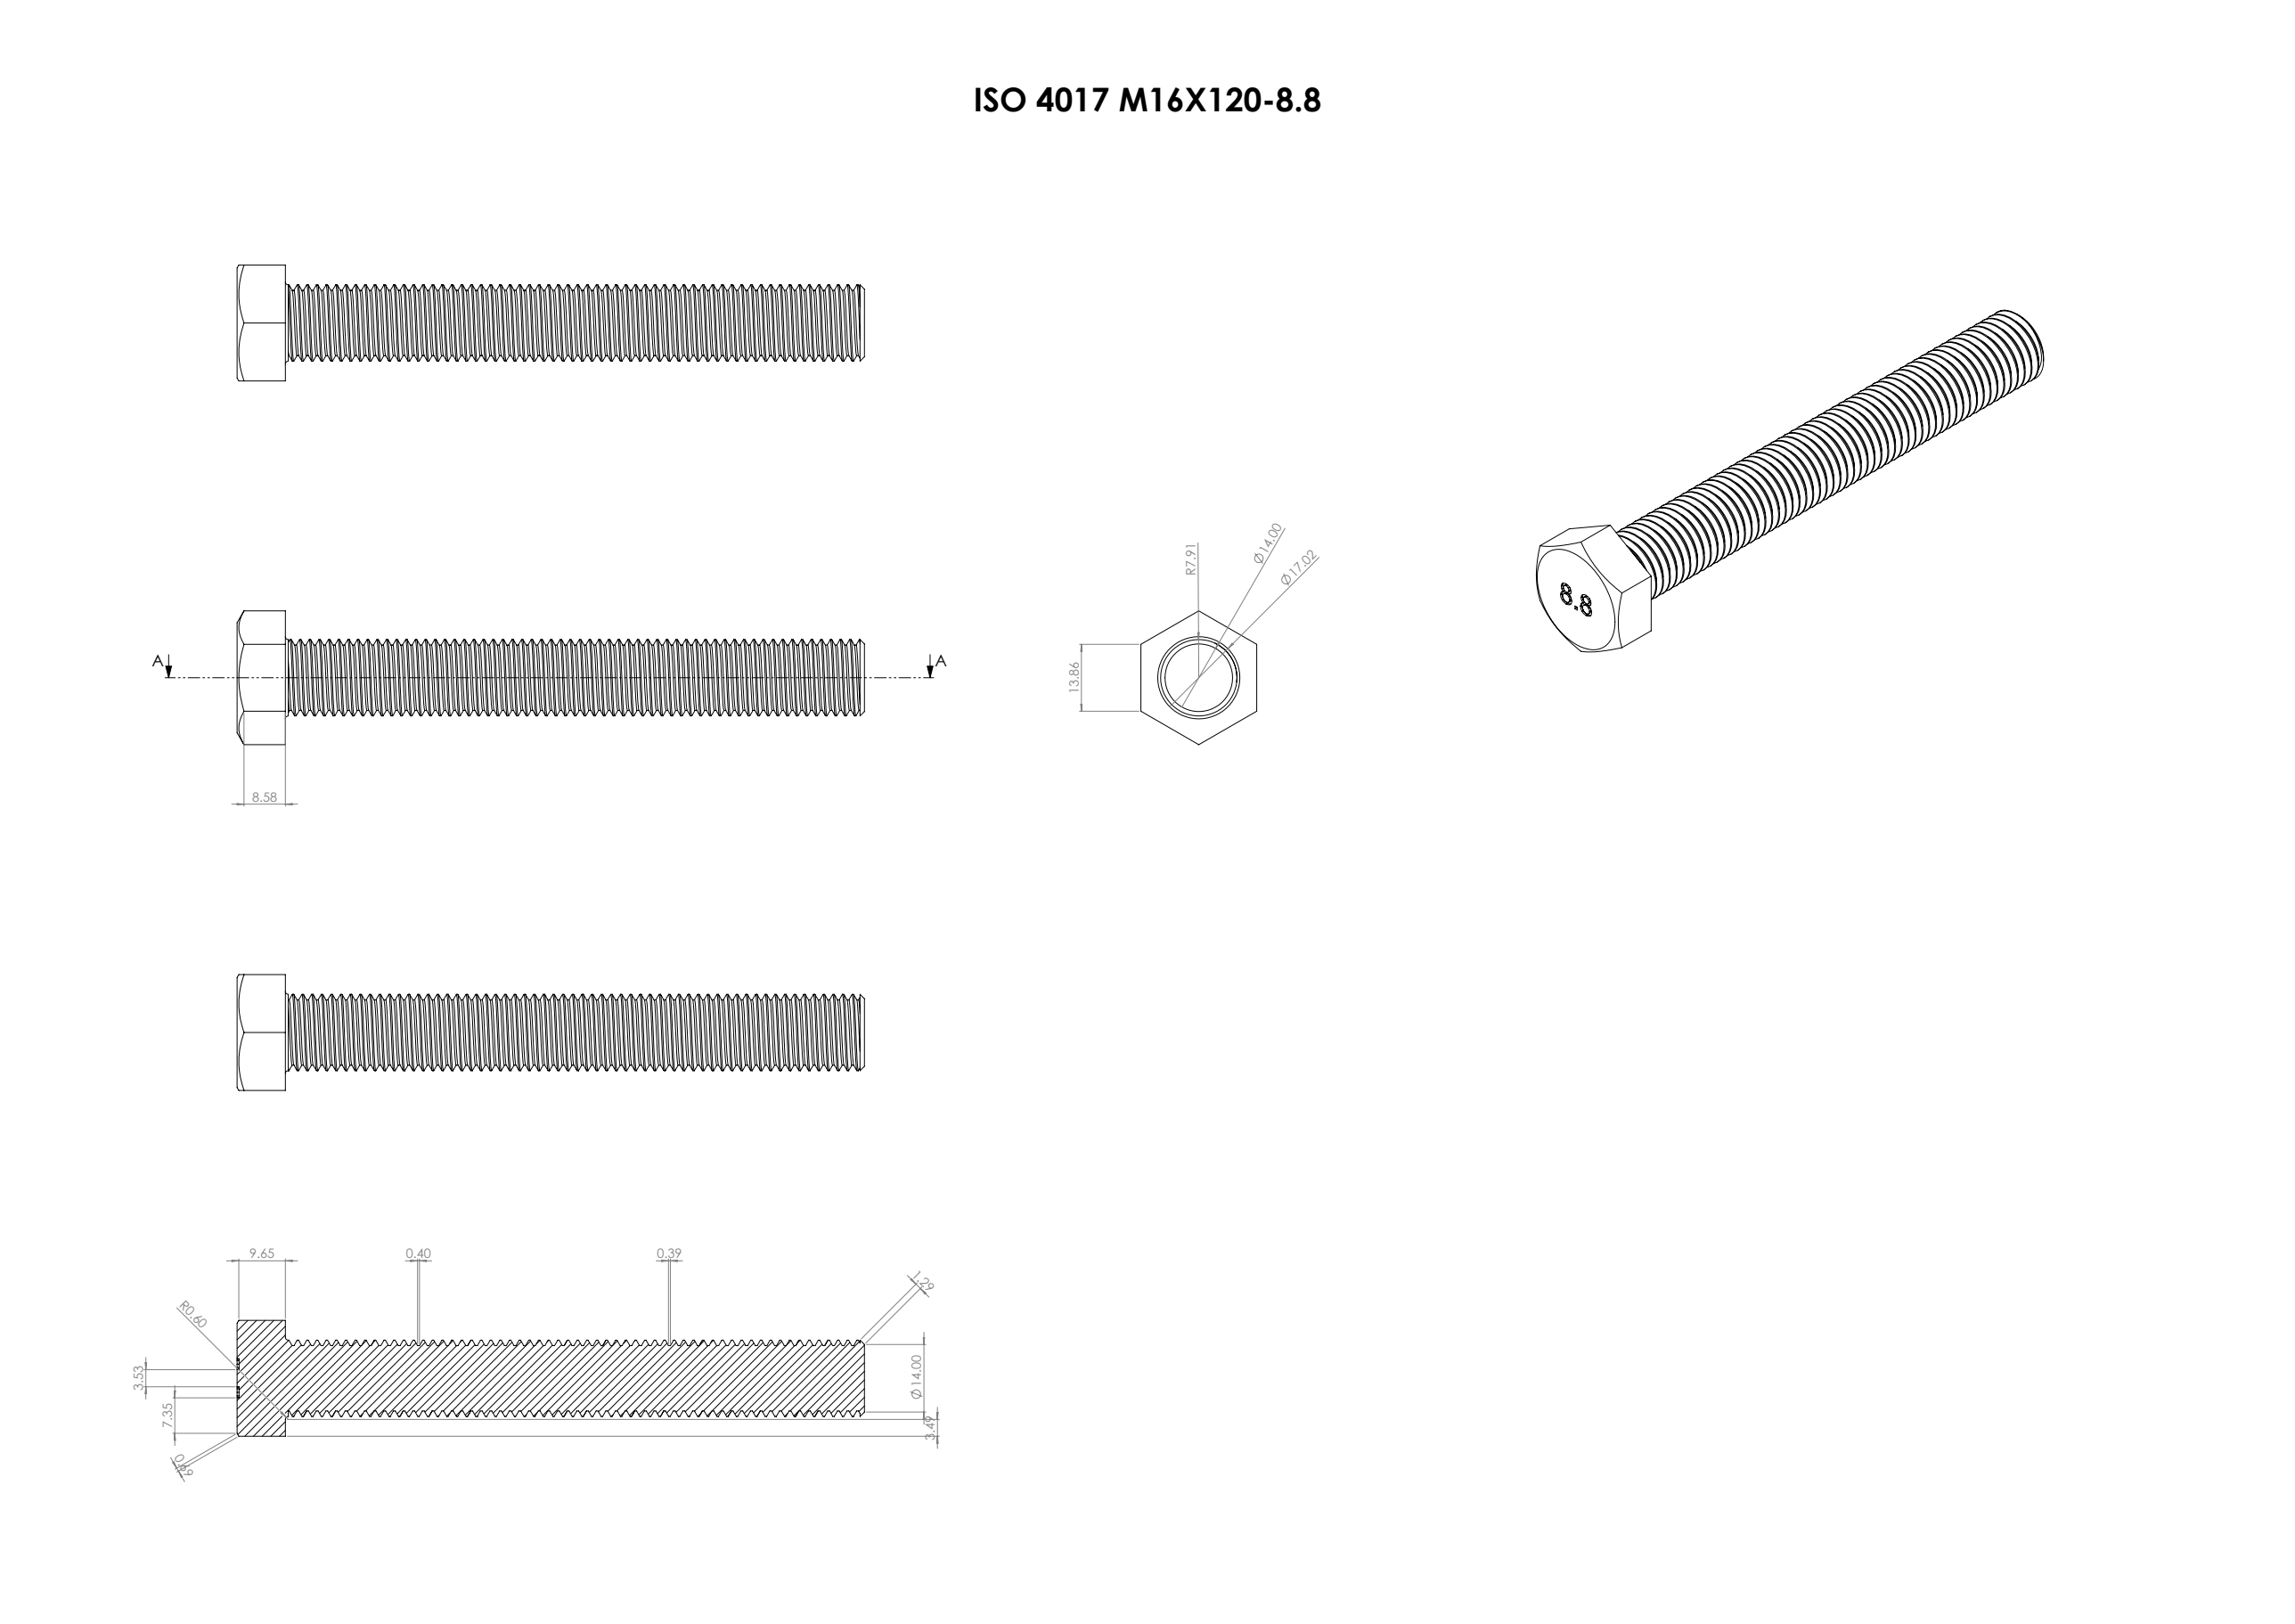
ISO-10303-21;
HEADER;
/* Generated by software containing ST-Developer
 * from STEP Tools, Inc. (www.steptools.com) 
 */

FILE_DESCRIPTION(
/* description */ (''),
/* implementation_level */ '2;1');

FILE_NAME(
/* name */ '17_ISO_4017_M16x120-8.8.step',
/* time_stamp */ '2026-10-20T10:03:03-07:00',
/* author */ (''),
/* organization */ (''),
/* preprocessor_version */ 'ST-DEVELOPER v20.2',
/* originating_system */ 'Autodesk Translation Framework v15.15.0.0',
/* authorisation */ '');

FILE_SCHEMA (('AUTOMOTIVE_DESIGN { 1 0 10303 214 3 1 1 }'));
ENDSEC;

DATA;
#10=MECHANICAL_DESIGN_GEOMETRIC_PRESENTATION_REPRESENTATION('',(#539),#71492);
#355=(
BOUNDED_CURVE()
B_SPLINE_CURVE(2,(#70524,#70525,#70526),.UNSPECIFIED.,.F.,.F.)
B_SPLINE_CURVE_WITH_KNOTS((3,3),(0.0830692064483412,1.5163968327409),
 .UNSPECIFIED.)
CURVE()
GEOMETRIC_REPRESENTATION_ITEM()
RATIONAL_B_SPLINE_CURVE((1.01933756729741,1.17702963774851,1.01933756729741))
REPRESENTATION_ITEM('')
);
#356=(
BOUNDED_CURVE()
B_SPLINE_CURVE(2,(#70528,#70529,#70530),.UNSPECIFIED.,.F.,.F.)
B_SPLINE_CURVE_WITH_KNOTS((3,3),(0.0830692064483407,1.5163968327409),
 .UNSPECIFIED.)
CURVE()
GEOMETRIC_REPRESENTATION_ITEM()
RATIONAL_B_SPLINE_CURVE((1.01933756729741,1.17702963774851,1.01933756729741))
REPRESENTATION_ITEM('')
);
#357=(
BOUNDED_CURVE()
B_SPLINE_CURVE(2,(#70532,#70533,#70534),.UNSPECIFIED.,.F.,.F.)
B_SPLINE_CURVE_WITH_KNOTS((3,3),(0.0830692064483414,1.5163968327409),
 .UNSPECIFIED.)
CURVE()
GEOMETRIC_REPRESENTATION_ITEM()
RATIONAL_B_SPLINE_CURVE((1.01933756729741,1.17702963774851,1.01933756729741))
REPRESENTATION_ITEM('')
);
#358=(
BOUNDED_CURVE()
B_SPLINE_CURVE(2,(#70536,#70537,#70538),.UNSPECIFIED.,.F.,.F.)
B_SPLINE_CURVE_WITH_KNOTS((3,3),(0.0830692064483412,1.5163968327409),
 .UNSPECIFIED.)
CURVE()
GEOMETRIC_REPRESENTATION_ITEM()
RATIONAL_B_SPLINE_CURVE((1.01933756729741,1.17702963774851,1.01933756729741))
REPRESENTATION_ITEM('')
);
#359=(
BOUNDED_CURVE()
B_SPLINE_CURVE(2,(#70540,#70541,#70542),.UNSPECIFIED.,.F.,.F.)
B_SPLINE_CURVE_WITH_KNOTS((3,3),(0.799733019594622,1.5163968327409),
 .UNSPECIFIED.)
CURVE()
GEOMETRIC_REPRESENTATION_ITEM()
RATIONAL_B_SPLINE_CURVE((1.09818360252296,1.09818360252296,1.01933756729741))
REPRESENTATION_ITEM('')
);
#360=(
BOUNDED_CURVE()
B_SPLINE_CURVE(2,(#70547,#70548,#70549),.UNSPECIFIED.,.F.,.F.)
B_SPLINE_CURVE_WITH_KNOTS((3,3),(0.083069206448341,0.799733019594622),
 .UNSPECIFIED.)
CURVE()
GEOMETRIC_REPRESENTATION_ITEM()
RATIONAL_B_SPLINE_CURVE((1.01933756729741,1.09818360252296,1.09818360252296))
REPRESENTATION_ITEM('')
);
#361=(
BOUNDED_CURVE()
B_SPLINE_CURVE(2,(#70550,#70551,#70552),.UNSPECIFIED.,.F.,.F.)
B_SPLINE_CURVE_WITH_KNOTS((3,3),(0.0830692064483408,1.5163968327409),
 .UNSPECIFIED.)
CURVE()
GEOMETRIC_REPRESENTATION_ITEM()
RATIONAL_B_SPLINE_CURVE((1.01933756729741,1.17702963774851,1.01933756729741))
REPRESENTATION_ITEM('')
);
#381=TOROIDAL_SURFACE('',#30426,0.8511,0.06);
#396=SHAPE_REPRESENTATION_RELATIONSHIP('SRR','None',#71617,#415);
#415=ADVANCED_BREP_SHAPE_REPRESENTATION('',(#434),#71487);
#434=MANIFOLD_SOLID_BREP('Bolt',#28473);
#539=STYLED_ITEM('',(#71894),#434);
#971=B_SPLINE_CURVE_WITH_KNOTS('',3,(#59083,#59084,#59085,#59086,#59087,
#59088,#59089,#59090,#59091,#59092),.UNSPECIFIED.,.F.,.F.,(4,3,3,4),(-4.0929304201308,
-3.25801350823594,-2.42309659634109,-2.07498647268397),.UNSPECIFIED.);
#972=B_SPLINE_CURVE_WITH_KNOTS('',3,(#59095,#59096,#59097,#59098,#59099,
#59100,#59101,#59102,#59103,#59104),.UNSPECIFIED.,.F.,.F.,(4,3,3,4),(0.,
0.499092211205179,0.998184422410358,1.12364870614423),.UNSPECIFIED.);
#973=B_SPLINE_CURVE_WITH_KNOTS('',3,(#59109,#59110,#59111,#59112,#59113,
#59114,#59115,#59116,#59117,#59118,#59119,#59120,#59121,#59122,#59123,#59124,
#59125,#59126,#59127,#59128,#59129,#59130,#59131,#59132,#59133,#59134,#59135,
#59136,#59137,#59138,#59139),.UNSPECIFIED.,.F.,.F.,(4,3,3,3,3,3,3,3,3,3,
4),(-10.3761157273104,-9.98184422410361,-8.98365980169324,-8.48456759048806,
-7.98547537928288,-6.98729095687252,-6.48819874566734,-5.98910653446216,
-5.49001432325698,-4.9909221120518,-4.0929304201308),.UNSPECIFIED.);
#974=B_SPLINE_CURVE_WITH_KNOTS('',3,(#59140,#59141,#59142,#59143,#59144,
#59145,#59146,#59147,#59148,#59149,#59150,#59151,#59152,#59153,#59154,#59155,
#59156,#59157,#59158,#59159,#59160,#59161,#59162,#59163,#59164,#59165,#59166,
#59167,#59168,#59169,#59170),.UNSPECIFIED.,.F.,.F.,(4,3,3,3,3,3,3,3,3,3,
4),(1.12364870614423,1.49727663361554,1.99636884482072,2.99455326723107,
3.99273768964143,4.99092211205179,5.49001432325697,5.98910653446215,6.48819874566733,
6.98729095687251,7.4068340133238),.UNSPECIFIED.);
#975=B_SPLINE_CURVE_WITH_KNOTS('',3,(#59175,#59176,#59177,#59178,#59179,
#59180,#59181,#59182,#59183,#59184,#59185,#59186,#59187,#59188,#59189,#59190,
#59191,#59192,#59193,#59194,#59195,#59196,#59197,#59198,#59199,#59200,#59201,
#59202,#59203,#59204,#59205),.UNSPECIFIED.,.F.,.F.,(4,3,3,3,3,3,3,3,3,3,
4),(-16.65930103449,-15.9709507585658,-15.4718585473606,-14.9727663361554,
-13.974581913745,-13.4754897025399,-12.9763974913347,-12.4773052801295,
-11.9782130689243,-10.980028646514,-10.3761157273104),.UNSPECIFIED.);
#976=B_SPLINE_CURVE_WITH_KNOTS('',3,(#59206,#59207,#59208,#59209,#59210,
#59211,#59212,#59213,#59214,#59215,#59216,#59217,#59218,#59219,#59220,#59221,
#59222,#59223,#59224,#59225,#59226,#59227,#59228,#59229,#59230),
 .UNSPECIFIED.,.F.,.F.,(4,3,3,3,3,3,3,3,4),(7.4068340133238,8.24175092521866,
9.07666783711352,9.91158474900838,10.7465016609032,11.5814185727981,12.416335484693,
13.2512523965878,13.6900193205034),.UNSPECIFIED.);
#977=B_SPLINE_CURVE_WITH_KNOTS('',3,(#59235,#59236,#59237,#59238,#59239,
#59240,#59241,#59242,#59243,#59244,#59245,#59246,#59247,#59248,#59249,#59250,
#59251,#59252,#59253,#59254,#59255,#59256,#59257,#59258,#59259,#59260,#59261,
#59262,#59263,#59264,#59265),.UNSPECIFIED.,.F.,.F.,(4,3,3,3,3,3,3,3,3,3,
4),(-22.9424863416695,-22.4591495042331,-21.9600572930279,-20.9618728706176,
-20.4627806594124,-19.9636884482072,-19.464596237002,-18.9655040257968,
-17.9673196033865,-16.9691351809761,-16.65930103449),.UNSPECIFIED.);
#978=B_SPLINE_CURVE_WITH_KNOTS('',3,(#59266,#59267,#59268,#59269,#59270,
#59271,#59272,#59273,#59274,#59275,#59276,#59277,#59278,#59279,#59280,#59281,
#59282,#59283,#59284,#59285,#59286,#59287,#59288,#59289,#59290),
 .UNSPECIFIED.,.F.,.F.,(4,3,3,3,3,3,3,3,4),(13.6900193205034,14.5249362323982,
15.3598531442931,16.1947700561879,17.0296869680828,17.8646038799776,18.6995207918725,
19.5344377037673,19.973204627683),.UNSPECIFIED.);
#979=B_SPLINE_CURVE_WITH_KNOTS('',3,(#59295,#59296,#59297,#59298,#59299,
#59300,#59301,#59302,#59303,#59304,#59305,#59306,#59307,#59308,#59309,#59310,
#59311,#59312,#59313,#59314,#59315,#59316,#59317,#59318,#59319,#59320,#59321,
#59322,#59323,#59324,#59325),.UNSPECIFIED.,.F.,.F.,(4,3,3,3,3,3,3,3,3,3,
4),(-29.2256716488491,-28.9473482499005,-27.9491638274901,-27.4500716162849,
-26.9509794050797,-26.4518871938745,-25.9527949826694,-24.954610560259,
-23.9564261378486,-22.9582417154383,-22.9424863416695),.UNSPECIFIED.);
#980=B_SPLINE_CURVE_WITH_KNOTS('',3,(#59326,#59327,#59328,#59329,#59330,
#59331,#59332,#59333,#59334,#59335,#59336,#59337,#59338,#59339,#59340,#59341,
#59342,#59343,#59344,#59345,#59346,#59347,#59348,#59349,#59350,#59351,#59352,
#59353),.UNSPECIFIED.,.F.,.F.,(4,3,3,3,3,3,3,3,3,4),(19.973204627683,20.4627806594124,
20.9618728706176,21.9600572930279,22.4591495042331,22.9582417154383,23.9564261378486,
24.954610560259,25.9527949826694,26.2563899348625),.UNSPECIFIED.);
#981=B_SPLINE_CURVE_WITH_KNOTS('',3,(#59358,#59359,#59360,#59361,#59362,
#59363,#59364,#59365,#59366,#59367,#59368,#59369,#59370,#59371,#59372,#59373,
#59374,#59375,#59376,#59377,#59378,#59379,#59380,#59381,#59382),
 .UNSPECIFIED.,.F.,.F.,(4,3,3,3,3,3,3,3,4),(-35.5088569560287,-34.6739400441339,
-33.839023132239,-33.0041062203442,-32.1691893084493,-31.3342723965544,
-30.4993554846596,-29.6644385727647,-29.2256716488491),.UNSPECIFIED.);
#982=B_SPLINE_CURVE_WITH_KNOTS('',3,(#59383,#59384,#59385,#59386,#59387,
#59388,#59389,#59390,#59391,#59392,#59393,#59394,#59395,#59396,#59397,#59398,
#59399,#59400,#59401,#59402,#59403,#59404,#59405,#59406,#59407,#59408,#59409,
#59410,#59411,#59412,#59413),.UNSPECIFIED.,.F.,.F.,(4,3,3,3,3,3,3,3,3,3,
4),(26.2563899348625,26.4518871938745,26.9509794050797,27.4500716162849,
27.9491638274901,28.9473482499005,29.4464404611057,29.9455326723108,30.9437170947212,
31.9419015171316,32.5395752420422),.UNSPECIFIED.);
#983=B_SPLINE_CURVE_WITH_KNOTS('',3,(#59418,#59419,#59420,#59421,#59422,
#59423,#59424,#59425,#59426,#59427,#59428,#59429,#59430,#59431,#59432,#59433,
#59434,#59435,#59436,#59437,#59438,#59439,#59440,#59441,#59442),
 .UNSPECIFIED.,.F.,.F.,(4,3,3,3,3,3,3,3,4),(-41.7920422632083,-40.9571253513134,
-40.1222084394186,-39.2872915275237,-38.4523746156289,-37.617457703734,
-36.7825407918392,-35.9476238799443,-35.5088569560287),.UNSPECIFIED.);
#984=B_SPLINE_CURVE_WITH_KNOTS('',3,(#59443,#59444,#59445,#59446,#59447,
#59448,#59449,#59450,#59451,#59452,#59453,#59454,#59455,#59456,#59457,#59458,
#59459,#59460,#59461,#59462,#59463,#59464,#59465,#59466,#59467,#59468,#59469,
#59470,#59471,#59472,#59473),.UNSPECIFIED.,.F.,.F.,(4,3,3,3,3,3,3,3,3,3,
4),(32.5395752420422,32.940085939542,33.4391781507471,33.9382703619523,
34.4373625731575,34.9364547843627,35.934639206773,36.4337314179782,36.9328236291834,
37.9310080515937,38.8227605492217),.UNSPECIFIED.);
#985=B_SPLINE_CURVE_WITH_KNOTS('',3,(#59478,#59479,#59480,#59481,#59482,
#59483,#59484,#59485,#59486,#59487,#59488,#59489,#59490,#59491,#59492,#59493,
#59494,#59495,#59496,#59497,#59498,#59499,#59500,#59501,#59502),
 .UNSPECIFIED.,.F.,.F.,(4,3,3,3,3,3,3,3,4),(-48.0752275703879,-47.240310658493,
-46.4053937465982,-45.5704768347033,-44.7355599228084,-43.9006430109136,
-43.0657260990187,-42.2308091871238,-41.7920422632083),.UNSPECIFIED.);
#986=B_SPLINE_CURVE_WITH_KNOTS('',3,(#59503,#59504,#59505,#59506,#59507,
#59508,#59509,#59510,#59511,#59512,#59513,#59514,#59515,#59516,#59517,#59518,
#59519,#59520,#59521,#59522,#59523,#59524,#59525,#59526,#59527,#59528,#59529,
#59530,#59531,#59532,#59533,#59534,#59535,#59536),.UNSPECIFIED.,.F.,.F.,
(4,3,3,3,3,3,3,3,3,3,3,4),(38.8227605492217,38.929192474004,39.9273768964144,
40.4264691076196,40.9255613188247,41.4246535300299,41.9237457412351,42.9219301636455,
43.4210223748506,43.9201145860558,44.9182990084662,45.1059458564013),
 .UNSPECIFIED.);
#987=B_SPLINE_CURVE_WITH_KNOTS('',3,(#59541,#59542,#59543,#59544,#59545,
#59546,#59547,#59548,#59549,#59550,#59551,#59552,#59553,#59554,#59555,#59556,
#59557,#59558,#59559,#59560,#59561,#59562,#59563,#59564,#59565),
 .UNSPECIFIED.,.F.,.F.,(4,3,3,3,3,3,3,3,4),(-54.3584128775675,-53.5234959656726,
-52.6885790537778,-51.8536621418829,-51.018745229988,-50.1838283180932,
-49.3489114061983,-48.5139944943034,-48.0752275703879),.UNSPECIFIED.);
#988=B_SPLINE_CURVE_WITH_KNOTS('',3,(#59566,#59567,#59568,#59569,#59570,
#59571,#59572,#59573,#59574,#59575,#59576,#59577,#59578,#59579,#59580,#59581,
#59582,#59583,#59584,#59585,#59586,#59587,#59588,#59589,#59590,#59591,#59592,
#59593,#59594,#59595,#59596),.UNSPECIFIED.,.F.,.F.,(4,3,3,3,3,3,3,3,3,3,
4),(45.1059458564013,45.9164834308765,46.9146678532869,47.4137600644921,
47.9128522756973,48.4119444869025,48.9110366981077,49.909221120518,50.4083133317232,
50.9074055429284,51.3891311635809),.UNSPECIFIED.);
#989=B_SPLINE_CURVE_WITH_KNOTS('',3,(#59601,#59602,#59603,#59604,#59605,
#59606,#59607,#59608,#59609,#59610,#59611,#59612,#59613,#59614,#59615,#59616,
#59617,#59618,#59619,#59620,#59621,#59622,#59623,#59624,#59625,#59626,#59627,
#59628,#59629,#59630,#59631),.UNSPECIFIED.,.F.,.F.,(4,3,3,3,3,3,3,3,3,3,
4),(-60.6415981847471,-59.8910653446216,-58.8928809222113,-57.8946964998009,
-57.3956042885957,-56.8965120773905,-55.8983276549802,-55.399235443775,
-54.9001432325698,-54.4010510213646,-54.3584128775675),.UNSPECIFIED.);
#990=B_SPLINE_CURVE_WITH_KNOTS('',3,(#59632,#59633,#59634,#59635,#59636,
#59637,#59638,#59639,#59640,#59641,#59642,#59643,#59644,#59645,#59646,#59647,
#59648,#59649,#59650,#59651,#59652,#59653,#59654,#59655,#59656,#59657,#59658,
#59659,#59660,#59661,#59662),.UNSPECIFIED.,.F.,.F.,(4,3,3,3,3,3,3,3,3,3,
4),(51.3891311635809,51.9055899653388,52.9037743877492,53.9019588101595,
54.4010510213647,54.9001432325699,55.3992354437751,55.8983276549802,56.8965120773906,
57.3956042885958,57.6723164707605),.UNSPECIFIED.);
#991=B_SPLINE_CURVE_WITH_KNOTS('',3,(#59667,#59668,#59669,#59670,#59671,
#59672,#59673,#59674,#59675,#59676,#59677,#59678,#59679,#59680,#59681,#59682,
#59683,#59684,#59685,#59686,#59687,#59688,#59689,#59690,#59691,#59692,#59693,
#59694,#59695,#59696,#59697,#59698,#59699,#59700),.UNSPECIFIED.,.F.,.F.,
(4,3,3,3,3,3,3,3,3,3,3,4),(-66.9247834919267,-66.8783563014941,-65.8801718790838,
-64.8819874566734,-64.3828952454682,-63.8838030342631,-62.8856186118527,
-62.3865264006475,-61.8874341894423,-61.3883419782372,-60.889249767032,
-60.6415981847471),.UNSPECIFIED.);
#992=B_SPLINE_CURVE_WITH_KNOTS('',3,(#59701,#59702,#59703,#59704,#59705,
#59706,#59707,#59708,#59709,#59710,#59711,#59712,#59713,#59714,#59715,#59716,
#59717,#59718,#59719,#59720,#59721,#59722,#59723,#59724,#59725,#59726,#59727,
#59728,#59729,#59730,#59731),.UNSPECIFIED.,.F.,.F.,(4,3,3,3,3,3,3,3,3,3,
4),(57.6723164707605,57.894696499801,58.8928809222113,59.8910653446217,
60.8892497670321,61.3883419782372,61.8874341894424,62.3865264006476,62.8856186118528,
63.8838030342631,63.9555017779401),.UNSPECIFIED.);
#993=B_SPLINE_CURVE_WITH_KNOTS('',3,(#59736,#59737,#59738,#59739,#59740,
#59741,#59742,#59743,#59744,#59745,#59746,#59747,#59748,#59749,#59750,#59751,
#59752,#59753,#59754,#59755,#59756,#59757,#59758,#59759,#59760,#59761,#59762,
#59763,#59764,#59765,#59766),.UNSPECIFIED.,.F.,.F.,(4,3,3,3,3,3,3,3,3,3,
4),(-73.2079687991063,-72.8674628359563,-71.869278413546,-71.3701862023408,
-70.8710939911356,-69.8729095687252,-69.37381735752,-68.8747251463149,-68.3756329351097,
-67.8765407239045,-66.9247834919267),.UNSPECIFIED.);
#994=B_SPLINE_CURVE_WITH_KNOTS('',3,(#59767,#59768,#59769,#59770,#59771,
#59772,#59773,#59774,#59775,#59776,#59777,#59778,#59779,#59780,#59781,#59782,
#59783,#59784,#59785,#59786,#59787,#59788,#59789,#59790,#59791,#59792,#59793,
#59794,#59795,#59796,#59797),.UNSPECIFIED.,.F.,.F.,(4,3,3,3,3,3,3,3,3,3,
4),(63.9555017779401,64.3828952454683,64.8819874566735,65.8801718790838,
66.8783563014942,67.8765407239045,68.3756329351097,68.8747251463149,69.37381735752,
69.8729095687252,70.2386870851197),.UNSPECIFIED.);
#995=B_SPLINE_CURVE_WITH_KNOTS('',3,(#59802,#59803,#59804,#59805,#59806,
#59807,#59808,#59809,#59810,#59811,#59812,#59813,#59814,#59815,#59816,#59817,
#59818,#59819,#59820,#59821,#59822,#59823,#59824,#59825,#59826,#59827,#59828,
#59829,#59830,#59831,#59832),.UNSPECIFIED.,.F.,.F.,(4,3,3,3,3,3,3,3,3,3,
4),(-79.4911541062859,-78.8565693704185,-78.3574771592133,-77.8583849480081,
-76.8602005255977,-76.3611083143926,-75.8620161031874,-75.3629238919822,
-74.863831680777,-73.8656472583666,-73.2079687991063),.UNSPECIFIED.);
#996=B_SPLINE_CURVE_WITH_KNOTS('',3,(#59833,#59834,#59835,#59836,#59837,
#59838,#59839,#59840,#59841,#59842,#59843,#59844,#59845,#59846,#59847,#59848,
#59849,#59850,#59851,#59852,#59853,#59854,#59855,#59856,#59857),
 .UNSPECIFIED.,.F.,.F.,(4,3,3,3,3,3,3,3,4),(70.2386870851197,71.0736039970146,
71.9085209089095,72.7434378208043,73.5783547326992,74.413271644594,75.2481885564889,
76.0831054683838,76.5218723922993),.UNSPECIFIED.);
#997=B_SPLINE_CURVE_WITH_KNOTS('',3,(#59862,#59863,#59864,#59865,#59866,
#59867,#59868,#59869,#59870,#59871,#59872,#59873,#59874,#59875,#59876,#59877,
#59878,#59879,#59880,#59881,#59882,#59883,#59884,#59885,#59886,#59887,#59888,
#59889,#59890,#59891,#59892),.UNSPECIFIED.,.F.,.F.,(4,3,3,3,3,3,3,3,3,3,
4),(-85.7743394134655,-85.3447681160858,-84.8456759048806,-83.8474914824703,
-83.3483992712651,-82.8493070600599,-82.3502148488547,-81.8511226376495,
-80.8529382152392,-79.8547537928288,-79.4911541062859),.UNSPECIFIED.);
#998=B_SPLINE_CURVE_WITH_KNOTS('',3,(#59893,#59894,#59895,#59896,#59897,
#59898,#59899,#59900,#59901,#59902,#59903,#59904,#59905,#59906,#59907,#59908,
#59909,#59910,#59911,#59912,#59913,#59914,#59915,#59916,#59917,#59918,#59919,
#59920),.UNSPECIFIED.,.F.,.F.,(4,3,3,3,3,3,3,3,3,4),(76.5218723922993,76.8602005255978,
77.8583849480082,78.3574771592134,78.8565693704185,79.8547537928289,80.8529382152392,
81.8511226376496,82.3502148488548,82.8050576994789),.UNSPECIFIED.);
#999=B_SPLINE_CURVE_WITH_KNOTS('',3,(#59925,#59926,#59927,#59928,#59929,
#59930,#59931,#59932,#59933,#59934,#59935,#59936,#59937,#59938,#59939,#59940,
#59941,#59942,#59943,#59944,#59945,#59946,#59947,#59948,#59949,#59950,#59951,
#59952,#59953,#59954,#59955),.UNSPECIFIED.,.F.,.F.,(4,3,3,3,3,3,3,3,3,3,
4),(-92.057524720645,-91.8329668617531,-90.8347824393428,-90.3356902281376,
-89.8365980169324,-89.3375058057272,-88.8384135945221,-87.8402291721117,
-86.8420447497013,-85.843860327291,-85.7743394134655),.UNSPECIFIED.);
#1000=B_SPLINE_CURVE_WITH_KNOTS('',3,(#59956,#59957,#59958,#59959,#59960,
#59961,#59962,#59963,#59964,#59965,#59966,#59967,#59968,#59969,#59970,#59971,
#59972,#59973,#59974,#59975,#59976,#59977,#59978,#59979,#59980,#59981,#59982,
#59983,#59984,#59985,#59986),.UNSPECIFIED.,.F.,.F.,(4,3,3,3,3,3,3,3,3,3,
4),(82.8050576994789,82.84930706006,83.3483992712651,83.8474914824703,84.8456759048807,
85.3447681160858,85.843860327291,86.8420447497014,87.8402291721117,88.8384135945221,
89.0882430066585),.UNSPECIFIED.);
#1001=B_SPLINE_CURVE_WITH_KNOTS('',3,(#59991,#59992,#59993,#59994,#59995,
#59996,#59997,#59998,#59999,#60000,#60001,#60002,#60003,#60004,#60005,#60006,
#60007,#60008,#60009,#60010,#60011,#60012,#60013,#60014,#60015),
 .UNSPECIFIED.,.F.,.F.,(4,3,3,3,3,3,3,3,4),(-98.3407100278246,-97.5057931159298,
-96.6708762040349,-95.8359592921401,-95.0010423802452,-94.1661254683504,
-93.3312085564555,-92.4962916445607,-92.057524720645),.UNSPECIFIED.);
#1002=B_SPLINE_CURVE_WITH_KNOTS('',3,(#60016,#60017,#60018,#60019,#60020,
#60021,#60022,#60023,#60024,#60025,#60026,#60027,#60028,#60029,#60030,#60031,
#60032,#60033,#60034,#60035,#60036,#60037,#60038,#60039,#60040,#60041,#60042,
#60043,#60044,#60045,#60046),.UNSPECIFIED.,.F.,.F.,(4,3,3,3,3,3,3,3,3,3,
4),(89.0882430066585,89.3375058057273,89.8365980169325,90.3356902281376,
90.8347824393428,91.8329668617532,92.3320590729584,92.8311512841636,93.8293357065739,
94.8275201289843,95.3714283138381),.UNSPECIFIED.);
#1003=B_SPLINE_CURVE_WITH_KNOTS('',3,(#60051,#60052,#60053,#60054,#60055,
#60056,#60057,#60058,#60059,#60060,#60061,#60062,#60063,#60064,#60065,#60066,
#60067,#60068,#60069,#60070,#60071,#60072,#60073,#60074,#60075),
 .UNSPECIFIED.,.F.,.F.,(4,3,3,3,3,3,3,3,4),(-104.623895335004,-103.788978423109,
-102.954061511215,-102.11914459932,-101.284227687425,-100.44931077553,-99.6143938636351,
-98.7794769517402,-98.3407100278246),.UNSPECIFIED.);
#1004=B_SPLINE_CURVE_WITH_KNOTS('',3,(#60076,#60077,#60078,#60079,#60080,
#60081,#60082,#60083,#60084,#60085,#60086,#60087,#60088,#60089,#60090,#60091,
#60092,#60093,#60094,#60095,#60096,#60097,#60098,#60099,#60100),
 .UNSPECIFIED.,.F.,.F.,(4,3,3,3,3,3,3,3,4),(95.3714283138381,96.206345225733,
97.0412621376278,97.8761790495227,98.7110959614176,99.5460128733125,100.380929785207,
101.215846697102,101.654613621018),.UNSPECIFIED.);
#1005=B_SPLINE_CURVE_WITH_KNOTS('',3,(#60105,#60106,#60107,#60108,#60109,
#60110,#60111,#60112,#60113,#60114,#60115,#60116,#60117,#60118,#60119,#60120,
#60121,#60122,#60123,#60124,#60125,#60126,#60127,#60128,#60129),
 .UNSPECIFIED.,.F.,.F.,(4,3,3,3,3,3,3,3,4),(-110.907080642184,-110.072163730289,
-109.237246818394,-108.402329906499,-107.567412994604,-106.73249608271,
-105.897579170815,-105.06266225892,-104.623895335004),.UNSPECIFIED.);
#1006=B_SPLINE_CURVE_WITH_KNOTS('',3,(#60130,#60131,#60132,#60133,#60134,
#60135,#60136,#60137,#60138,#60139,#60140,#60141,#60142,#60143,#60144,#60145,
#60146,#60147,#60148,#60149,#60150,#60151,#60152,#60153,#60154),
 .UNSPECIFIED.,.F.,.F.,(4,3,3,3,3,3,3,3,4),(101.654613621018,102.489530532913,
103.324447444807,104.159364356702,104.994281268597,105.829198180492,106.664115092387,
107.499032004282,107.937798928197),.UNSPECIFIED.);
#1007=B_SPLINE_CURVE_WITH_KNOTS('',3,(#60159,#60160,#60161,#60162,#60163,
#60164,#60165,#60166,#60167,#60168,#60169,#60170,#60171,#60172,#60173,#60174,
#60175,#60176,#60177,#60178,#60179,#60180,#60181,#60182,#60183),
 .UNSPECIFIED.,.F.,.F.,(4,3,3,3,3,3,3,3,4),(-117.190265949363,-116.355349037469,
-115.520432125574,-114.685515213679,-113.850598301784,-113.015681389889,
-112.180764477994,-111.345847566099,-110.907080642184),.UNSPECIFIED.);
#1008=B_SPLINE_CURVE_WITH_KNOTS('',3,(#60184,#60185,#60186,#60187,#60188,
#60189,#60190,#60191,#60192,#60193,#60194,#60195,#60196,#60197,#60198,#60199,
#60200,#60201,#60202,#60203,#60204,#60205,#60206,#60207,#60208,#60209,#60210,
#60211,#60212,#60213,#60214),.UNSPECIFIED.,.F.,.F.,(4,3,3,3,3,3,3,3,3,3,
4),(107.937798928197,108.802102042729,109.80028646514,110.299378676345,
110.79847088755,111.297563098755,111.79665530996,112.794839732371,113.293931943576,
113.793024154781,114.220984235377),.UNSPECIFIED.);
#1009=B_SPLINE_CURVE_WITH_KNOTS('',3,(#60219,#60220,#60221,#60222,#60223,
#60224,#60225,#60226,#60227,#60228,#60229,#60230,#60231,#60232,#60233,#60234,
#60235,#60236,#60237,#60238,#60239,#60240,#60241,#60242,#60243,#60244,#60245,
#60246,#60247,#60248,#60249),.UNSPECIFIED.,.F.,.F.,(4,3,3,3,3,3,3,3,3,3,
4),(-123.473451256543,-122.776683956474,-121.778499534064,-120.780315111654,
-120.281222900448,-119.782130689243,-118.783946266833,-118.284854055628,
-117.785761844422,-117.286669633217,-117.190265949363),.UNSPECIFIED.);
#1010=B_SPLINE_CURVE_WITH_KNOTS('',3,(#60250,#60251,#60252,#60253,#60254,
#60255,#60256,#60257,#60258,#60259,#60260,#60261,#60262,#60263,#60264,#60265,
#60266,#60267,#60268,#60269,#60270,#60271,#60272,#60273,#60274,#60275,#60276,
#60277,#60278,#60279,#60280),.UNSPECIFIED.,.F.,.F.,(4,3,3,3,3,3,3,3,3,3,
4),(114.220984235377,114.791208577191,115.789392999602,116.787577422012,
117.286669633217,117.785761844423,118.284854055628,118.783946266833,119.782130689243,
120.281222900448,120.504169542556),.UNSPECIFIED.);
#1011=B_SPLINE_CURVE_WITH_KNOTS('',3,(#60285,#60286,#60287,#60288,#60289,
#60290,#60291,#60292,#60293,#60294,#60295,#60296,#60297,#60298,#60299,#60300,
#60301,#60302,#60303,#60304,#60305,#60306,#60307,#60308,#60309,#60310,#60311,
#60312,#60313,#60314,#60315),.UNSPECIFIED.,.F.,.F.,(4,3,3,3,3,3,3,3,3,3,
4),(-129.756636563723,-128.765790490936,-127.767606068526,-127.268513857321,
-126.769421646116,-125.771237223705,-125.2721450125,-124.773052801295,-124.27396059009,
-123.774868378885,-123.473451256543),.UNSPECIFIED.);
#1012=B_SPLINE_CURVE_WITH_KNOTS('',3,(#60316,#60317,#60318,#60319,#60320,
#60321,#60322,#60323,#60324,#60325,#60326,#60327,#60328,#60329,#60330,#60331,
#60332,#60333,#60334,#60335,#60336,#60337,#60338,#60339,#60340,#60341,#60342,
#60343,#60344,#60345,#60346),.UNSPECIFIED.,.F.,.F.,(4,3,3,3,3,3,3,3,3,3,
4),(120.504169542556,120.780315111654,121.778499534064,122.776683956474,
123.774868378885,124.27396059009,124.773052801295,125.2721450125,125.771237223705,
126.769421646116,126.787354849736),.UNSPECIFIED.);
#1013=B_SPLINE_CURVE_WITH_KNOTS('',3,(#60351,#60352,#60353,#60354,#60355,
#60356,#60357,#60358,#60359,#60360,#60361,#60362,#60363,#60364,#60365,#60366,
#60367,#60368,#60369,#60370,#60371,#60372,#60373,#60374,#60375,#60376,#60377,
#60378,#60379,#60380,#60381,#60382,#60383,#60384),.UNSPECIFIED.,.F.,.F.,
(4,3,3,3,3,3,3,3,3,3,3,4),(-136.039821870902,-135.753081447809,-134.754897025399,
-134.255804814193,-133.756712602988,-132.758528180578,-132.259435969373,
-131.760343758168,-131.261251546962,-130.762159335757,-129.763974913347,
-129.756636563723),.UNSPECIFIED.);
#1014=B_SPLINE_CURVE_WITH_KNOTS('',3,(#60385,#60386,#60387,#60388,#60389,
#60390,#60391,#60392,#60393,#60394,#60395,#60396,#60397,#60398,#60399,#60400,
#60401,#60402,#60403,#60404,#60405,#60406,#60407,#60408,#60409,#60410,#60411,
#60412,#60413,#60414,#60415),.UNSPECIFIED.,.F.,.F.,(4,3,3,3,3,3,3,3,3,3,
4),(126.787354849736,127.268513857321,127.767606068526,128.765790490936,
129.763974913347,130.762159335757,131.261251546962,131.760343758168,132.259435969373,
132.758528180578,133.070540156916),.UNSPECIFIED.);
#1015=B_SPLINE_CURVE_WITH_KNOTS('',3,(#60420,#60421,#60422,#60423,#60424,
#60425,#60426,#60427,#60428,#60429,#60430,#60431,#60432,#60433,#60434,#60435,
#60436,#60437,#60438,#60439,#60440,#60441,#60442,#60443,#60444,#60445,#60446,
#60447,#60448,#60449,#60450),.UNSPECIFIED.,.F.,.F.,(4,3,3,3,3,3,3,3,3,3,
4),(-142.323007178082,-141.742187982271,-141.243095771066,-140.744003559861,
-139.74581913745,-139.246726926245,-138.74763471504,-138.248542503835,-137.74945029263,
-136.751265870219,-136.039821870902),.UNSPECIFIED.);
#1016=B_SPLINE_CURVE_WITH_KNOTS('',3,(#60451,#60452,#60453,#60454,#60455,
#60456,#60457,#60458,#60459,#60460,#60461,#60462,#60463,#60464,#60465,#60466,
#60467,#60468,#60469,#60470,#60471,#60472,#60473,#60474,#60475),
 .UNSPECIFIED.,.F.,.F.,(4,3,3,3,3,3,3,3,4),(133.070540156916,133.905457068811,
134.740373980705,135.5752908926,136.410207804495,137.24512471639,138.080041628285,
138.91495854018,139.353725464095),.UNSPECIFIED.);
#1017=B_SPLINE_CURVE_WITH_KNOTS('',3,(#60480,#60481,#60482,#60483,#60484,
#60485,#60486,#60487,#60488,#60489,#60490,#60491,#60492,#60493,#60494,#60495,
#60496,#60497,#60498,#60499,#60500,#60501,#60502,#60503,#60504,#60505,#60506,
#60507,#60508,#60509,#60510),.UNSPECIFIED.,.F.,.F.,(4,3,3,3,3,3,3,3,3,3,
4),(-148.606192485261,-148.230386727938,-147.731294516733,-146.733110094323,
-146.234017883118,-145.734925671913,-145.235833460707,-144.736741249502,
-143.738556827092,-142.740372404682,-142.323007178082),.UNSPECIFIED.);
#1018=B_SPLINE_CURVE_WITH_KNOTS('',3,(#60511,#60512,#60513,#60514,#60515,
#60516,#60517,#60518,#60519,#60520,#60521,#60522,#60523,#60524,#60525,#60526,
#60527,#60528,#60529,#60530,#60531,#60532,#60533,#60534,#60535,#60536,#60537,
#60538),.UNSPECIFIED.,.F.,.F.,(4,3,3,3,3,3,3,3,3,4),(139.353725464095,139.74581913745,
140.744003559861,141.243095771066,141.742187982271,142.740372404682,143.738556827092,
144.736741249502,145.235833460707,145.636910771275),.UNSPECIFIED.);
#1019=B_SPLINE_CURVE_WITH_KNOTS('',3,(#60543,#60544,#60545,#60546,#60547,
#60548,#60549,#60550,#60551,#60552,#60553,#60554,#60555,#60556,#60557,#60558,
#60559,#60560,#60561,#60562,#60563,#60564,#60565,#60566,#60567,#60568,#60569,
#60570,#60571,#60572,#60573),.UNSPECIFIED.,.F.,.F.,(4,3,3,3,3,3,3,3,3,3,
4),(-154.889377792441,-154.718585473606,-153.720401051195,-153.22130883999,
-152.722216628785,-152.22312441758,-151.724032206375,-150.725847783964,
-149.727663361554,-148.729478939144,-148.606192485261),.UNSPECIFIED.);
#1020=B_SPLINE_CURVE_WITH_KNOTS('',3,(#60574,#60575,#60576,#60577,#60578,
#60579,#60580,#60581,#60582,#60583,#60584,#60585,#60586,#60587,#60588,#60589,
#60590,#60591,#60592,#60593,#60594,#60595,#60596,#60597,#60598,#60599,#60600,
#60601,#60602,#60603,#60604),.UNSPECIFIED.,.F.,.F.,(4,3,3,3,3,3,3,3,3,3,
4),(145.636910771275,145.734925671913,146.234017883118,146.733110094323,
147.731294516733,148.230386727939,148.729478939144,149.727663361554,150.725847783964,
151.724032206375,151.920096078454),.UNSPECIFIED.);
#1021=B_SPLINE_CURVE_WITH_KNOTS('',3,(#60609,#60610,#60611,#60612,#60613,
#60614,#60615,#60616,#60617,#60618,#60619,#60620,#60621,#60622,#60623,#60624,
#60625,#60626,#60627,#60628,#60629,#60630,#60631,#60632,#60633,#60634,#60635,
#60636,#60637,#60638,#60639),.UNSPECIFIED.,.F.,.F.,(4,3,3,3,3,3,3,3,3,3,
4),(-161.17256309962,-160.707692008068,-160.208599796863,-159.709507585658,
-159.210415374452,-158.711323163247,-157.713138740837,-156.714954318427,
-155.716769896016,-155.217677684811,-154.889377792441),.UNSPECIFIED.);
#1022=B_SPLINE_CURVE_WITH_KNOTS('',3,(#60640,#60641,#60642,#60643,#60644,
#60645,#60646,#60647,#60648,#60649,#60650,#60651,#60652,#60653,#60654,#60655,
#60656,#60657,#60658,#60659,#60660,#60661,#60662,#60663,#60664,#60665,#60666,
#60667,#60668,#60669,#60670),.UNSPECIFIED.,.F.,.F.,(4,3,3,3,3,3,3,3,3,3,
4),(151.920096078454,152.22312441758,152.722216628785,153.22130883999,153.720401051196,
154.718585473606,155.217677684811,155.716769896016,156.714954318427,157.713138740837,
158.203281385634),.UNSPECIFIED.);
#1023=B_SPLINE_CURVE_WITH_KNOTS('',3,(#60675,#60676,#60677,#60678,#60679,
#60680,#60681,#60682,#60683,#60684,#60685,#60686,#60687,#60688,#60689,#60690,
#60691,#60692,#60693,#60694,#60695,#60696,#60697,#60698,#60699),
 .UNSPECIFIED.,.F.,.F.,(4,3,3,3,3,3,3,3,4),(-167.4557484068,-166.620831494905,
-165.78591458301,-164.950997671115,-164.116080759221,-163.281163847326,
-162.446246935431,-161.611330023536,-161.17256309962),.UNSPECIFIED.);
#1024=B_SPLINE_CURVE_WITH_KNOTS('',3,(#60700,#60701,#60702,#60703,#60704,
#60705,#60706,#60707,#60708,#60709,#60710,#60711,#60712,#60713,#60714,#60715,
#60716,#60717,#60718,#60719,#60720,#60721,#60722,#60723,#60724),
 .UNSPECIFIED.,.F.,.F.,(4,3,3,3,3,3,3,3,4),(158.203281385634,159.038198297529,
159.873115209424,160.708032121319,161.542949033213,162.377865945108,163.212782857003,
164.047699768898,164.486466692813),.UNSPECIFIED.);
#1025=B_SPLINE_CURVE_WITH_KNOTS('',3,(#60729,#60730,#60731,#60732,#60733,
#60734,#60735,#60736,#60737,#60738,#60739,#60740,#60741,#60742,#60743,#60744,
#60745,#60746,#60747,#60748,#60749,#60750,#60751,#60752,#60753),
 .UNSPECIFIED.,.F.,.F.,(4,3,3,3,3,3,3,3,4),(-173.73893371398,-172.904016802085,
-172.06909989019,-171.234182978295,-170.3992660664,-169.564349154505,-168.72943224261,
-167.894515330716,-167.4557484068),.UNSPECIFIED.);
#1026=B_SPLINE_CURVE_WITH_KNOTS('',3,(#60754,#60755,#60756,#60757,#60758,
#60759,#60760,#60761,#60762,#60763,#60764,#60765,#60766,#60767,#60768,#60769,
#60770,#60771,#60772,#60773,#60774,#60775,#60776,#60777,#60778),
 .UNSPECIFIED.,.F.,.F.,(4,3,3,3,3,3,3,3,4),(164.486466692813,165.321383604708,
166.156300516603,166.991217428498,167.826134340393,168.661051252288,169.495968164183,
170.330885076077,170.769651999993),.UNSPECIFIED.);
#1027=B_SPLINE_CURVE_WITH_KNOTS('',3,(#60783,#60784,#60785,#60786,#60787,
#60788,#60789,#60790,#60791,#60792,#60793,#60794,#60795,#60796,#60797,#60798,
#60799,#60800,#60801,#60802,#60803,#60804,#60805,#60806,#60807,#60808,#60809,
#60810),.UNSPECIFIED.,.F.,.F.,(4,3,3,3,3,3,3,3,3,4),(-180.022119021159,
-179.673196033865,-178.675011611454,-177.676827189044,-176.678642766634,
-176.179550555429,-175.680458344223,-174.682273921813,-174.183181710608,
-173.73893371398),.UNSPECIFIED.);
#1028=B_SPLINE_CURVE_WITH_KNOTS('',3,(#60811,#60812,#60813,#60814,#60815,
#60816,#60817,#60818,#60819,#60820,#60821,#60822,#60823,#60824,#60825,#60826,
#60827,#60828,#60829,#60830,#60831,#60832,#60833,#60834,#60835,#60836,#60837,
#60838,#60839,#60840,#60841),.UNSPECIFIED.,.F.,.F.,(4,3,3,3,3,3,3,3,3,3,
4),(170.769651999993,171.687720654582,172.685905076992,173.184997288198,
173.684089499403,174.183181710608,174.682273921813,175.680458344223,176.179550555429,
176.678642766634,177.052837307173),.UNSPECIFIED.);
#1029=B_SPLINE_CURVE_WITH_KNOTS('',3,(#60846,#60847,#60848,#60849,#60850,
#60851,#60852,#60853,#60854,#60855,#60856,#60857,#60858,#60859,#60860,#60861,
#60862,#60863,#60864,#60865,#60866,#60867,#60868,#60869,#60870,#60871,#60872,
#60873,#60874,#60875,#60876),.UNSPECIFIED.,.F.,.F.,(4,3,3,3,3,3,3,3,3,3,
4),(-186.305304328339,-185.662302568327,-184.664118145917,-183.665933723506,
-183.166841512301,-182.667749301096,-181.669564878686,-181.17047266748,
-180.671380456275,-180.17228824507,-180.022119021159),.UNSPECIFIED.);
#1030=B_SPLINE_CURVE_WITH_KNOTS('',3,(#60877,#60878,#60879,#60880,#60881,
#60882,#60883,#60884,#60885,#60886,#60887,#60888,#60889,#60890,#60891,#60892,
#60893,#60894,#60895,#60896,#60897,#60898,#60899,#60900,#60901,#60902,#60903,
#60904,#60905,#60906,#60907),.UNSPECIFIED.,.F.,.F.,(4,3,3,3,3,3,3,3,3,3,
4),(177.052837307173,177.676827189044,178.675011611455,179.673196033865,
180.17228824507,180.671380456275,181.17047266748,181.669564878686,182.667749301096,
183.166841512301,183.336022614352),.UNSPECIFIED.);
#1031=B_SPLINE_CURVE_WITH_KNOTS('',3,(#60912,#60913,#60914,#60915,#60916,
#60917,#60918,#60919,#60920,#60921,#60922,#60923,#60924,#60925,#60926,#60927,
#60928,#60929,#60930,#60931,#60932,#60933,#60934,#60935,#60936),
 .UNSPECIFIED.,.F.,.F.,(4,3,3,3,3,3,3,3,4),(-192.588489635518,-191.753572723623,
-190.918655811729,-190.083738899834,-189.248821987939,-188.413905076044,
-187.578988164149,-186.744071252255,-186.305304328339),.UNSPECIFIED.);
#1032=B_SPLINE_CURVE_WITH_KNOTS('',3,(#60937,#60938,#60939,#60940,#60941,
#60942,#60943,#60944,#60945,#60946,#60947,#60948,#60949,#60950,#60951,#60952,
#60953,#60954,#60955,#60956,#60957,#60958),.UNSPECIFIED.,.F.,.F.,(4,3,3,
3,3,3,3,4),(183.336022614352,183.665933723506,184.664118145917,185.662302568327,
186.660486990737,187.658671413148,188.656855835558,189.619207921532),
 .UNSPECIFIED.);
#1033=B_SPLINE_CURVE_WITH_KNOTS('',3,(#60963,#60964,#60965,#60966,#60967,
#60968,#60969,#60970,#60971,#60972,#60973,#60974,#60975,#60976,#60977,#60978,
#60979,#60980,#60981,#60982,#60983,#60984,#60985,#60986,#60987),
 .UNSPECIFIED.,.F.,.F.,(4,3,3,3,3,3,3,3,4),(-198.871674942698,-198.036758030803,
-197.201841118908,-196.366924207013,-195.532007295118,-194.697090383223,
-193.862173471329,-193.027256559434,-192.588489635518),.UNSPECIFIED.);
#1034=B_SPLINE_CURVE_WITH_KNOTS('',3,(#60988,#60989,#60990,#60991,#60992,
#60993,#60994,#60995,#60996,#60997,#60998,#60999,#61000,#61001,#61002,#61003,
#61004,#61005,#61006,#61007,#61008,#61009,#61010,#61011,#61012,#61013,#61014,
#61015,#61016,#61017,#61018,#61019,#61020,#61021),.UNSPECIFIED.,.F.,.F.,
(4,3,3,3,3,3,3,3,3,3,3,4),(189.619207921532,189.655040257969,190.653224680379,
191.152316891584,191.651409102789,192.6495935252,193.148685736405,193.64777794761,
194.146870158815,194.64596237002,195.644146792431,195.902393228711),
 .UNSPECIFIED.);
#1035=B_SPLINE_CURVE_WITH_KNOTS('',3,(#61026,#61027,#61028,#61029,#61030,
#61031,#61032,#61033,#61034,#61035,#61036,#61037,#61038,#61039,#61040,#61041,
#61042,#61043,#61044,#61045,#61046,#61047,#61048,#61049,#61050),
 .UNSPECIFIED.,.F.,.F.,(4,3,3,3,3,3,3,3,4),(-205.154860249877,-204.319943337983,
-203.485026426088,-202.650109514193,-201.815192602298,-200.980275690403,
-200.145358778508,-199.310441866614,-198.871674942698),.UNSPECIFIED.);
#1036=B_SPLINE_CURVE_WITH_KNOTS('',3,(#61051,#61052,#61053,#61054,#61055,
#61056,#61057,#61058,#61059,#61060,#61061,#61062,#61063,#61064,#61065,#61066,
#61067,#61068,#61069,#61070,#61071,#61072,#61073,#61074,#61075),
 .UNSPECIFIED.,.F.,.F.,(4,3,3,3,3,3,3,3,4),(195.902393228711,196.737310140606,
197.572227052501,198.407143964396,199.242060876291,200.076977788185,200.91189470008,
201.746811611975,202.185578535891),.UNSPECIFIED.);
#1037=B_SPLINE_CURVE_WITH_KNOTS('',3,(#61080,#61081,#61082,#61083,#61084,
#61085,#61086,#61087,#61088,#61089,#61090,#61091,#61092,#61093,#61094,#61095,
#61096,#61097,#61098,#61099,#61100,#61101,#61102,#61103,#61104,#61105,#61106,
#61107),.UNSPECIFIED.,.F.,.F.,(4,3,3,3,3,3,3,3,3,4),(-211.438045557057,
-210.616913128586,-209.618728706176,-208.620544283765,-208.12145207256,
-207.622359861355,-207.12326765015,-206.624175438945,-205.625991016534,
-205.154860249877),.UNSPECIFIED.);
#1038=B_SPLINE_CURVE_WITH_KNOTS('',3,(#61108,#61109,#61110,#61111,#61112,
#61113,#61114,#61115,#61116,#61117,#61118,#61119,#61120,#61121,#61122,#61123,
#61124,#61125,#61126,#61127,#61128,#61129,#61130,#61131,#61132,#61133,#61134,
#61135,#61136,#61137,#61138),.UNSPECIFIED.,.F.,.F.,(4,3,3,3,3,3,3,3,3,3,
4),(202.185578535891,202.631437749303,203.629622171714,204.627806594124,
205.126898805329,205.625991016534,206.624175438945,207.12326765015,207.622359861355,
208.12145207256,208.46876384307),.UNSPECIFIED.);
#1039=B_SPLINE_CURVE_WITH_KNOTS('',3,(#61143,#61144,#61145,#61146,#61147,
#61148,#61149,#61150,#61151,#61152,#61153,#61154,#61155,#61156,#61157,#61158,
#61159,#61160,#61161,#61162,#61163,#61164,#61165,#61166,#61167,#61168,#61169,
#61170,#61171,#61172,#61173,#61174,#61175,#61176),.UNSPECIFIED.,.F.,.F.,
(4,3,3,3,3,3,3,3,3,3,3,4),(-217.721230864237,-217.604204085459,-216.606019663048,
-215.607835240638,-215.108743029433,-214.609650818227,-214.110558607022,
-213.611466395817,-212.613281973407,-212.114189762202,-211.615097550996,
-211.438045557057),.UNSPECIFIED.);
#1040=B_SPLINE_CURVE_WITH_KNOTS('',3,(#61177,#61178,#61179,#61180,#61181,
#61182,#61183,#61184,#61185,#61186,#61187,#61188,#61189,#61190,#61191,#61192,
#61193,#61194,#61195,#61196,#61197,#61198,#61199,#61200,#61201,#61202,#61203,
#61204,#61205,#61206,#61207),.UNSPECIFIED.,.F.,.F.,(4,3,3,3,3,3,3,3,3,3,
4),(208.46876384307,208.620544283765,209.618728706176,210.616913128586,
211.615097550996,212.114189762202,212.613281973407,213.611466395817,214.110558607022,
214.609650818228,214.75194915025),.UNSPECIFIED.);
#1041=B_SPLINE_CURVE_WITH_KNOTS('',3,(#61212,#61213,#61214,#61215,#61216,
#61217,#61218,#61219,#61220,#61221,#61222,#61223,#61224,#61225,#61226,#61227,
#61228,#61229,#61230,#61231,#61232,#61233,#61234,#61235,#61236,#61237,#61238,
#61239,#61240,#61241,#61242),.UNSPECIFIED.,.F.,.F.,(4,3,3,3,3,3,3,3,3,3,
4),(-224.004416171416,-223.593310619921,-222.59512619751,-222.096033986305,
-221.5969417751,-221.097849563895,-220.59875735269,-219.600572930279,-219.101480719074,
-218.602388507869,-217.721230864237),.UNSPECIFIED.);
#1042=B_SPLINE_CURVE_WITH_KNOTS('',3,(#61243,#61244,#61245,#61246,#61247,
#61248,#61249,#61250,#61251,#61252,#61253,#61254,#61255,#61256,#61257,#61258,
#61259,#61260,#61261,#61262,#61263,#61264,#61265,#61266,#61267,#61268,#61269,
#61270),.UNSPECIFIED.,.F.,.F.,(4,3,3,3,3,3,3,3,3,4),(214.75194915025,215.108743029433,
215.607835240638,216.606019663048,217.604204085459,218.602388507869,219.101480719074,
219.600572930279,220.59875735269,221.03513445743),.UNSPECIFIED.);
#1043=B_SPLINE_CURVE_WITH_KNOTS('',3,(#61275,#61276,#61277,#61278,#61279,
#61280,#61281,#61282,#61283,#61284,#61285,#61286,#61287,#61288,#61289,#61290,
#61291,#61292,#61293,#61294,#61295,#61296,#61297,#61298,#61299),
 .UNSPECIFIED.,.F.,.F.,(4,3,3,3,3,3,3,3,4),(-230.287601478596,-229.452684566701,
-228.617767654806,-227.782850742911,-226.947933831016,-226.113016919121,
-225.278100007226,-224.443183095332,-224.004416171416),.UNSPECIFIED.);
#1044=B_SPLINE_CURVE_WITH_KNOTS('',3,(#61300,#61301,#61302,#61303,#61304,
#61305,#61306,#61307,#61308,#61309,#61310,#61311,#61312,#61313,#61314,#61315,
#61316,#61317,#61318,#61319,#61320,#61321,#61322,#61323,#61324),
 .UNSPECIFIED.,.F.,.F.,(4,3,3,3,3,3,3,3,4),(221.03513445743,221.870051369324,
222.704968281219,223.539885193114,224.374802105009,225.209719016904,226.044635928799,
226.879552840694,227.318319764609),.UNSPECIFIED.);
#1045=B_SPLINE_CURVE_WITH_KNOTS('',3,(#61329,#61330,#61331,#61332,#61333,
#61334,#61335,#61336,#61337,#61338,#61339,#61340,#61341,#61342,#61343,#61344,
#61345,#61346,#61347,#61348,#61349,#61350,#61351,#61352,#61353,#61354,#61355,
#61356,#61357,#61358,#61359),.UNSPECIFIED.,.F.,.F.,(4,3,3,3,3,3,3,3,3,3,
4),(-236.570786785775,-236.07061590005,-235.571523688845,-235.07243147764,
-234.573339266435,-233.575154844024,-233.076062632819,-232.576970421614,
-231.578785999204,-230.580601576793,-230.287601478596),.UNSPECIFIED.);
#1046=B_SPLINE_CURVE_WITH_KNOTS('',3,(#61360,#61361,#61362,#61363,#61364,
#61365,#61366,#61367,#61368,#61369,#61370,#61371,#61372,#61373,#61374,#61375,
#61376,#61377,#61378,#61379,#61380,#61381,#61382,#61383,#61384),
 .UNSPECIFIED.,.F.,.F.,(4,3,3,3,3,3,3,3,4),(227.318319764609,228.153236676504,
228.988153588399,229.823070500294,230.657987412188,231.492904324083,232.327821235978,
233.162738147873,233.601505071789),.UNSPECIFIED.);
#1047=B_SPLINE_CURVE_WITH_KNOTS('',3,(#61389,#61390,#61391,#61392,#61393,
#61394,#61395,#61396,#61397,#61398,#61399,#61400,#61401,#61402,#61403,#61404,
#61405,#61406,#61407,#61408,#61409,#61410,#61411,#61412,#61413,#61414,#61415,
#61416),.UNSPECIFIED.,.F.,.F.,(4,3,3,3,3,3,3,3,3,4),(-242.853972092955,
-242.558814645718,-242.059722434512,-241.560630223307,-240.562445800897,
-240.063353589692,-239.564261378486,-238.566076956076,-237.567892533666,
-236.570786785775),.UNSPECIFIED.);
#1048=B_SPLINE_CURVE_WITH_KNOTS('',3,(#61417,#61418,#61419,#61420,#61421,
#61422,#61423,#61424,#61425,#61426,#61427,#61428,#61429,#61430,#61431,#61432,
#61433,#61434,#61435,#61436,#61437,#61438,#61439,#61440,#61441,#61442,#61443,
#61444),.UNSPECIFIED.,.F.,.F.,(4,3,3,3,3,3,3,3,3,4),(233.601505071789,234.573339266435,
235.07243147764,235.571523688845,236.07061590005,236.569708111256,237.567892533666,
238.566076956076,239.564261378487,239.884690378968),.UNSPECIFIED.);
#1049=B_SPLINE_CURVE_WITH_KNOTS('',3,(#61449,#61450,#61451,#61452,#61453,
#61454,#61455,#61456,#61457,#61458,#61459,#61460,#61461,#61462,#61463,#61464,
#61465,#61466,#61467,#61468,#61469,#61470,#61471,#61472,#61473),
 .UNSPECIFIED.,.F.,.F.,(4,3,3,3,3,3,3,3,4),(-249.137157400134,-248.302240488239,
-247.467323576345,-246.63240666445,-245.797489752555,-244.96257284066,-244.127655928765,
-243.29273901687,-242.853972092955),.UNSPECIFIED.);
#1050=B_SPLINE_CURVE_WITH_KNOTS('',3,(#61474,#61475,#61476,#61477,#61478,
#61479,#61480,#61481,#61482,#61483,#61484,#61485,#61486,#61487,#61488,#61489,
#61490,#61491,#61492,#61493,#61494,#61495,#61496,#61497,#61498,#61499,#61500,
#61501,#61502,#61503,#61504),.UNSPECIFIED.,.F.,.F.,(4,3,3,3,3,3,3,3,3,3,
4),(239.884690378968,240.063353589692,240.562445800897,241.560630223307,
242.059722434512,242.558814645718,243.057906856923,243.556999068128,244.555183490538,
245.553367912949,246.167875686148),.UNSPECIFIED.);
#1051=B_SPLINE_CURVE_WITH_KNOTS('',3,(#61509,#61510,#61511,#61512,#61513,
#61514,#61515,#61516,#61517,#61518,#61519,#61520,#61521,#61522,#61523,#61524,
#61525,#61526,#61527,#61528,#61529,#61530,#61531,#61532,#61533,#61534,#61535,
#61536),.UNSPECIFIED.,.F.,.F.,(4,3,3,3,3,3,3,3,3,4),(-255.420342707314,
-254.537027714642,-254.037935503437,-253.538843292232,-252.540658869821,
-251.542474447411,-250.544290025,-250.045197813795,-249.54610560259,-249.137157400134),
 .UNSPECIFIED.);
#1052=B_SPLINE_CURVE_WITH_KNOTS('',3,(#61537,#61538,#61539,#61540,#61541,
#61542,#61543,#61544,#61545,#61546,#61547,#61548,#61549,#61550,#61551,#61552,
#61553,#61554,#61555,#61556,#61557,#61558,#61559,#61560,#61561,#61562,#61563,
#61564,#61565,#61566,#61567),.UNSPECIFIED.,.F.,.F.,(4,3,3,3,3,3,3,3,3,3,
4),(246.167875686148,246.551552335359,247.050644546564,247.549736757769,
248.54792118018,249.047013391385,249.54610560259,250.045197813795,250.544290025001,
251.542474447411,252.451060993327),.UNSPECIFIED.);
#1053=B_SPLINE_CURVE_WITH_KNOTS('',3,(#61572,#61573,#61574,#61575,#61576,
#61577,#61578,#61579,#61580,#61581,#61582,#61583,#61584,#61585,#61586,#61587,
#61588,#61589,#61590,#61591,#61592,#61593,#61594,#61595,#61596),
 .UNSPECIFIED.,.F.,.F.,(4,3,3,3,3,3,3,3,4),(-261.703528014493,-260.868611102599,
-260.033694190704,-259.198777278809,-258.363860366914,-257.528943455019,
-256.694026543124,-255.859109631229,-255.420342707314),.UNSPECIFIED.);
#1054=B_SPLINE_CURVE_WITH_KNOTS('',3,(#61597,#61598,#61599,#61600,#61601,
#61602,#61603,#61604,#61605,#61606,#61607,#61608,#61609,#61610,#61611,#61612,
#61613,#61614,#61615,#61616,#61617,#61618,#61619,#61620,#61621),
 .UNSPECIFIED.,.F.,.F.,(4,3,3,3,3,3,3,3,4),(252.451060993327,253.285977905222,
254.120894817117,254.955811729012,255.790728640907,256.625645552802,257.460562464697,
258.295479376592,258.734246300507),.UNSPECIFIED.);
#1055=B_SPLINE_CURVE_WITH_KNOTS('',3,(#61626,#61627,#61628,#61629,#61630,
#61631,#61632,#61633,#61634,#61635,#61636,#61637,#61638,#61639,#61640,#61641,
#61642,#61643,#61644,#61645,#61646,#61647,#61648,#61649,#61650),
 .UNSPECIFIED.,.F.,.F.,(4,3,3,3,3,3,3,3,4),(-267.986713321673,-267.151796409778,
-266.316879497883,-265.481962585988,-264.647045674094,-263.812128762199,
-262.977211850304,-262.142294938409,-261.703528014493),.UNSPECIFIED.);
#1056=B_SPLINE_CURVE_WITH_KNOTS('',3,(#61651,#61652,#61653,#61654,#61655,
#61656,#61657,#61658,#61659,#61660,#61661,#61662,#61663,#61664,#61665,#61666,
#61667,#61668,#61669,#61670,#61671,#61672,#61673,#61674,#61675),
 .UNSPECIFIED.,.F.,.F.,(4,3,3,3,3,3,3,3,4),(258.734246300507,259.569163212402,
260.404080124297,261.238997036192,262.073913948086,262.908830859981,263.743747771876,
264.578664683771,265.017431607686),.UNSPECIFIED.);
#1057=B_SPLINE_CURVE_WITH_KNOTS('',3,(#61680,#61681,#61682,#61683,#61684,
#61685,#61686,#61687,#61688,#61689,#61690,#61691,#61692,#61693,#61694,#61695,
#61696,#61697,#61698,#61699,#61700,#61701,#61702,#61703,#61704,#61705,#61706,
#61707,#61708,#61709,#61710),.UNSPECIFIED.,.F.,.F.,(4,3,3,3,3,3,3,3,3,3,
4),(-274.269898628853,-273.502531740439,-272.504347318028,-271.506162895618,
-271.007070684413,-270.507978473208,-270.008886262002,-269.509794050797,
-268.511609628387,-268.012517417182,-267.986713321673),.UNSPECIFIED.);
#1058=B_SPLINE_CURVE_WITH_KNOTS('',3,(#61711,#61712,#61713,#61714,#61715,
#61716,#61717,#61718,#61719,#61720,#61721,#61722,#61723,#61724,#61725,#61726,
#61727,#61728,#61729,#61730,#61731,#61732,#61733,#61734,#61735,#61736,#61737,
#61738,#61739,#61740,#61741),.UNSPECIFIED.,.F.,.F.,(4,3,3,3,3,3,3,3,3,3,
4),(265.017431607686,265.517056361156,266.515240783566,267.513425205977,
268.012517417182,268.511609628387,269.509794050797,270.008886262003,270.507978473208,
271.007070684413,271.300616914866),.UNSPECIFIED.);
#1059=B_SPLINE_CURVE_WITH_KNOTS('',3,(#61746,#61747,#61748,#61749,#61750,
#61751,#61752,#61753,#61754,#61755,#61756,#61757,#61758,#61759,#61760,#61761,
#61762,#61763,#61764,#61765,#61766,#61767,#61768,#61769,#61770,#61771,#61772,
#61773,#61774,#61775,#61776,#61777,#61778,#61779),.UNSPECIFIED.,.F.,.F.,
(4,3,3,3,3,3,3,3,3,3,3,4),(-280.553083936032,-280.489822697311,-279.491638274901,
-278.493453852491,-277.994361641285,-277.49526943008,-276.996177218875,
-276.49708500767,-275.498900585259,-274.999808374054,-274.500716162849,
-274.269898628853),.UNSPECIFIED.);
#1060=B_SPLINE_CURVE_WITH_KNOTS('',3,(#61780,#61781,#61782,#61783,#61784,
#61785,#61786,#61787,#61788,#61789,#61790,#61791,#61792,#61793,#61794,#61795,
#61796,#61797,#61798,#61799,#61800,#61801,#61802,#61803,#61804,#61805,#61806,
#61807,#61808,#61809,#61810),.UNSPECIFIED.,.F.,.F.,(4,3,3,3,3,3,3,3,3,3,
4),(271.300616914866,271.506162895618,272.504347318028,273.502531740439,
274.500716162849,274.999808374054,275.498900585259,276.49708500767,276.996177218875,
277.49526943008,277.583802222046),.UNSPECIFIED.);
#1061=B_SPLINE_CURVE_WITH_KNOTS('',3,(#61815,#61816,#61817,#61818,#61819,
#61820,#61821,#61822,#61823,#61824,#61825,#61826,#61827,#61828,#61829,#61830,
#61831,#61832,#61833,#61834,#61835,#61836,#61837,#61838,#61839,#61840,#61841,
#61842,#61843,#61844,#61845),.UNSPECIFIED.,.F.,.F.,(4,3,3,3,3,3,3,3,3,3,
4),(-286.836269243212,-286.478929231773,-285.480744809363,-284.981652598158,
-284.482560386953,-283.983468175747,-283.484375964542,-282.486191542132,
-281.987099330927,-281.488007119722,-280.553083936032),.UNSPECIFIED.);
#1062=B_SPLINE_CURVE_WITH_KNOTS('',3,(#61846,#61847,#61848,#61849,#61850,
#61851,#61852,#61853,#61854,#61855,#61856,#61857,#61858,#61859,#61860,#61861,
#61862,#61863,#61864,#61865,#61866,#61867,#61868,#61869,#61870,#61871,#61872,
#61873),.UNSPECIFIED.,.F.,.F.,(4,3,3,3,3,3,3,3,3,4),(277.583802222046,277.994361641285,
278.493453852491,279.491638274901,280.489822697311,281.488007119722,281.987099330927,
282.486191542132,283.484375964542,283.866987529225),.UNSPECIFIED.);
#1063=B_SPLINE_CURVE_WITH_KNOTS('',3,(#61878,#61879,#61880,#61881,#61882,
#61883,#61884,#61885,#61886,#61887,#61888,#61889,#61890,#61891,#61892,#61893,
#61894,#61895,#61896,#61897,#61898,#61899,#61900,#61901,#61902),
 .UNSPECIFIED.,.F.,.F.,(4,3,3,3,3,3,3,3,4),(-293.119454550391,-292.284537638496,
-291.449620726602,-290.614703814707,-289.779786902812,-288.944869990917,
-288.109953079022,-287.275036167127,-286.836269243212),.UNSPECIFIED.);
#1064=B_SPLINE_CURVE_WITH_KNOTS('',3,(#61903,#61904,#61905,#61906,#61907,
#61908,#61909,#61910,#61911,#61912,#61913,#61914,#61915,#61916,#61917,#61918,
#61919,#61920,#61921,#61922,#61923,#61924,#61925,#61926,#61927),
 .UNSPECIFIED.,.F.,.F.,(4,3,3,3,3,3,3,3,4),(283.866987529225,284.70190444112,
285.536821353015,286.37173826491,287.206655176804,288.041572088699,288.876489000594,
289.711405912489,290.150172836405),.UNSPECIFIED.);
#1065=B_SPLINE_CURVE_WITH_KNOTS('',3,(#61932,#61933,#61934,#61935,#61936,
#61937,#61938,#61939,#61940,#61941,#61942,#61943,#61944,#61945,#61946,#61947,
#61948,#61949,#61950,#61951,#61952,#61953,#61954,#61955,#61956,#61957,#61958,
#61959,#61960,#61961,#61962),.UNSPECIFIED.,.F.,.F.,(4,3,3,3,3,3,3,3,3,3,
4),(-299.402639857571,-298.956234511903,-298.457142300698,-297.958050089493,
-297.458957878287,-296.460773455877,-295.961681244672,-295.462589033467,
-294.464404611056,-293.466220188646,-293.119454550391),.UNSPECIFIED.);
#1066=B_SPLINE_CURVE_WITH_KNOTS('',3,(#61963,#61964,#61965,#61966,#61967,
#61968,#61969,#61970,#61971,#61972,#61973,#61974,#61975,#61976,#61977,#61978,
#61979,#61980,#61981,#61982,#61983,#61984,#61985,#61986,#61987,#61988,#61989,
#61990,#61991,#61992,#61993),.UNSPECIFIED.,.F.,.F.,(4,3,3,3,3,3,3,3,3,3,
4),(290.150172836405,290.471666921415,290.97075913262,291.469851343825,
291.96894355503,292.468035766236,293.466220188646,294.464404611056,295.462589033467,
295.961681244672,296.433358143584),.UNSPECIFIED.);
#1067=B_SPLINE_CURVE_WITH_KNOTS('',3,(#61998,#61999,#62000,#62001,#62002,
#62003,#62004,#62005,#62006,#62007,#62008,#62009,#62010,#62011,#62012,#62013,
#62014,#62015,#62016,#62017,#62018,#62019,#62020,#62021,#62022,#62023,#62024,
#62025,#62026,#62027,#62028),.UNSPECIFIED.,.F.,.F.,(4,3,3,3,3,3,3,3,3,3,
4),(-305.68582516475,-305.44443325757,-304.945341046365,-304.44624883516,
-303.448064412749,-302.948972201544,-302.449879990339,-301.451695567929,
-300.453511145518,-299.455326723108,-299.402639857571),.UNSPECIFIED.);
#1068=B_SPLINE_CURVE_WITH_KNOTS('',3,(#62029,#62030,#62031,#62032,#62033,
#62034,#62035,#62036,#62037,#62038,#62039,#62040,#62041,#62042,#62043,#62044,
#62045,#62046,#62047,#62048,#62049,#62050,#62051,#62052,#62053,#62054,#62055,
#62056,#62057,#62058,#62059),.UNSPECIFIED.,.F.,.F.,(4,3,3,3,3,3,3,3,3,3,
4),(296.433358143584,296.460773455877,297.458957878287,297.958050089493,
298.457142300698,298.956234511903,299.455326723108,300.453511145519,301.451695567929,
302.449879990339,302.716543450764),.UNSPECIFIED.);
#1069=B_SPLINE_CURVE_WITH_KNOTS('',3,(#62064,#62065,#62066,#62067,#62068,
#62069,#62070,#62071,#62072,#62073,#62074,#62075,#62076,#62077,#62078,#62079,
#62080,#62081,#62082,#62083,#62084,#62085,#62086,#62087,#62088),
 .UNSPECIFIED.,.F.,.F.,(4,3,3,3,3,3,3,3,4),(-311.96901047193,-311.134093560035,
-310.29917664814,-309.464259736245,-308.62934282435,-307.794425912456,-306.959509000561,
-306.124592088666,-305.68582516475),.UNSPECIFIED.);
#1070=B_SPLINE_CURVE_WITH_KNOTS('',3,(#62089,#62090,#62091,#62092,#62093,
#62094,#62095,#62096,#62097,#62098,#62099,#62100,#62101,#62102,#62103,#62104,
#62105,#62106,#62107,#62108,#62109,#62110,#62111,#62112,#62113,#62114,#62115,
#62116,#62117,#62118,#62119),.UNSPECIFIED.,.F.,.F.,(4,3,3,3,3,3,3,3,3,3,
4),(302.716543450764,302.948972201544,303.44806441275,304.44624883516,304.945341046365,
305.44443325757,305.943525468776,306.442617679981,307.440802102391,308.438986524802,
308.999728757943),.UNSPECIFIED.);
#1071=B_SPLINE_CURVE_WITH_KNOTS('',3,(#62124,#62125,#62126,#62127,#62128,
#62129,#62130,#62131,#62132,#62133,#62134,#62135,#62136,#62137,#62138,#62139,
#62140,#62141,#62142,#62143,#62144,#62145,#62146,#62147,#62148),
 .UNSPECIFIED.,.F.,.F.,(4,3,3,3,3,3,3,3,4),(-318.25219577911,-317.417278867215,
-316.58236195532,-315.747445043425,-314.91252813153,-314.077611219635,-313.24269430774,
-312.407777395845,-311.96901047193),.UNSPECIFIED.);
#1072=B_SPLINE_CURVE_WITH_KNOTS('',3,(#62149,#62150,#62151,#62152,#62153,
#62154,#62155,#62156,#62157,#62158,#62159,#62160,#62161,#62162,#62163,#62164,
#62165,#62166,#62167,#62168,#62169,#62170,#62171,#62172,#62173,#62174,#62175,
#62176,#62177,#62178,#62179),.UNSPECIFIED.,.F.,.F.,(4,3,3,3,3,3,3,3,3,3,
4),(308.999728757943,309.437170947212,309.936263158417,310.435355369622,
311.433539792033,311.932632003238,312.431724214443,312.930816425648,313.429908636853,
314.428093059264,315.282914065123),.UNSPECIFIED.);
#1073=B_SPLINE_CURVE_WITH_KNOTS('',3,(#62184,#62185,#62186,#62187,#62188,
#62189,#62190,#62191,#62192,#62193,#62194,#62195,#62196,#62197,#62198,#62199,
#62200,#62201,#62202,#62203,#62204,#62205,#62206,#62207,#62208),
 .UNSPECIFIED.,.F.,.F.,(4,3,3,3,3,3,3,3,4),(-324.535381086289,-323.700464174394,
-322.865547262499,-322.030630350604,-321.19571343871,-320.360796526815,
-319.52587961492,-318.690962703025,-318.25219577911),.UNSPECIFIED.);
#1074=B_SPLINE_CURVE_WITH_KNOTS('',3,(#62209,#62210,#62211,#62212,#62213,
#62214,#62215,#62216,#62217,#62218,#62219,#62220,#62221,#62222,#62223,#62224,
#62225,#62226,#62227,#62228,#62229,#62230,#62231,#62232,#62233),
 .UNSPECIFIED.,.F.,.F.,(4,3,3,3,3,3,3,3,4),(315.282914065123,316.117830977018,
316.952747888913,317.787664800807,318.622581712702,319.457498624597,320.292415536492,
321.127332448387,321.566099372303),.UNSPECIFIED.);
#1075=B_SPLINE_CURVE_WITH_KNOTS('',3,(#62238,#62239,#62240,#62241,#62242,
#62243,#62244,#62245,#62246,#62247,#62248,#62249,#62250,#62251,#62252,#62253,
#62254,#62255,#62256,#62257,#62258,#62259,#62260,#62261,#62262,#62263,#62264,
#62265),.UNSPECIFIED.,.F.,.F.,(4,3,3,3,3,3,3,3,3,4),(-330.818566393469,
-330.399043817829,-329.400859395419,-328.402674973009,-327.404490550598,
-326.905398339393,-326.406306128188,-325.907213916983,-325.408121705777,
-324.535381086289),.UNSPECIFIED.);
#1076=B_SPLINE_CURVE_WITH_KNOTS('',3,(#62266,#62267,#62268,#62269,#62270,
#62271,#62272,#62273,#62274,#62275,#62276,#62277,#62278,#62279,#62280,#62281,
#62282,#62283,#62284,#62285,#62286,#62287,#62288,#62289,#62290),
 .UNSPECIFIED.,.F.,.F.,(4,3,3,3,3,3,3,3,4),(321.566099372303,322.401016284197,
323.235933196092,324.070850107987,324.905767019882,325.740683931777,326.575600843672,
327.410517755567,327.849284679482),.UNSPECIFIED.);
#1077=B_SPLINE_CURVE_WITH_KNOTS('',3,(#62295,#62296,#62297,#62298,#62299,
#62300,#62301,#62302,#62303,#62304,#62305,#62306,#62307,#62308,#62309,#62310,
#62311,#62312,#62313,#62314,#62315,#62316,#62317,#62318,#62319,#62320,#62321,
#62322,#62323,#62324,#62325),.UNSPECIFIED.,.F.,.F.,(4,3,3,3,3,3,3,3,3,3,
4),(-337.101751700648,-336.388150352291,-335.389965929881,-334.391781507471,
-333.892689296266,-333.39359708506,-332.894504873855,-332.39541266265,-331.39722824024,
-330.898136029034,-330.818566393469),.UNSPECIFIED.);
#1078=B_SPLINE_CURVE_WITH_KNOTS('',3,(#62326,#62327,#62328,#62329,#62330,
#62331,#62332,#62333,#62334,#62335,#62336,#62337,#62338,#62339,#62340,#62341,
#62342,#62343,#62344,#62345,#62346,#62347,#62348,#62349,#62350,#62351,#62352,
#62353,#62354,#62355,#62356),.UNSPECIFIED.,.F.,.F.,(4,3,3,3,3,3,3,3,3,3,
4),(327.849284679482,328.402674973009,329.400859395419,330.399043817829,
330.898136029035,331.39722824024,332.39541266265,332.894504873855,333.39359708506,
333.892689296266,334.132469986662),.UNSPECIFIED.);
#1079=B_SPLINE_CURVE_WITH_KNOTS('',3,(#62361,#62362,#62363,#62364,#62365,
#62366,#62367,#62368,#62369,#62370,#62371,#62372,#62373,#62374,#62375,#62376,
#62377,#62378,#62379,#62380,#62381,#62382,#62383,#62384,#62385,#62386,#62387,
#62388,#62389,#62390,#62391,#62392,#62393,#62394),.UNSPECIFIED.,.F.,.F.,
(4,3,3,3,3,3,3,3,3,3,3,4),(-343.384937007828,-343.375441309164,-342.377256886754,
-341.379072464343,-340.879980253138,-340.380888041933,-339.881795830728,
-339.382703619523,-338.384519197112,-337.885426985907,-337.386334774702,
-337.101751700648),.UNSPECIFIED.);
#1080=B_SPLINE_CURVE_WITH_KNOTS('',3,(#62395,#62396,#62397,#62398,#62399,
#62400,#62401,#62402,#62403,#62404,#62405,#62406,#62407,#62408,#62409,#62410,
#62411,#62412,#62413,#62414,#62415,#62416,#62417,#62418,#62419,#62420,#62421,
#62422,#62423,#62424,#62425),.UNSPECIFIED.,.F.,.F.,(4,3,3,3,3,3,3,3,3,3,
4),(334.132469986662,334.391781507471,335.389965929881,336.388150352292,
337.386334774702,337.885426985907,338.384519197112,339.382703619523,339.881795830728,
340.380888041933,340.415655293841),.UNSPECIFIED.);
#1081=B_SPLINE_CURVE_WITH_KNOTS('',3,(#62430,#62431,#62432,#62433,#62434,
#62435,#62436,#62437,#62438,#62439,#62440,#62441,#62442,#62443,#62444,#62445,
#62446,#62447,#62448,#62449,#62450,#62451,#62452,#62453,#62454,#62455,#62456,
#62457,#62458,#62459,#62460),.UNSPECIFIED.,.F.,.F.,(4,3,3,3,3,3,3,3,3,3,
4),(-349.668122315007,-349.364547843626,-348.366363421216,-347.867271210011,
-347.368178998805,-346.8690867876,-346.369994576395,-345.371810153985,-344.87271794278,
-344.373625731574,-343.384937007828),.UNSPECIFIED.);
#1082=B_SPLINE_CURVE_WITH_KNOTS('',3,(#62461,#62462,#62463,#62464,#62465,
#62466,#62467,#62468,#62469,#62470,#62471,#62472,#62473,#62474,#62475,#62476,
#62477,#62478,#62479,#62480,#62481,#62482,#62483,#62484,#62485,#62486,#62487,
#62488),.UNSPECIFIED.,.F.,.F.,(4,3,3,3,3,3,3,3,3,4),(340.415655293841,340.879980253138,
341.379072464343,342.377256886754,343.375441309164,344.373625731574,344.87271794278,
345.371810153985,346.369994576395,346.698840601021),.UNSPECIFIED.);
#1083=B_SPLINE_CURVE_WITH_KNOTS('',3,(#62493,#62494,#62495,#62496,#62497,
#62498,#62499,#62500,#62501,#62502,#62503,#62504,#62505,#62506,#62507,#62508,
#62509,#62510,#62511,#62512,#62513,#62514,#62515,#62516,#62517),
 .UNSPECIFIED.,.F.,.F.,(4,3,3,3,3,3,3,3,4),(-355.951307622187,-355.116390710292,
-354.281473798397,-353.446556886502,-352.611639974607,-351.776723062712,
-350.941806150817,-350.106889238922,-349.668122315007),.UNSPECIFIED.);
#1084=B_SPLINE_CURVE_WITH_KNOTS('',3,(#62518,#62519,#62520,#62521,#62522,
#62523,#62524,#62525,#62526,#62527,#62528,#62529,#62530,#62531,#62532,#62533,
#62534,#62535,#62536,#62537,#62538,#62539,#62540,#62541,#62542),
 .UNSPECIFIED.,.F.,.F.,(4,3,3,3,3,3,3,3,4),(346.698840601021,347.533757512916,
348.36867442481,349.203591336705,350.0385082486,350.873425160495,351.70834207239,
352.543258984285,352.9820259082),.UNSPECIFIED.);
#1085=B_SPLINE_CURVE_WITH_KNOTS('',3,(#62547,#62548,#62549,#62550,#62551,
#62552,#62553,#62554,#62555,#62556,#62557,#62558,#62559,#62560,#62561,#62562,
#62563,#62564,#62565,#62566,#62567,#62568,#62569,#62570,#62571,#62572,#62573,
#62574,#62575,#62576,#62577),.UNSPECIFIED.,.F.,.F.,(4,3,3,3,3,3,3,3,3,3,
4),(-362.234492929366,-361.841853123756,-361.34276091255,-360.843668701345,
-360.34457649014,-359.34639206773,-358.847299856525,-358.348207645319,-357.350023222909,
-356.351838800499,-355.951307622187),.UNSPECIFIED.);
#1086=B_SPLINE_CURVE_WITH_KNOTS('',3,(#62578,#62579,#62580,#62581,#62582,
#62583,#62584,#62585,#62586,#62587,#62588,#62589,#62590,#62591,#62592,#62593,
#62594,#62595,#62596,#62597,#62598,#62599,#62600,#62601,#62602,#62603,#62604,
#62605,#62606,#62607,#62608),.UNSPECIFIED.,.F.,.F.,(4,3,3,3,3,3,3,3,3,3,
4),(352.9820259082,353.357285533268,353.856377744473,354.355469955678,354.854562166883,
355.353654378088,356.351838800499,357.350023222909,358.348207645319,358.847299856525,
359.26521121538),.UNSPECIFIED.);
#1087=B_SPLINE_CURVE_WITH_KNOTS('',3,(#62613,#62614,#62615,#62616,#62617,
#62618,#62619,#62620,#62621,#62622,#62623,#62624,#62625,#62626,#62627,#62628,
#62629,#62630,#62631,#62632,#62633,#62634,#62635,#62636,#62637,#62638,#62639,
#62640,#62641,#62642,#62643),.UNSPECIFIED.,.F.,.F.,(4,3,3,3,3,3,3,3,3,3,
4),(-368.517678236546,-368.330051869423,-367.830959658218,-367.331867447013,
-366.333683024602,-365.834590813397,-365.335498602192,-364.337314179782,
-363.339129757371,-362.340945334961,-362.234492929366),.UNSPECIFIED.);
#1088=B_SPLINE_CURVE_WITH_KNOTS('',3,(#62644,#62645,#62646,#62647,#62648,
#62649,#62650,#62651,#62652,#62653,#62654,#62655,#62656,#62657,#62658,#62659,
#62660,#62661,#62662,#62663,#62664,#62665,#62666,#62667,#62668,#62669,#62670,
#62671,#62672,#62673,#62674),.UNSPECIFIED.,.F.,.F.,(4,3,3,3,3,3,3,3,3,3,
4),(359.26521121538,359.34639206773,360.34457649014,360.843668701345,361.342760912551,
361.841853123756,362.340945334961,363.339129757371,364.337314179782,365.335498602192,
365.54839652256),.UNSPECIFIED.);
#1089=B_SPLINE_CURVE_WITH_KNOTS('',3,(#62681,#62682,#62683,#62684,#62685,
#62686,#62687,#62688,#62689,#62690,#62691,#62692,#62693,#62694,#62695,#62696,
#62697,#62698,#62699,#62700,#62701,#62702),.UNSPECIFIED.,.F.,.F.,(4,3,3,
3,3,3,3,4),(-374.319158403885,-373.48424149199,-372.649324580095,-371.8144076682,
-370.979490756305,-370.14457384441,-369.309656932515,-368.517678236546),
 .UNSPECIFIED.);
#1090=B_SPLINE_CURVE_WITH_KNOTS('',3,(#62703,#62704,#62705,#62706,#62707,
#62708,#62709,#62710,#62711,#62712,#62713,#62714,#62715,#62716,#62717,#62718,
#62719,#62720,#62721,#62722,#62723,#62724,#62725,#62726,#62727,#62728,#62729,
#62730,#62731,#62732,#62733),.UNSPECIFIED.,.F.,.F.,(4,3,3,3,3,3,3,3,3,3,
4),(365.54839652256,365.834590813397,366.333683024602,367.331867447013,
367.830959658218,368.330051869423,368.829144080628,369.328236291833,370.326420714244,
371.324605136654,371.831581829739),.UNSPECIFIED.);
#1091=B_SPLINE_CURVE_WITH_KNOTS('',3,(#62739,#62740,#62741,#62742,#62743,
#62744,#62745,#62746,#62747,#62748,#62749,#62750,#62751,#62752,#62753,#62754),
 .UNSPECIFIED.,.F.,.F.,(4,3,3,3,3,4),(380.132711084365,380.584976729012,
381.45314130285,382.321305876688,383.189470450526,383.85920477902),
 .UNSPECIFIED.);
#1092=B_SPLINE_CURVE_WITH_KNOTS('',3,(#62757,#62758,#62759,#62760,#62761,
#62762,#62763,#62764),.UNSPECIFIED.,.F.,.F.,(4,1,1,1,1,4),(380.132711084365,
380.623918813691,381.123011024896,381.622103236102,382.121195447307,382.620287658512),
 .UNSPECIFIED.);
#1093=B_SPLINE_CURVE_WITH_KNOTS('',3,(#62769,#62770,#62771,#62772,#62773,
#62774,#62775,#62776,#62777,#62778,#62779,#62780,#62781),.UNSPECIFIED.,
 .F.,.F.,(4,1,1,1,1,1,1,1,1,1,4),(373.849525777185,373.95597818278,374.95416260519,
375.9523470276,376.950531450011,377.449623661216,377.948715872421,378.946900294831,
379.445992506037,379.945084717242,380.132711084365),.UNSPECIFIED.);
#1094=B_SPLINE_CURVE_WITH_KNOTS('',3,(#62782,#62783,#62784,#62785,#62786,
#62787,#62788,#62789,#62790,#62791,#62792,#62793,#62794),.UNSPECIFIED.,
 .F.,.F.,(4,1,1,1,1,1,1,1,1,1,4),(373.849525777185,374.135720068024,374.634812279229,
375.632996701639,376.132088912845,376.63118112405,377.130273335255,377.62936554646,
378.627549968871,379.625734391281,380.132711084365),.UNSPECIFIED.);
#1095=B_SPLINE_CURVE_WITH_KNOTS('',3,(#62799,#62800,#62801,#62802,#62803,
#62804,#62805,#62806,#62807,#62808,#62809,#62810,#62811),.UNSPECIFIED.,
 .F.,.F.,(4,1,1,1,1,1,1,1,1,1,4),(367.566340470006,367.966871648318,368.965056070728,
369.963240493138,370.462332704343,370.961424915549,371.959609337959,372.458701549164,
372.957793760369,373.456885971574,373.849525777185),.UNSPECIFIED.);
#1096=B_SPLINE_CURVE_WITH_KNOTS('',3,(#62812,#62813,#62814,#62815,#62816,
#62817,#62818,#62819,#62820,#62821,#62822,#62823,#62824),.UNSPECIFIED.,
 .F.,.F.,(4,1,1,1,1,1,1,1,1,1,4),(367.566340470006,367.647521322357,368.645705744767,
369.144797955972,369.643890167177,370.142982378382,370.642074589588,371.640259011998,
372.638443434408,373.636627856819,373.849525777185),.UNSPECIFIED.);
#1097=B_SPLINE_CURVE_WITH_KNOTS('',3,(#62829,#62830,#62831,#62832,#62833,
#62834,#62835,#62836,#62837,#62838,#62839,#62840,#62841,#62842,#62843,#62844,
#62845,#62846,#62847,#62848,#62849,#62850,#62851,#62852,#62853,#62854,#62855,
#62856),.UNSPECIFIED.,.F.,.F.,(4,3,3,3,3,3,3,3,3,4),(361.283155162826,361.485356104573,
362.353520678412,363.22168525225,364.089849826088,364.958014399926,365.826178973764,
366.694343547602,367.56250812144,367.566340470006),.UNSPECIFIED.);
#1098=B_SPLINE_CURVE_WITH_KNOTS('',3,(#62857,#62858,#62859,#62860,#62861,
#62862,#62863,#62864,#62865,#62866,#62867,#62868,#62869),.UNSPECIFIED.,
 .F.,.F.,(4,1,1,1,1,1,1,1,1,1,4),(361.283155162826,361.658414787894,362.1575069991,
362.656599210305,363.15569142151,363.654783632715,364.652968055125,365.651152477536,
366.649336899946,367.148429111151,367.566340470006),.UNSPECIFIED.);
#1099=B_SPLINE_CURVE_WITH_KNOTS('',3,(#62874,#62875,#62876,#62877,#62878,
#62879,#62880,#62881,#62882,#62883,#62884,#62885,#62886),.UNSPECIFIED.,
 .F.,.F.,(4,1,1,1,1,1,1,1,1,1,4),(354.999969855647,355.988658579393,356.487750790598,
356.986843001804,357.985027424214,358.484119635419,358.983211846624,359.48230405783,
359.981396269035,360.979580691445,361.283155162826),.UNSPECIFIED.);
#1100=B_SPLINE_CURVE_WITH_KNOTS('',3,(#62887,#62888,#62889,#62890,#62891,
#62892,#62893,#62894,#62895,#62896,#62897,#62898,#62899,#62900,#62901,#62902,
#62903,#62904,#62905,#62906,#62907,#62908,#62909,#62910,#62911,#62912,#62913,
#62914),.UNSPECIFIED.,.F.,.F.,(4,3,3,3,3,3,3,3,3,4),(354.999969855647,355.037451541037,
355.905616114875,356.773780688713,357.641945262551,358.510109836389,359.378274410227,
360.246438984065,361.114603557904,361.283155162826),.UNSPECIFIED.);
#1101=B_SPLINE_CURVE_WITH_KNOTS('',3,(#62919,#62920,#62921,#62922,#62923,
#62924,#62925,#62926,#62927,#62928,#62929,#62930,#62931,#62932),
 .UNSPECIFIED.,.F.,.F.,(4,1,1,1,1,1,1,1,1,1,1,4),(348.716784548467,349.001367622521,
349.500459833726,349.999552044931,350.997736467341,351.496828678547,351.995920889752,
352.495013100957,352.994105312162,353.992289734573,354.990474156983,354.999969855647),
 .UNSPECIFIED.);
#1102=B_SPLINE_CURVE_WITH_KNOTS('',3,(#62933,#62934,#62935,#62936,#62937,
#62938,#62939,#62940,#62941,#62942,#62943,#62944),.UNSPECIFIED.,.F.,.F.,
(4,1,1,1,1,1,1,1,1,4),(348.716784548467,349.181109507765,349.68020171897,
350.67838614138,351.676570563791,352.674754986201,353.173847197406,353.672939408612,
354.671123831022,354.999969855647),.UNSPECIFIED.);
#1103=B_SPLINE_CURVE_WITH_KNOTS('',3,(#62949,#62950,#62951,#62952,#62953,
#62954,#62955,#62956,#62957,#62958,#62959,#62960,#62961),.UNSPECIFIED.,
 .F.,.F.,(4,1,1,1,1,1,1,1,1,1,4),(342.433599241287,342.513168876853,343.012261088059,
344.010445510469,344.509537721674,345.008629932879,345.507722144084,346.00681435529,
347.0049987777,348.00318320011,348.716784548467),.UNSPECIFIED.);
#1104=B_SPLINE_CURVE_WITH_KNOTS('',3,(#62962,#62963,#62964,#62965,#62966,
#62967,#62968,#62969,#62970,#62971,#62972,#62973,#62974),.UNSPECIFIED.,
 .F.,.F.,(4,1,1,1,1,1,1,1,1,1,4),(342.433599241288,342.692910762098,343.691095184508,
344.689279606918,345.687464029329,346.186556240534,346.685648451739,347.683832874149,
348.182925085355,348.68201729656,348.716784548467),.UNSPECIFIED.);
#1105=B_SPLINE_CURVE_WITH_KNOTS('',3,(#62979,#62980,#62981,#62982,#62983,
#62984,#62985,#62986,#62987,#62988,#62989,#62990),.UNSPECIFIED.,.F.,.F.,
(4,1,1,1,1,1,1,1,1,4),(336.150413934108,337.023154553596,337.522246764802,
338.021338976007,338.520431187212,339.019523398417,340.017707820827,341.015892243238,
342.014076665648,342.433599241287),.UNSPECIFIED.);
#1106=B_SPLINE_CURVE_WITH_KNOTS('',3,(#62991,#62992,#62993,#62994,#62995,
#62996,#62997,#62998,#62999,#63000,#63001,#63002,#63003),.UNSPECIFIED.,
 .F.,.F.,(4,1,1,1,1,1,1,1,1,1,4),(336.150413934108,336.703804227635,337.701988650046,
338.700173072456,339.199265283661,339.698357494866,340.696541917277,341.195634128482,
341.694726339687,342.193818550892,342.433599241288),.UNSPECIFIED.);
#1107=B_SPLINE_CURVE_WITH_KNOTS('',3,(#63008,#63009,#63010,#63011,#63012,
#63013,#63014,#63015,#63016,#63017,#63018,#63019,#63020,#63021,#63022,#63023,
#63024,#63025,#63026,#63027,#63028,#63029,#63030,#63031,#63032),
 .UNSPECIFIED.,.F.,.F.,(4,3,3,3,3,3,3,3,4),(329.867228626928,330.231431446402,
331.09959602024,331.967760594078,332.835925167916,333.704089741754,334.572254315592,
335.44041888943,336.150413934108),.UNSPECIFIED.);
#1108=B_SPLINE_CURVE_WITH_KNOTS('',3,(#63033,#63034,#63035,#63036,#63037,
#63038,#63039,#63040,#63041,#63042,#63043,#63044,#63045),.UNSPECIFIED.,
 .F.,.F.,(4,1,1,1,1,1,1,1,1,1,4),(329.867228626928,330.714697693173,331.712882115584,
332.211974326789,332.711066537994,333.709250960404,334.208343171609,334.707435382815,
335.20652759402,335.705619805225,336.150413934108),.UNSPECIFIED.);
#1109=B_SPLINE_CURVE_WITH_KNOTS('',3,(#63050,#63051,#63052,#63053,#63054,
#63055,#63056,#63057,#63058,#63059,#63060,#63061),.UNSPECIFIED.,.F.,.F.,
(4,1,1,1,1,1,1,1,1,4),(323.584043319749,324.046757062262,324.545849273467,
325.044941484672,326.043125907082,327.041310329493,328.039494751903,328.538586963108,
329.037679174313,329.867228626928),.UNSPECIFIED.);
#1110=B_SPLINE_CURVE_WITH_KNOTS('',3,(#63062,#63063,#63064,#63065,#63066,
#63067,#63068,#63069,#63070,#63071,#63072,#63073,#63074,#63075),
 .UNSPECIFIED.,.F.,.F.,(4,1,1,1,1,1,1,1,1,1,1,4),(323.584043319749,323.727406736301,
324.725591158711,325.224683369916,325.723775581121,326.721960003532,327.221052214737,
327.720144425942,328.219236637147,328.718328848352,329.716513270763,329.867228626928),
 .UNSPECIFIED.);
#1111=B_SPLINE_CURVE_WITH_KNOTS('',3,(#63080,#63081,#63082,#63083,#63084,
#63085,#63086,#63087,#63088,#63089,#63090,#63091,#63092,#63093,#63094,#63095,
#63096,#63097,#63098,#63099,#63100,#63101,#63102,#63103,#63104),
 .UNSPECIFIED.,.F.,.F.,(4,3,3,3,3,3,3,3,4),(317.300858012569,318.077127412668,
318.945291986507,319.813456560345,320.681621134183,321.549785708021,322.417950281859,
323.286114855697,323.584043319749),.UNSPECIFIED.);
#1112=B_SPLINE_CURVE_WITH_KNOTS('',3,(#63105,#63106,#63107,#63108,#63109,
#63110,#63111,#63112,#63113,#63114,#63115,#63116,#63117),.UNSPECIFIED.,
 .F.,.F.,(4,1,1,1,1,1,1,1,1,1,4),(317.300858012569,317.738300201839,318.237392413044,
318.736484624249,319.734669046659,320.233761257864,320.73285346907,321.231945680275,
321.73103789148,322.72922231389,323.584043319749),.UNSPECIFIED.);
#1113=B_SPLINE_CURVE_WITH_KNOTS('',3,(#63122,#63123,#63124,#63125,#63126,
#63127,#63128,#63129,#63130,#63131,#63132,#63133,#63134),.UNSPECIFIED.,
 .F.,.F.,(4,1,1,1,1,1,1,1,1,1,4),(311.01767270539,311.070359570927,312.068543993337,
313.066728415748,314.064912838158,314.564005049363,315.063097260568,316.061281682979,
316.560373894184,317.059466105389,317.300858012569),.UNSPECIFIED.);
#1114=B_SPLINE_CURVE_WITH_KNOTS('',3,(#63135,#63136,#63137,#63138,#63139,
#63140,#63141,#63142,#63143,#63144,#63145,#63146,#63147),.UNSPECIFIED.,
 .F.,.F.,(4,1,1,1,1,1,1,1,1,1,4),(311.01767270539,311.250101456171,311.749193667376,
312.747378089787,313.246470300992,313.745562512197,314.244654723402,314.743746934607,
315.741931357018,316.740115779428,317.300858012569),.UNSPECIFIED.);
#1115=B_SPLINE_CURVE_WITH_KNOTS('',3,(#63152,#63153,#63154,#63155,#63156,
#63157,#63158,#63159,#63160,#63161,#63162,#63163,#63164),.UNSPECIFIED.,
 .F.,.F.,(4,1,1,1,1,1,1,1,1,1,4),(304.73448739821,305.081253036465,306.079437458875,
307.077621881286,307.576714092491,308.075806303696,309.073990726106,309.573082937311,
310.072175148517,310.571267359722,311.01767270539),.UNSPECIFIED.);
#1116=B_SPLINE_CURVE_WITH_KNOTS('',3,(#63165,#63166,#63167,#63168,#63169,
#63170,#63171,#63172,#63173,#63174,#63175,#63176,#63177),.UNSPECIFIED.,
 .F.,.F.,(4,1,1,1,1,1,1,1,1,1,4),(304.73448739821,304.761902710504,305.760087132914,
306.259179344119,306.758271555325,307.25736376653,307.756455977735,308.754640400145,
309.752824822556,310.751009244966,311.01767270539),.UNSPECIFIED.);
#1117=B_SPLINE_CURVE_WITH_KNOTS('',3,(#63182,#63183,#63184,#63185,#63186,
#63187,#63188,#63189,#63190,#63191,#63192,#63193,#63194,#63195,#63196,#63197,
#63198,#63199,#63200,#63201,#63202,#63203,#63204,#63205,#63206),
 .UNSPECIFIED.,.F.,.F.,(4,3,3,3,3,3,3,3,4),(298.451302091031,298.97750678823,
299.845671362068,300.713835935906,301.582000509745,302.450165083583,303.318329657421,
304.186494231259,304.73448739821),.UNSPECIFIED.);
#1118=B_SPLINE_CURVE_WITH_KNOTS('',3,(#63207,#63208,#63209,#63210,#63211,
#63212,#63213,#63214,#63215,#63216,#63217,#63218,#63219),.UNSPECIFIED.,
 .F.,.F.,(4,1,1,1,1,1,1,1,1,1,4),(298.451302091031,298.772796176042,299.271888387247,
299.770980598452,300.270072809657,300.769165020862,301.767349443273,302.765533865683,
303.763718288094,304.262810499299,304.73448739821),.UNSPECIFIED.);
#1119=B_SPLINE_CURVE_WITH_KNOTS('',3,(#63224,#63225,#63226,#63227,#63228,
#63229,#63230,#63231,#63232,#63233,#63234,#63235,#63236),.UNSPECIFIED.,
 .F.,.F.,(4,1,1,1,1,1,1,1,1,1,4),(292.168116783851,293.103039967541,293.602132178746,
294.101224389951,295.099408812361,295.598501023566,296.097593234772,296.596685445977,
297.095777657182,298.093962079592,298.451302091031),.UNSPECIFIED.);
#1120=B_SPLINE_CURVE_WITH_KNOTS('',3,(#63237,#63238,#63239,#63240,#63241,
#63242,#63243,#63244,#63245,#63246,#63247,#63248,#63249,#63250,#63251,#63252,
#63253,#63254,#63255,#63256,#63257,#63258,#63259,#63260,#63261),
 .UNSPECIFIED.,.F.,.F.,(4,3,3,3,3,3,3,3,4),(292.168116783851,292.529602224694,
293.397766798532,294.26593137237,295.134095946208,296.002260520046,296.870425093884,
297.738589667722,298.451302091031),.UNSPECIFIED.);
#1121=B_SPLINE_CURVE_WITH_KNOTS('',3,(#63266,#63267,#63268,#63269,#63270,
#63271,#63272,#63273,#63274,#63275,#63276,#63277,#63278,#63279),
 .UNSPECIFIED.,.F.,.F.,(4,1,1,1,1,1,1,1,1,1,1,4),(285.884931476671,286.115749010668,
286.614841221873,287.113933433078,288.112117855489,288.611210066694,289.110302277899,
289.609394489104,290.108486700309,291.10667112272,292.10485554513,292.168116783851),
 .UNSPECIFIED.);
#1122=B_SPLINE_CURVE_WITH_KNOTS('',3,(#63280,#63281,#63282,#63283,#63284,
#63285,#63286,#63287,#63288,#63289,#63290,#63291),.UNSPECIFIED.,.F.,.F.,
(4,1,1,1,1,1,1,1,1,4),(285.884931476671,286.295490895912,286.794583107117,
287.792767529528,288.790951951938,289.789136374348,290.288228585554,290.787320796759,
291.785505219169,292.168116783851),.UNSPECIFIED.);
#1123=B_SPLINE_CURVE_WITH_KNOTS('',3,(#63296,#63297,#63298,#63299,#63300,
#63301,#63302,#63303,#63304,#63305,#63306,#63307,#63308),.UNSPECIFIED.,
 .F.,.F.,(4,1,1,1,1,1,1,1,1,1,4),(279.601746169492,279.627550265001,280.126642476206,
281.124826898616,281.623919109821,282.123011321027,282.622103532232,283.121195743437,
284.119380165847,285.117564588258,285.884931476671),.UNSPECIFIED.);
#1124=B_SPLINE_CURVE_WITH_KNOTS('',3,(#63309,#63310,#63311,#63312,#63313,
#63314,#63315,#63316,#63317,#63318,#63319,#63320,#63321),.UNSPECIFIED.,
 .F.,.F.,(4,1,1,1,1,1,1,1,1,1,4),(279.601746169492,279.807292150245,280.805476572655,
281.803660995066,282.801845417476,283.300937628681,283.800029839886,284.798214262297,
285.297306473502,285.796398684707,285.884931476671),.UNSPECIFIED.);
#1125=B_SPLINE_CURVE_WITH_KNOTS('',3,(#63326,#63327,#63328,#63329,#63330,
#63331,#63332,#63333,#63334,#63335,#63336,#63337,#63338,#63339,#63340,#63341,
#63342,#63343,#63344,#63345,#63346,#63347,#63348,#63349,#63350),
 .UNSPECIFIED.,.F.,.F.,(4,3,3,3,3,3,3,3,4),(273.318560862312,273.800734146925,
274.668898720763,275.537063294602,276.40522786844,277.273392442278,278.141557016116,
279.009721589954,279.601746169492),.UNSPECIFIED.);
#1126=B_SPLINE_CURVE_WITH_KNOTS('',3,(#63351,#63352,#63353,#63354,#63355,
#63356,#63357,#63358,#63359,#63360,#63361,#63362,#63363),.UNSPECIFIED.,
 .F.,.F.,(4,1,1,1,1,1,1,1,1,1,4),(273.318560862312,273.818185615783,274.816370038193,
275.814554460603,276.313646671809,276.812738883014,277.810923305424,278.310015516629,
278.809107727834,279.30819993904,279.601746169492),.UNSPECIFIED.);
#1127=B_SPLINE_CURVE_WITH_KNOTS('',3,(#63368,#63369,#63370,#63371,#63372,
#63373,#63374,#63375,#63376,#63377,#63378,#63379,#63380,#63381,#63382,#63383,
#63384,#63385,#63386,#63387,#63388,#63389,#63390,#63391,#63392),
 .UNSPECIFIED.,.F.,.F.,(4,3,3,3,3,3,3,3,4),(267.035375555133,267.723582130059,
268.591746703897,269.459911277735,270.328075851573,271.196240425411,272.064404999249,
272.932569573087,273.318560862312),.UNSPECIFIED.);
#1128=B_SPLINE_CURVE_WITH_KNOTS('',3,(#63393,#63394,#63395,#63396,#63397,
#63398,#63399,#63400,#63401,#63402,#63403,#63404,#63405,#63406,#63407,#63408,
#63409,#63410,#63411,#63412,#63413,#63414,#63415,#63416,#63417),
 .UNSPECIFIED.,.F.,.F.,(4,3,3,3,3,3,3,3,4),(267.035375555133,267.352829583389,
268.220994157227,269.089158731065,269.957323304903,270.825487878741,271.693652452579,
272.561817026417,273.318560862312),.UNSPECIFIED.);
#1129=B_SPLINE_CURVE_WITH_KNOTS('',3,(#63422,#63423,#63424,#63425,#63426,
#63427,#63428,#63429,#63430,#63431,#63432,#63433),.UNSPECIFIED.,.F.,.F.,
(4,1,1,1,1,1,1,1,1,4),(260.752190247953,261.161138450409,261.660230661614,
262.159322872819,263.15750729523,264.15569171764,265.15387614005,265.652968351256,
266.152060562461,267.035375555133),.UNSPECIFIED.);
#1130=B_SPLINE_CURVE_WITH_KNOTS('',3,(#63434,#63435,#63436,#63437,#63438,
#63439,#63440,#63441,#63442,#63443,#63444,#63445,#63446,#63447),
 .UNSPECIFIED.,.F.,.F.,(4,1,1,1,1,1,1,1,1,1,1,4),(260.752190247953,260.841788124448,
261.839972546858,262.339064758064,262.838156969269,263.836341391679,264.335433602884,
264.834525814089,265.333618025295,265.8327102365,266.83089465891,267.035375555133),
 .UNSPECIFIED.);
#1131=B_SPLINE_CURVE_WITH_KNOTS('',3,(#63452,#63453,#63454,#63455,#63456,
#63457,#63458,#63459,#63460,#63461,#63462,#63463,#63464,#63465,#63466,#63467,
#63468,#63469,#63470,#63471,#63472,#63473,#63474,#63475,#63476),
 .UNSPECIFIED.,.F.,.F.,(4,3,3,3,3,3,3,3,4),(254.469004940774,254.701113522487,
255.569278096325,256.437442670163,257.305607244001,258.17377181784,259.041936391678,
259.910100965516,260.752190247953),.UNSPECIFIED.);
#1132=B_SPLINE_CURVE_WITH_KNOTS('',3,(#63477,#63478,#63479,#63480,#63481,
#63482,#63483,#63484,#63485,#63486,#63487,#63488,#63489),.UNSPECIFIED.,
 .F.,.F.,(4,1,1,1,1,1,1,1,1,1,4),(254.469004940774,254.852681589986,255.351773801191,
255.850866012396,256.849050434807,257.348142646012,257.847234857217,258.346327068422,
258.845419279627,259.843603702038,260.752190247953),.UNSPECIFIED.);
#1133=B_SPLINE_CURVE_WITH_KNOTS('',3,(#63494,#63495,#63496,#63497,#63498,
#63499,#63500,#63501,#63502,#63503,#63504,#63505),.UNSPECIFIED.,.F.,.F.,
(4,1,1,1,1,1,1,1,1,4),(248.185819633594,249.182925381485,250.181109803895,
251.179294226305,251.678386437511,252.177478648716,253.175663071126,253.674755282331,
254.173847493536,254.469004940774),.UNSPECIFIED.);
#1134=B_SPLINE_CURVE_WITH_KNOTS('',3,(#63506,#63507,#63508,#63509,#63510,
#63511,#63512,#63513,#63514,#63515,#63516,#63517,#63518),.UNSPECIFIED.,
 .F.,.F.,(4,1,1,1,1,1,1,1,1,1,4),(248.185819633594,248.364482844319,248.863575055524,
249.861759477934,250.360851689139,250.859943900344,251.35903611155,251.858128322755,
252.856312745165,253.854497167575,254.469004940774),.UNSPECIFIED.);
#1135=B_SPLINE_CURVE_WITH_KNOTS('',3,(#63523,#63524,#63525,#63526,#63527,
#63528,#63529,#63530,#63531,#63532,#63533,#63534,#63535,#63536),
 .UNSPECIFIED.,.F.,.F.,(4,1,1,1,1,1,1,1,1,1,1,4),(241.902634326414,242.195634424612,
243.193818847023,244.192003269433,244.691095480638,245.190187691843,246.188372114254,
246.687464325459,247.186556536664,247.685648747869,248.184740959074,248.185819633594),
 .UNSPECIFIED.);
#1136=B_SPLINE_CURVE_WITH_KNOTS('',3,(#63537,#63538,#63539,#63540,#63541,
#63542,#63543,#63544,#63545,#63546,#63547,#63548),.UNSPECIFIED.,.F.,.F.,
(4,1,1,1,1,1,1,1,1,4),(241.902634326415,242.874468521062,243.373560732267,
243.872652943472,244.371745154677,244.870837365882,245.869021788293,246.867206210703,
247.865390633113,248.185819633594),.UNSPECIFIED.);
#1137=B_SPLINE_CURVE_WITH_KNOTS('',3,(#63553,#63554,#63555,#63556,#63557,
#63558,#63559,#63560,#63561,#63562,#63563,#63564,#63565,#63566,#63567,#63568,
#63569,#63570,#63571,#63572,#63573,#63574,#63575,#63576,#63577),
 .UNSPECIFIED.,.F.,.F.,(4,3,3,3,3,3,3,3,4),(235.619449019235,236.469657471887,
237.337822045725,238.205986619563,239.074151193401,239.942315767239,240.810480341078,
241.678644914916,241.902634326414),.UNSPECIFIED.);
#1138=B_SPLINE_CURVE_WITH_KNOTS('',3,(#63578,#63579,#63580,#63581,#63582,
#63583,#63584,#63585,#63586,#63587,#63588,#63589,#63590,#63591),
 .UNSPECIFIED.,.F.,.F.,(4,1,1,1,1,1,1,1,1,1,1,4),(235.619449019235,235.887177564189,
236.386269775394,236.885361986599,237.384454197805,237.88354640901,238.88173083142,
239.87991525383,240.878099676241,241.377191887446,241.876284098651,241.902634326415),
 .UNSPECIFIED.);
#1139=B_SPLINE_CURVE_WITH_KNOTS('',3,(#63596,#63597,#63598,#63599,#63600,
#63601,#63602,#63603,#63604,#63605,#63606,#63607,#63608),.UNSPECIFIED.,
 .F.,.F.,(4,1,1,1,1,1,1,1,1,1,4),(229.336263712055,230.217421355688,230.716513566893,
231.215605778098,232.213790200509,232.712882411714,233.211974622919,233.711066834124,
234.210159045329,235.20834346774,235.619449019235),.UNSPECIFIED.);
#1140=B_SPLINE_CURVE_WITH_KNOTS('',3,(#63609,#63610,#63611,#63612,#63613,
#63614,#63615,#63616,#63617,#63618,#63619,#63620,#63621,#63622,#63623,#63624,
#63625,#63626,#63627,#63628,#63629,#63630,#63631,#63632,#63633),
 .UNSPECIFIED.,.F.,.F.,(4,3,3,3,3,3,3,3,4),(229.336263712055,230.02175290835,
230.889917482188,231.758082056027,232.626246629865,233.494411203703,234.362575777541,
235.230740351379,235.619449019235),.UNSPECIFIED.);
#1141=B_SPLINE_CURVE_WITH_KNOTS('',3,(#63638,#63639,#63640,#63641,#63642,
#63643,#63644,#63645,#63646,#63647,#63648,#63649,#63650,#63651),
 .UNSPECIFIED.,.F.,.F.,(4,1,1,1,1,1,1,1,1,1,1,4),(223.053078404876,223.230130398815,
223.72922261002,224.228314821226,225.226499243636,225.725591454841,226.224683666046,
226.723775877252,227.222868088457,228.221052510867,229.219236933277,229.336263712055),
 .UNSPECIFIED.);
#1142=B_SPLINE_CURVE_WITH_KNOTS('',3,(#63652,#63653,#63654,#63655,#63656,
#63657,#63658,#63659,#63660,#63661,#63662,#63663),.UNSPECIFIED.,.F.,.F.,
(4,1,1,1,1,1,1,1,1,4),(223.053078404876,223.40987228406,223.908964495265,
224.907148917675,225.905333340085,226.903517762496,227.402609973701,227.901702184906,
228.899886607316,229.336263712055),.UNSPECIFIED.);
#1143=B_SPLINE_CURVE_WITH_KNOTS('',3,(#63668,#63669,#63670,#63671,#63672,
#63673,#63674,#63675,#63676,#63677,#63678,#63679),.UNSPECIFIED.,.F.,.F.,
(4,1,1,1,1,1,1,1,1,4),(216.769893097696,217.241023864353,218.239208286764,
218.738300497969,219.237392709174,219.736484920379,220.235577131584,221.233761553995,
222.231945976405,223.053078404876),.UNSPECIFIED.);
#1144=B_SPLINE_CURVE_WITH_KNOTS('',3,(#63680,#63681,#63682,#63683,#63684,
#63685,#63686,#63687,#63688,#63689,#63690,#63691,#63692),.UNSPECIFIED.,
 .F.,.F.,(4,1,1,1,1,1,1,1,1,1,4),(216.769893097696,216.921673538392,217.919857960803,
218.918042383213,219.916226805623,220.415319016828,220.914411228034,221.912595650444,
222.411687861649,222.910780072854,223.053078404876),.UNSPECIFIED.);
#1145=B_SPLINE_CURVE_WITH_KNOTS('',3,(#63697,#63698,#63699,#63700,#63701,
#63702,#63703,#63704,#63705,#63706,#63707,#63708,#63709,#63710,#63711,#63712,
#63713,#63714,#63715,#63716,#63717,#63718,#63719,#63720,#63721),
 .UNSPECIFIED.,.F.,.F.,(4,3,3,3,3,3,3,3,4),(210.486707790517,211.292884830582,
212.16104940442,213.029213978258,213.897378552096,214.765543125934,215.633707699773,
216.501872273611,216.769893097696),.UNSPECIFIED.);
#1146=B_SPLINE_CURVE_WITH_KNOTS('',3,(#63722,#63723,#63724,#63725,#63726,
#63727,#63728,#63729,#63730,#63731,#63732,#63733,#63734),.UNSPECIFIED.,
 .F.,.F.,(4,1,1,1,1,1,1,1,1,1,4),(210.486707790517,210.93256700393,211.93075142634,
212.928935848751,213.428028059956,213.927120271161,214.925304693571,215.424396904777,
215.923489115982,216.422581327187,216.769893097696),.UNSPECIFIED.);
#1147=B_SPLINE_CURVE_WITH_KNOTS('',3,(#63739,#63740,#63741,#63742,#63743,
#63744,#63745,#63746,#63747,#63748,#63749,#63750,#63751,#63752,#63753,#63754,
#63755,#63756,#63757,#63758,#63759,#63760,#63761,#63762,#63763,#63764,#63765,
#63766),.UNSPECIFIED.,.F.,.F.,(4,3,3,3,3,3,3,3,3,4),(204.203522483337,204.347568239877,
205.215732813715,206.083897387553,206.952061961392,207.82022653523,208.688391109068,
209.556555682906,210.424720256744,210.486707790517),.UNSPECIFIED.);
#1148=B_SPLINE_CURVE_WITH_KNOTS('',3,(#63767,#63768,#63769,#63770,#63771,
#63772,#63773,#63774,#63775,#63776,#63777,#63778,#63779,#63780,#63781,#63782,
#63783,#63784,#63785,#63786,#63787,#63788,#63789,#63790,#63791),
 .UNSPECIFIED.,.F.,.F.,(4,3,3,3,3,3,3,3,4),(204.203522483337,204.844980267045,
205.713144840884,206.581309414722,207.44947398856,208.317638562398,209.185803136236,
210.053967710074,210.486707790517),.UNSPECIFIED.);
#1149=B_SPLINE_CURVE_WITH_KNOTS('',3,(#63796,#63797,#63798,#63799,#63800,
#63801,#63802,#63803,#63804,#63805,#63806),.UNSPECIFIED.,.F.,.F.,(4,1,1,
1,1,1,1,1,4),(197.920337176157,198.275519838556,199.273704260967,200.271888683377,
201.270073105787,202.268257528198,202.767349739403,203.266441950608,204.203522483337),
 .UNSPECIFIED.);
#1150=B_SPLINE_CURVE_WITH_KNOTS('',3,(#63807,#63808,#63809,#63810,#63811,
#63812,#63813,#63814,#63815,#63816,#63817,#63818,#63819,#63820),
 .UNSPECIFIED.,.F.,.F.,(4,1,1,1,1,1,1,1,1,1,1,4),(197.920337176158,197.956169512595,
198.954353935006,199.453446146211,199.952538357416,200.950722779826,201.449814991032,
201.948907202237,202.447999413442,202.947091624647,203.945276047057,204.203522483337),
 .UNSPECIFIED.);
#1151=B_SPLINE_CURVE_WITH_KNOTS('',3,(#63825,#63826,#63827,#63828,#63829,
#63830,#63831,#63832,#63833,#63834,#63835,#63836,#63837),.UNSPECIFIED.,
 .F.,.F.,(4,1,1,1,1,1,1,1,1,1,4),(191.637151868978,191.787321092889,192.286413304094,
192.785505515299,193.284597726505,194.282782148915,194.78187436012,195.280966571325,
196.279150993736,197.277335416146,197.920337176157),.UNSPECIFIED.);
#1152=B_SPLINE_CURVE_WITH_KNOTS('',3,(#63838,#63839,#63840,#63841,#63842,
#63843,#63844,#63845,#63846,#63847),.UNSPECIFIED.,.F.,.F.,(4,1,1,1,1,1,
1,4),(191.637151868978,191.967062978133,192.965247400543,193.963431822954,
194.961616245364,195.959800667775,196.957985090185,197.920337176158),
 .UNSPECIFIED.);
#1153=B_SPLINE_CURVE_WITH_KNOTS('',3,(#63852,#63853,#63854,#63855,#63856,
#63857,#63858,#63859,#63860,#63861,#63862,#63863),.UNSPECIFIED.,.F.,.F.,
(4,1,1,1,1,1,1,1,1,4),(185.353966561798,185.798214558427,186.297306769632,
187.295491192042,187.794583403248,188.293675614453,189.291860036863,190.290044459273,
191.288228881684,191.637151868978),.UNSPECIFIED.);
#1154=B_SPLINE_CURVE_WITH_KNOTS('',3,(#63864,#63865,#63866,#63867,#63868,
#63869,#63870,#63871,#63872,#63873,#63874,#63875,#63876),.UNSPECIFIED.,
 .F.,.F.,(4,1,1,1,1,1,1,1,1,1,4),(185.353966561798,185.977956443671,186.976140866081,
187.974325288492,188.473417499697,188.972509710902,189.471601922107,189.970694133312,
190.968878555723,191.467970766928,191.637151868978),.UNSPECIFIED.);
#1155=B_SPLINE_CURVE_WITH_KNOTS('',3,(#63881,#63882,#63883,#63884,#63885,
#63886,#63887,#63888,#63889,#63890,#63891,#63892,#63893,#63894,#63895,#63896,
#63897,#63898,#63899,#63900,#63901,#63902,#63903,#63904,#63905,#63906,#63907,
#63908),.UNSPECIFIED.,.F.,.F.,(4,3,3,3,3,3,3,3,3,4),(179.070781254619,179.170795598572,
180.03896017241,180.907124746249,181.775289320087,182.643453893925,183.511618467763,
184.379783041601,185.247947615439,185.353966561798),.UNSPECIFIED.);
#1156=B_SPLINE_CURVE_WITH_KNOTS('',3,(#63909,#63910,#63911,#63912,#63913,
#63914,#63915,#63916,#63917,#63918,#63919,#63920,#63921),.UNSPECIFIED.,
 .F.,.F.,(4,1,1,1,1,1,1,1,1,1,4),(179.070781254619,179.988849909209,180.987034331619,
181.486126542824,181.98521875403,182.484310965235,182.98340317644,183.98158759885,
184.480679810055,184.979772021261,185.353966561798),.UNSPECIFIED.);
#1157=B_SPLINE_CURVE_WITH_KNOTS('',3,(#63926,#63927,#63928,#63929,#63930,
#63931,#63932,#63933,#63934,#63935,#63936,#63937,#63938,#63939,#63940,#63941,
#63942,#63943,#63944,#63945,#63946,#63947,#63948,#63949,#63950),
 .UNSPECIFIED.,.F.,.F.,(4,3,3,3,3,3,3,3,4),(172.787595947439,173.093643581706,
173.961808155544,174.829972729382,175.69813730322,176.566301877058,177.434466450896,
178.302631024734,179.070781254619),.UNSPECIFIED.);
#1158=B_SPLINE_CURVE_WITH_KNOTS('',3,(#63951,#63952,#63953,#63954,#63955,
#63956,#63957,#63958,#63959,#63960,#63961,#63962,#63963,#63964),
 .UNSPECIFIED.,.F.,.F.,(4,1,1,1,1,1,1,1,1,1,1,4),(172.787595947439,173.001558952336,
173.999743374747,174.498835585952,174.997927797157,175.497020008362,175.996112219567,
176.994296641978,177.493388853183,177.992481064388,178.990665486798,179.070781254619),
 .UNSPECIFIED.);
#1159=B_SPLINE_CURVE_WITH_KNOTS('',3,(#63969,#63970,#63971,#63972,#63973,
#63974,#63975,#63976,#63977,#63978,#63979,#63980,#63981),.UNSPECIFIED.,
 .F.,.F.,(4,1,1,1,1,1,1,1,1,1,4),(166.50441064026,166.83271053263,167.331802743835,
168.329987166246,169.328171588656,170.326356011066,170.825448222271,171.324540433477,
171.823632644682,172.322724855887,172.787595947439),.UNSPECIFIED.);
#1160=B_SPLINE_CURVE_WITH_KNOTS('',3,(#63982,#63983,#63984,#63985,#63986,
#63987,#63988,#63989,#63990,#63991,#63992,#63993,#63994,#63995,#63996,#63997,
#63998,#63999,#64000,#64001,#64002,#64003,#64004,#64005,#64006,#64007,#64008,
#64009),.UNSPECIFIED.,.F.,.F.,(4,3,3,3,3,3,3,3,3,4),(166.50441064026,166.645739018169,
167.513903592007,168.382068165845,169.250232739683,170.118397313521,170.986561887359,
171.854726461198,172.722891035036,172.787595947439),.UNSPECIFIED.);
#1161=B_SPLINE_CURVE_WITH_KNOTS('',3,(#64014,#64015,#64016,#64017,#64018,
#64019,#64020,#64021,#64022,#64023,#64024,#64025,#64026),.UNSPECIFIED.,
 .F.,.F.,(4,1,1,1,1,1,1,1,1,1,4),(160.22122533308,160.344511786963,161.342696209373,
162.340880631783,163.339065054194,163.838157265399,164.337249476604,164.836341687809,
165.335433899014,166.333618321425,166.50441064026),.UNSPECIFIED.);
#1162=B_SPLINE_CURVE_WITH_KNOTS('',3,(#64027,#64028,#64029,#64030,#64031,
#64032,#64033,#64034,#64035,#64036,#64037,#64038,#64039),.UNSPECIFIED.,
 .F.,.F.,(4,1,1,1,1,1,1,1,1,1,4),(160.22122533308,160.524253672207,161.023345883412,
161.522438094617,162.021530305822,163.019714728233,163.518806939438,164.017899150643,
165.016083573053,166.014267995464,166.50441064026),.UNSPECIFIED.);
#1163=B_SPLINE_CURVE_WITH_KNOTS('',3,(#64044,#64045,#64046,#64047,#64048,
#64049,#64050,#64051,#64052,#64053,#64054,#64055,#64056),.UNSPECIFIED.,
 .F.,.F.,(4,1,1,1,1,1,1,1,1,1,4),(153.938040025901,154.3554052525,155.353589674911,
156.351774097321,156.850866308526,157.349958519732,157.849050730937,158.348142942142,
159.346327364552,159.845419575757,160.22122533308),.UNSPECIFIED.);
#1164=B_SPLINE_CURVE_WITH_KNOTS('',3,(#64057,#64058,#64059,#64060,#64061,
#64062,#64063,#64064,#64065,#64066,#64067,#64068,#64069),.UNSPECIFIED.,
 .F.,.F.,(4,1,1,1,1,1,1,1,1,1,4),(153.938040025901,154.036054926539,154.535147137745,
155.03423934895,156.03242377136,156.531515982565,157.030608193771,158.028792616181,
159.026977038591,160.025161461002,160.22122533308),.UNSPECIFIED.);
#1165=B_SPLINE_CURVE_WITH_KNOTS('',3,(#64074,#64075,#64076,#64077,#64078,
#64079,#64080,#64081,#64082,#64083,#64084,#64085,#64086),.UNSPECIFIED.,
 .F.,.F.,(4,1,1,1,1,1,1,1,1,1,4),(147.654854718721,148.366298718038,149.364483140449,
149.863575351654,150.362667562859,150.861759774064,151.360851985269,152.35903640768,
152.858128618885,153.35722083009,153.938040025901),.UNSPECIFIED.);
#1166=B_SPLINE_CURVE_WITH_KNOTS('',3,(#64087,#64088,#64089,#64090,#64091,
#64092,#64093,#64094,#64095,#64096,#64097,#64098),.UNSPECIFIED.,.F.,.F.,
(4,1,1,1,1,1,1,1,1,4),(147.654854718721,148.046948392077,149.045132814488,
149.544225025693,150.043317236898,151.041501659308,152.039686081719,153.037870504129,
153.536962715334,153.938040025901),.UNSPECIFIED.);
#1167=B_SPLINE_CURVE_WITH_KNOTS('',3,(#64103,#64104,#64105,#64106,#64107,
#64108,#64109,#64110,#64111,#64112,#64113,#64114,#64115,#64116),
 .UNSPECIFIED.,.F.,.F.,(4,1,1,1,1,1,1,1,1,1,1,4),(141.371669411541,141.379007761166,
142.377192183576,142.876284394781,143.375376605987,143.874468817192,144.373561028397,
145.371745450807,145.870837662012,146.369929873218,147.368114295628,147.654854718721),
 .UNSPECIFIED.);
#1168=B_SPLINE_CURVE_WITH_KNOTS('',3,(#64117,#64118,#64119,#64120,#64121,
#64122,#64123,#64124,#64125,#64126,#64127,#64128,#64129,#64130,#64131,#64132,
#64133,#64134,#64135,#64136,#64137,#64138,#64139,#64140,#64141,#64142,#64143,
#64144),.UNSPECIFIED.,.F.,.F.,(4,3,3,3,3,3,3,3,3,4),(141.371669411542,141.468966376864,
142.337130950702,143.20529552454,144.073460098378,144.941624672216,145.809789246055,
146.677953819893,147.546118393731,147.654854718721),.UNSPECIFIED.);
#1169=B_SPLINE_CURVE_WITH_KNOTS('',3,(#64149,#64150,#64151,#64152,#64153,
#64154,#64155,#64156,#64157,#64158,#64159,#64160,#64161),.UNSPECIFIED.,
 .F.,.F.,(4,1,1,1,1,1,1,1,1,1,4),(135.088484104362,135.389901226704,135.888993437909,
136.388085649114,136.887177860319,137.386270071524,138.384454493935,138.88354670514,
139.382638916345,140.380823338755,141.371669411541),.UNSPECIFIED.);
#1170=B_SPLINE_CURVE_WITH_KNOTS('',3,(#64162,#64163,#64164,#64165,#64166,
#64167,#64168,#64169,#64170,#64171,#64172,#64173,#64174),.UNSPECIFIED.,
 .F.,.F.,(4,1,1,1,1,1,1,1,1,1,4),(135.088484104362,135.569643111948,136.068735323153,
137.066919745563,138.065104167974,139.063288590384,139.562380801589,140.061473012794,
140.560565224,141.059657435205,141.371669411542),.UNSPECIFIED.);
#1171=B_SPLINE_CURVE_WITH_KNOTS('',3,(#64179,#64180,#64181,#64182,#64183,
#64184,#64185,#64186,#64187,#64188,#64189,#64190,#64191),.UNSPECIFIED.,
 .F.,.F.,(4,1,1,1,1,1,1,1,1,1,4),(128.805298797182,128.901702481036,129.400794692241,
129.899886903447,130.398979114652,131.397163537062,131.896255748267,132.395347959473,
133.393532381883,134.391716804293,135.088484104362),.UNSPECIFIED.);
#1172=B_SPLINE_CURVE_WITH_KNOTS('',3,(#64192,#64193,#64194,#64195,#64196,
#64197,#64198,#64199,#64200,#64201,#64202,#64203,#64204),.UNSPECIFIED.,
 .F.,.F.,(4,1,1,1,1,1,1,1,1,1,4),(128.805298797182,129.08144436628,130.079628788691,
131.077813211101,132.075997633511,132.575089844717,133.074182055922,133.573274267127,
134.072366478332,135.070550900743,135.088484104362),.UNSPECIFIED.);
#1173=B_SPLINE_CURVE_WITH_KNOTS('',3,(#64209,#64210,#64211,#64212,#64213,
#64214,#64215,#64216,#64217,#64218,#64219,#64220),.UNSPECIFIED.,.F.,.F.,
(4,1,1,1,1,1,1,1,1,4),(122.522113490003,122.912595946574,123.411688157779,
124.40987258019,124.908964791395,125.4080570026,126.40624142501,127.404425847421,
128.402610269831,128.805298797182),.UNSPECIFIED.);
#1174=B_SPLINE_CURVE_WITH_KNOTS('',3,(#64221,#64222,#64223,#64224,#64225,
#64226,#64227,#64228,#64229,#64230,#64231,#64232,#64233),.UNSPECIFIED.,
 .F.,.F.,(4,1,1,1,1,1,1,1,1,1,4),(122.522113490003,123.092337831818,124.090522254229,
125.088706676639,125.587798887844,126.086891099049,126.585983310255,127.08507552146,
128.08325994387,128.582352155075,128.805298797182),.UNSPECIFIED.);
#1175=B_SPLINE_CURVE_WITH_KNOTS('',3,(#64238,#64239,#64240,#64241,#64242,
#64243,#64244,#64245,#64246,#64247,#64248,#64249,#64250,#64251,#64252,#64253,
#64254,#64255,#64256,#64257,#64258,#64259,#64260,#64261,#64262),
 .UNSPECIFIED.,.F.,.F.,(4,3,3,3,3,3,3,3,4),(116.238928182823,116.662946282229,
117.531110856067,118.399275429905,119.267440003743,120.135604577582,121.00376915142,
121.871933725258,122.522113490003),.UNSPECIFIED.);
#1176=B_SPLINE_CURVE_WITH_KNOTS('',3,(#64263,#64264,#64265,#64266,#64267,
#64268,#64269,#64270,#64271,#64272,#64273,#64274,#64275),.UNSPECIFIED.,
 .F.,.F.,(4,1,1,1,1,1,1,1,1,1,4),(116.238928182823,117.103231297356,118.101415719766,
118.600507930972,119.099600142177,119.598692353382,120.097784564587,121.095968986998,
121.595061198203,122.094153409408,122.522113490003),.UNSPECIFIED.);
#1177=B_SPLINE_CURVE_WITH_KNOTS('',3,(#64280,#64281,#64282,#64283,#64284,
#64285,#64286,#64287,#64288,#64289,#64290,#64291,#64292,#64293,#64294,#64295,
#64296,#64297,#64298,#64299,#64300,#64301,#64302,#64303,#64304),
 .UNSPECIFIED.,.F.,.F.,(4,3,3,3,3,3,3,3,4),(109.955742875643,110.585794265362,
111.453958839201,112.322123413039,113.190287986877,114.058452560715,114.926617134553,
115.794781708391,116.238928182823),.UNSPECIFIED.);
#1178=B_SPLINE_CURVE_WITH_KNOTS('',3,(#64305,#64306,#64307,#64308,#64309,
#64310,#64311,#64312,#64313,#64314,#64315,#64316,#64317,#64318),
 .UNSPECIFIED.,.F.,.F.,(4,1,1,1,1,1,1,1,1,1,1,4),(109.955742875644,110.115940340484,
111.114124762894,111.613216974099,112.112309185304,112.611401396509,113.110493607715,
114.108678030125,114.60777024133,115.106862452535,116.105046874946,116.238928182823),
 .UNSPECIFIED.);
#1179=B_SPLINE_CURVE_WITH_KNOTS('',3,(#64323,#64324,#64325,#64326,#64327,
#64328,#64329,#64330,#64331,#64332,#64333,#64334,#64335,#64336,#64337,#64338,
#64339,#64340,#64341,#64342,#64343,#64344,#64345,#64346,#64347),
 .UNSPECIFIED.,.F.,.F.,(4,3,3,3,3,3,3,3,4),(103.672557568464,104.508642248496,
105.376806822334,106.244971396172,107.11313597001,107.981300543848,108.849465117686,
109.717629691524,109.955742875643),.UNSPECIFIED.);
#1180=B_SPLINE_CURVE_WITH_KNOTS('',3,(#64348,#64349,#64350,#64351,#64352,
#64353,#64354,#64355,#64356,#64357,#64358,#64359,#64360),.UNSPECIFIED.,
 .F.,.F.,(4,1,1,1,1,1,1,1,1,1,4),(103.672557568464,104.126833806021,104.625926017227,
105.125018228432,105.624110439637,106.123202650842,107.121387073252,107.620479284458,
108.119571495663,109.117755918073,109.955742875644),.UNSPECIFIED.);
#1181=B_SPLINE_CURVE_WITH_KNOTS('',3,(#64365,#64366,#64367,#64368,#64369,
#64370,#64371,#64372,#64373,#64374,#64375,#64376,#64377),.UNSPECIFIED.,
 .F.,.F.,(4,1,1,1,1,1,1,1,1,1,4),(97.3893722612843,97.4588931751099,98.4570775975203,
99.4552620199306,100.453446442341,100.952538653546,101.451630864751,101.950723075957,
102.449815287162,103.447999709572,103.672557568464),.UNSPECIFIED.);
#1182=B_SPLINE_CURVE_WITH_KNOTS('',3,(#64378,#64379,#64380,#64381,#64382,
#64383,#64384,#64385,#64386,#64387,#64388,#64389,#64390),.UNSPECIFIED.,
 .F.,.F.,(4,1,1,1,1,1,1,1,1,1,4),(97.3893722612844,97.638635060354,98.1377272715592,
98.6368194827644,99.1359116939696,100.13409611638,100.633188327585,101.13228053879,
102.130464961201,103.128649383611,103.672557568464),.UNSPECIFIED.);
#1183=B_SPLINE_CURVE_WITH_KNOTS('',3,(#64395,#64396,#64397,#64398,#64399,
#64400,#64401,#64402,#64403,#64404,#64405,#64406,#64407),.UNSPECIFIED.,
 .F.,.F.,(4,1,1,1,1,1,1,1,1,1,4),(91.1061869541047,91.4697866406478,92.4679710630581,
93.4661554854685,93.9652476966737,94.4643399078788,94.963432119084,95.4625243302892,
96.4607087526996,96.9598009639047,97.3893722612843),.UNSPECIFIED.);
#1184=B_SPLINE_CURVE_WITH_KNOTS('',3,(#64408,#64409,#64410,#64411,#64412,
#64413,#64414,#64415,#64416,#64417,#64418,#64419,#64420),.UNSPECIFIED.,
 .F.,.F.,(4,1,1,1,1,1,1,1,1,1,4),(91.1061869541048,91.1504363146867,91.6495285258919,
92.1486207370971,93.1468051595074,93.6458973707126,94.1449895819178,95.1431740043281,
96.1413584267385,97.1395428491489,97.3893722612844),.UNSPECIFIED.);
#1185=B_SPLINE_CURVE_WITH_KNOTS('',3,(#64425,#64426,#64427,#64428,#64429,
#64430,#64431,#64432,#64433,#64434,#64435,#64436,#64437),.UNSPECIFIED.,
 .F.,.F.,(4,1,1,1,1,1,1,1,1,1,4),(84.8230016469251,85.4806801061856,86.4788645285959,
86.9779567398011,87.4770489510063,87.9761411622115,88.4752333734167,89.473417795827,
89.9725100070322,90.4716022182374,91.1061869541047),.UNSPECIFIED.);
#1186=B_SPLINE_CURVE_WITH_KNOTS('',3,(#64438,#64439,#64440,#64441,#64442,
#64443,#64444,#64445,#64446,#64447,#64448,#64449),.UNSPECIFIED.,.F.,.F.,
(4,1,1,1,1,1,1,1,1,4),(84.8230016469252,85.1613297802245,86.1595142026349,
86.6586064138401,87.1576986250453,88.1558830474556,89.154067469866,90.1522518922763,
90.6513441034815,91.1061869541048),.UNSPECIFIED.);
#1187=B_SPLINE_CURVE_WITH_KNOTS('',3,(#64454,#64455,#64456,#64457,#64458,
#64459,#64460,#64461,#64462,#64463,#64464,#64465,#64466),.UNSPECIFIED.,
 .F.,.F.,(4,1,1,1,1,1,1,1,1,1,4),(78.5398163397456,79.4915735717234,79.9906657829286,
80.4897579941338,80.988850205339,81.4879424165442,82.4861268389545,82.9852190501597,
83.4843112613649,84.4824956837752,84.8230016469251),.UNSPECIFIED.);
#1188=B_SPLINE_CURVE_WITH_KNOTS('',3,(#64467,#64468,#64469,#64470,#64471,
#64472,#64473,#64474,#64475,#64476,#64477,#64478,#64479,#64480,#64481,#64482,
#64483,#64484,#64485,#64486,#64487,#64488,#64489,#64490,#64491),
 .UNSPECIFIED.,.F.,.F.,(4,3,3,3,3,3,3,3,4),(78.5398163397456,78.9611170605208,
79.8292816343589,80.697446208197,81.5656107820351,82.4337753558732,83.3019399297113,
84.1701045035494,84.8230016469252),.UNSPECIFIED.);
#1189=B_SPLINE_CURVE_WITH_KNOTS('',3,(#64496,#64497,#64498,#64499,#64500,
#64501,#64502,#64503,#64504,#64505,#64506,#64507,#64508,#64509),
 .UNSPECIFIED.,.F.,.F.,(4,1,1,1,1,1,1,1,1,1,1,4),(72.2566310325659,72.5042826148509,
73.0033748260561,73.5024670372613,74.0015592484665,74.5006514596716,75.498835882082,
75.9979280932872,76.4970203044924,77.4952047269027,78.4933891493131,78.5398163397456),
 .UNSPECIFIED.);
#1190=B_SPLINE_CURVE_WITH_KNOTS('',3,(#64510,#64511,#64512,#64513,#64514,
#64515,#64516,#64517,#64518,#64519,#64520,#64521,#64522),.UNSPECIFIED.,
 .F.,.F.,(4,1,1,1,1,1,1,1,1,1,4),(72.256631032566,72.684024500095,73.1831167113002,
74.1813011337106,75.1794855561209,76.1776699785313,76.6767621897365,77.1758544009417,
77.6749466121468,78.174038823352,78.5398163397456),.UNSPECIFIED.);
#1191=B_SPLINE_CURVE_WITH_KNOTS('',3,(#64527,#64528,#64529,#64530,#64531,
#64532,#64533,#64534,#64535,#64536,#64537,#64538,#64539),.UNSPECIFIED.,
 .F.,.F.,(4,1,1,1,1,1,1,1,1,1,4),(65.9734457253863,66.0160838691836,66.5151760803888,
67.0142682915939,67.5133605027991,68.5115449252095,69.0106371364147,69.5097293476198,
70.5079137700302,71.5060981924406,72.2566310325659),.UNSPECIFIED.);
#1192=B_SPLINE_CURVE_WITH_KNOTS('',3,(#64540,#64541,#64542,#64543,#64544,
#64545,#64546,#64547,#64548,#64549,#64550,#64551,#64552),.UNSPECIFIED.,
 .F.,.F.,(4,1,1,1,1,1,1,1,1,1,4),(65.9734457253865,66.1958257544277,67.194010176838,
68.1921945992484,69.1903790216588,69.689471232864,70.1885634440691,70.6876556552743,
71.1867478664795,72.1849322888899,72.256631032566),.UNSPECIFIED.);
#1193=B_SPLINE_CURVE_WITH_KNOTS('',3,(#64557,#64558,#64559,#64560,#64561,
#64562,#64563,#64564,#64565,#64566,#64567,#64568,#64569,#64570,#64571,#64572,
#64573,#64574,#64575,#64576,#64577,#64578,#64579,#64580,#64581),
 .UNSPECIFIED.,.F.,.F.,(4,3,3,3,3,3,3,3,4),(59.6902604182067,60.2322489827526,
61.1004135565907,61.9685781304288,62.8367427042669,63.704907278105,64.5730718519431,
65.4412364257812,65.9734457253863),.UNSPECIFIED.);
#1194=B_SPLINE_CURVE_WITH_KNOTS('',3,(#64582,#64583,#64584,#64585,#64586,
#64587,#64588,#64589,#64590,#64591,#64592,#64593,#64594),.UNSPECIFIED.,
 .F.,.F.,(4,1,1,1,1,1,1,1,1,1,4),(59.6902604182069,60.2067192199655,61.2049036423759,
62.2030880647862,62.7021802759914,63.2012724871966,63.7003646984018,64.199456909607,
65.1976413320173,65.6967335432225,65.9734457253865),.UNSPECIFIED.);
#1195=B_SPLINE_CURVE_WITH_KNOTS('',3,(#64599,#64600,#64601,#64602,#64603,
#64604,#64605,#64606,#64607,#64608,#64609,#64610,#64611,#64612,#64613,#64614,
#64615,#64616,#64617,#64618,#64619,#64620,#64621,#64622,#64623),
 .UNSPECIFIED.,.F.,.F.,(4,3,3,3,3,3,3,3,4),(53.4070751110271,54.1550969658859,
55.023261539724,55.8914261135621,56.7595906874002,57.6277552612383,58.4959198350764,
59.3640844089145,59.6902604182067),.UNSPECIFIED.);
#1196=B_SPLINE_CURVE_WITH_KNOTS('',3,(#64624,#64625,#64626,#64627,#64628,
#64629,#64630,#64631,#64632,#64633,#64634,#64635,#64636),.UNSPECIFIED.,
 .F.,.F.,(4,1,1,1,1,1,1,1,1,1,4),(53.4070751110272,54.2176126855034,55.2157971079137,
55.7148893191189,56.2139815303241,56.7130737415293,57.2121659527344,58.2103503751448,
58.70944258635,59.2085347975552,59.6902604182069),.UNSPECIFIED.);
#1197=B_SPLINE_CURVE_WITH_KNOTS('',3,(#64641,#64642,#64643,#64644,#64645,
#64646,#64647,#64648,#64649,#64650,#64651,#64652,#64653),.UNSPECIFIED.,
 .F.,.F.,(4,1,1,1,1,1,1,1,1,1,4),(47.1238898038476,47.5496720545919,48.0487642657971,
48.5478564770023,49.5460408994126,50.544225321823,51.5424097442334,52.0415019554385,
52.5405941666437,53.0396863778489,53.4070751110271),.UNSPECIFIED.);
#1198=B_SPLINE_CURVE_WITH_KNOTS('',3,(#64654,#64655,#64656,#64657,#64658,
#64659,#64660,#64661,#64662,#64663,#64664,#64665,#64666,#64667),
 .UNSPECIFIED.,.F.,.F.,(4,1,1,1,1,1,1,1,1,1,1,4),(47.1238898038477,47.2303217286308,
48.2285061510412,48.7275983622464,49.2266905734515,49.7257827846567,50.2248749958619,
51.2230594182723,51.7221516294775,52.2212438406826,53.219428263093,53.4070751110272),
 .UNSPECIFIED.);
#1199=B_SPLINE_CURVE_WITH_KNOTS('',3,(#64672,#64673,#64674,#64675,#64676,
#64677,#64678,#64679,#64680,#64681,#64682,#64683,#64684,#64685,#64686,#64687,
#64688,#64689,#64690,#64691,#64692,#64693,#64694,#64695,#64696),
 .UNSPECIFIED.,.F.,.F.,(4,3,3,3,3,3,3,3,4),(40.8407044966679,41.1326283583144,
42.0007929321525,42.8689575059906,43.7371220798287,44.6052866536668,45.4734512275049,
46.341615801343,47.1238898038476),.UNSPECIFIED.);
#1200=B_SPLINE_CURVE_WITH_KNOTS('',3,(#64697,#64698,#64699,#64700,#64701,
#64702,#64703,#64704,#64705,#64706,#64707,#64708,#64709),.UNSPECIFIED.,
 .F.,.F.,(4,1,1,1,1,1,1,1,1,1,4),(40.8407044966681,41.2412151941687,41.7403074053738,
42.239399616579,42.7384918277842,43.2375840389894,44.2357684613998,44.7348606726049,
45.2339528838101,46.2321373062205,47.1238898038477),.UNSPECIFIED.);
#1201=B_SPLINE_CURVE_WITH_KNOTS('',3,(#64714,#64715,#64716,#64717,#64718,
#64719,#64720,#64721,#64722,#64723,#64724,#64725,#64726),.UNSPECIFIED.,
 .F.,.F.,(4,1,1,1,1,1,1,1,1,1,4),(34.5575191894884,34.5732745632572,35.5714589856676,
36.569643408078,37.5678278304883,38.0669200416935,38.5660122528987,39.0651044641039,
39.564196675309,40.5623810977194,40.8407044966679),.UNSPECIFIED.);
#1202=B_SPLINE_CURVE_WITH_KNOTS('',3,(#64727,#64728,#64729,#64730,#64731,
#64732,#64733,#64734,#64735,#64736,#64737,#64738,#64739),.UNSPECIFIED.,
 .F.,.F.,(4,1,1,1,1,1,1,1,1,1,4),(34.5575191894885,34.7530164485013,35.2521086597065,
35.7512008709117,36.2502930821169,37.2484775045272,37.7475697157324,38.2466619269376,
39.2448463493479,40.2430307717583,40.8407044966681),.UNSPECIFIED.);
#1203=B_SPLINE_CURVE_WITH_KNOTS('',3,(#64744,#64745,#64746,#64747,#64748,
#64749,#64750,#64751,#64752,#64753,#64754,#64755,#64756),.UNSPECIFIED.,
 .F.,.F.,(4,1,1,1,1,1,1,1,1,1,4),(28.2743338823088,28.5841680287951,29.5823524512054,
30.5805368736158,31.079629084821,31.5787212960261,32.0778135072313,32.5769057184365,
33.5750901408469,34.074182352052,34.5575191894884),.UNSPECIFIED.);
#1204=B_SPLINE_CURVE_WITH_KNOTS('',3,(#64757,#64758,#64759,#64760,#64761,
#64762,#64763,#64764,#64765,#64766,#64767,#64768),.UNSPECIFIED.,.F.,.F.,
(4,1,1,1,1,1,1,1,1,4),(28.2743338823089,28.7639099140392,29.2630021252443,
30.2611865476547,30.7602787588599,31.2593709700651,32.2575553924754,33.2557398148858,
34.2539242372961,34.5575191894885),.UNSPECIFIED.);
#1205=B_SPLINE_CURVE_WITH_KNOTS('',3,(#64773,#64774,#64775,#64776,#64777,
#64778,#64779,#64780,#64781,#64782,#64783,#64784,#64785),.UNSPECIFIED.,
 .F.,.F.,(4,1,1,1,1,1,1,1,1,1,4),(21.9911485751292,22.5950614943329,23.5932459167433,
24.0923381279484,24.5914303391536,25.0905225503588,25.589614761564,26.5877991839743,
27.0868913951795,27.5859836063847,28.2743338823088),.UNSPECIFIED.);
#1206=B_SPLINE_CURVE_WITH_KNOTS('',3,(#64786,#64787,#64788,#64789,#64790,
#64791,#64792,#64793,#64794,#64795,#64796,#64797,#64798),.UNSPECIFIED.,
 .F.,.F.,(4,1,1,1,1,1,1,1,1,1,4),(21.9911485751293,22.2757111683718,23.2738955907822,
23.7729878019874,24.2720800131925,25.2702644356029,26.2684488580133,27.2666332804236,
27.7657254916288,28.264817702834,28.2743338823089),.UNSPECIFIED.);
#1207=B_SPLINE_CURVE_WITH_KNOTS('',3,(#64803,#64804,#64805,#64806,#64807,
#64808,#64809,#64810,#64811,#64812,#64813,#64814,#64815),.UNSPECIFIED.,
 .F.,.F.,(4,1,1,1,1,1,1,1,1,1,4),(15.7079632679496,16.6059549598707,17.1050471710759,
17.6041393822811,18.1032315934863,18.6023238046915,19.6005082271018,20.099600438307,
20.5986926495122,21.5968770719225,21.9911485751292),.UNSPECIFIED.);
#1208=B_SPLINE_CURVE_WITH_KNOTS('',3,(#64816,#64817,#64818,#64819,#64820,
#64821,#64822,#64823,#64824,#64825,#64826,#64827,#64828,#64829,#64830,#64831,
#64832,#64833,#64834,#64835,#64836,#64837,#64838,#64839,#64840),
 .UNSPECIFIED.,.F.,.F.,(4,3,3,3,3,3,3,3,4),(15.7079632679497,16.4532677441776,
17.3214323180157,18.1895968918538,19.0577614656919,19.92592603953,20.7940906133681,
21.6622551872062,21.9911485751293),.UNSPECIFIED.);
#1209=B_SPLINE_CURVE_WITH_KNOTS('',2,(#64849,#64850,#64851),
 .UNSPECIFIED.,.F.,.F.,(3,3),(0.,1.),.UNSPECIFIED.);
#1210=B_SPLINE_CURVE_WITH_KNOTS('',2,(#64855,#64856,#64857),
 .UNSPECIFIED.,.F.,.F.,(3,3),(0.,1.),.UNSPECIFIED.);
#1211=B_SPLINE_CURVE_WITH_KNOTS('',2,(#64866,#64867,#64868),
 .UNSPECIFIED.,.F.,.F.,(3,3),(0.,1.),.UNSPECIFIED.);
#1212=B_SPLINE_CURVE_WITH_KNOTS('',2,(#64871,#64872,#64873),
 .UNSPECIFIED.,.F.,.F.,(3,3),(0.,1.),.UNSPECIFIED.);
#1213=B_SPLINE_CURVE_WITH_KNOTS('',2,(#64881,#64882,#64883),
 .UNSPECIFIED.,.F.,.F.,(3,3),(0.,1.),.UNSPECIFIED.);
#1214=B_SPLINE_CURVE_WITH_KNOTS('',2,(#64886,#64887,#64888),
 .UNSPECIFIED.,.F.,.F.,(3,3),(0.,1.),.UNSPECIFIED.);
#1215=B_SPLINE_CURVE_WITH_KNOTS('',2,(#64896,#64897,#64898),
 .UNSPECIFIED.,.F.,.F.,(3,3),(0.,1.),.UNSPECIFIED.);
#1216=B_SPLINE_CURVE_WITH_KNOTS('',2,(#64901,#64902,#64903),
 .UNSPECIFIED.,.F.,.F.,(3,3),(0.,1.),.UNSPECIFIED.);
#1217=B_SPLINE_CURVE_WITH_KNOTS('',2,(#64911,#64912,#64913),
 .UNSPECIFIED.,.F.,.F.,(3,3),(0.,1.),.UNSPECIFIED.);
#1218=B_SPLINE_CURVE_WITH_KNOTS('',2,(#64916,#64917,#64918),
 .UNSPECIFIED.,.F.,.F.,(3,3),(0.,1.),.UNSPECIFIED.);
#1219=B_SPLINE_CURVE_WITH_KNOTS('',2,(#64926,#64927,#64928),
 .UNSPECIFIED.,.F.,.F.,(3,3),(0.,1.),.UNSPECIFIED.);
#1220=B_SPLINE_CURVE_WITH_KNOTS('',2,(#64931,#64932,#64933),
 .UNSPECIFIED.,.F.,.F.,(3,3),(0.,1.),.UNSPECIFIED.);
#1221=B_SPLINE_CURVE_WITH_KNOTS('',2,(#64941,#64942,#64943),
 .UNSPECIFIED.,.F.,.F.,(3,3),(0.,1.),.UNSPECIFIED.);
#1222=B_SPLINE_CURVE_WITH_KNOTS('',2,(#64946,#64947,#64948),
 .UNSPECIFIED.,.F.,.F.,(3,3),(0.,1.),.UNSPECIFIED.);
#1223=B_SPLINE_CURVE_WITH_KNOTS('',2,(#64956,#64957,#64958),
 .UNSPECIFIED.,.F.,.F.,(3,3),(0.,1.),.UNSPECIFIED.);
#1224=B_SPLINE_CURVE_WITH_KNOTS('',2,(#64961,#64962,#64963),
 .UNSPECIFIED.,.F.,.F.,(3,3),(0.,1.),.UNSPECIFIED.);
#1225=B_SPLINE_CURVE_WITH_KNOTS('',2,(#64970,#64971,#64972),
 .UNSPECIFIED.,.F.,.F.,(3,3),(0.,1.),.UNSPECIFIED.);
#1226=B_SPLINE_CURVE_WITH_KNOTS('',2,(#64973,#64974,#64975),
 .UNSPECIFIED.,.F.,.F.,(3,3),(0.,1.),.UNSPECIFIED.);
#1227=B_SPLINE_CURVE_WITH_KNOTS('',2,(#64984,#64985,#64986),
 .UNSPECIFIED.,.F.,.F.,(3,3),(0.,1.),.UNSPECIFIED.);
#1228=B_SPLINE_CURVE_WITH_KNOTS('',2,(#64990,#64991,#64992),
 .UNSPECIFIED.,.F.,.F.,(3,3),(0.,1.),.UNSPECIFIED.);
#1229=B_SPLINE_CURVE_WITH_KNOTS('',2,(#65001,#65002,#65003),
 .UNSPECIFIED.,.F.,.F.,(3,3),(0.,1.),.UNSPECIFIED.);
#1230=B_SPLINE_CURVE_WITH_KNOTS('',2,(#65006,#65007,#65008),
 .UNSPECIFIED.,.F.,.F.,(3,3),(0.,1.),.UNSPECIFIED.);
#1231=B_SPLINE_CURVE_WITH_KNOTS('',2,(#65016,#65017,#65018),
 .UNSPECIFIED.,.F.,.F.,(3,3),(0.,1.),.UNSPECIFIED.);
#1232=B_SPLINE_CURVE_WITH_KNOTS('',2,(#65021,#65022,#65023),
 .UNSPECIFIED.,.F.,.F.,(3,3),(0.,1.),.UNSPECIFIED.);
#1233=B_SPLINE_CURVE_WITH_KNOTS('',2,(#65031,#65032,#65033),
 .UNSPECIFIED.,.F.,.F.,(3,3),(0.,1.),.UNSPECIFIED.);
#1234=B_SPLINE_CURVE_WITH_KNOTS('',2,(#65036,#65037,#65038),
 .UNSPECIFIED.,.F.,.F.,(3,3),(0.,1.),.UNSPECIFIED.);
#1235=B_SPLINE_CURVE_WITH_KNOTS('',2,(#65046,#65047,#65048),
 .UNSPECIFIED.,.F.,.F.,(3,3),(0.,1.),.UNSPECIFIED.);
#1236=B_SPLINE_CURVE_WITH_KNOTS('',2,(#65051,#65052,#65053),
 .UNSPECIFIED.,.F.,.F.,(3,3),(0.,1.),.UNSPECIFIED.);
#1237=B_SPLINE_CURVE_WITH_KNOTS('',2,(#65061,#65062,#65063),
 .UNSPECIFIED.,.F.,.F.,(3,3),(0.,1.),.UNSPECIFIED.);
#1238=B_SPLINE_CURVE_WITH_KNOTS('',2,(#65066,#65067,#65068),
 .UNSPECIFIED.,.F.,.F.,(3,3),(0.,1.),.UNSPECIFIED.);
#1239=B_SPLINE_CURVE_WITH_KNOTS('',2,(#65076,#65077,#65078),
 .UNSPECIFIED.,.F.,.F.,(3,3),(0.,1.),.UNSPECIFIED.);
#1240=B_SPLINE_CURVE_WITH_KNOTS('',2,(#65081,#65082,#65083),
 .UNSPECIFIED.,.F.,.F.,(3,3),(0.,1.),.UNSPECIFIED.);
#1241=B_SPLINE_CURVE_WITH_KNOTS('',2,(#65090,#65091,#65092),
 .UNSPECIFIED.,.F.,.F.,(3,3),(0.,1.),.UNSPECIFIED.);
#1242=B_SPLINE_CURVE_WITH_KNOTS('',2,(#65093,#65094,#65095),
 .UNSPECIFIED.,.F.,.F.,(3,3),(0.,1.),.UNSPECIFIED.);
#1243=B_SPLINE_CURVE_WITH_KNOTS('',2,(#65104,#65105,#65106),
 .UNSPECIFIED.,.F.,.F.,(3,3),(0.,1.),.UNSPECIFIED.);
#1244=B_SPLINE_CURVE_WITH_KNOTS('',2,(#65110,#65111,#65112),
 .UNSPECIFIED.,.F.,.F.,(3,3),(0.,1.),.UNSPECIFIED.);
#1245=B_SPLINE_CURVE_WITH_KNOTS('',2,(#65121,#65122,#65123),
 .UNSPECIFIED.,.F.,.F.,(3,3),(0.,1.),.UNSPECIFIED.);
#1246=B_SPLINE_CURVE_WITH_KNOTS('',2,(#65126,#65127,#65128),
 .UNSPECIFIED.,.F.,.F.,(3,3),(0.,1.),.UNSPECIFIED.);
#1247=B_SPLINE_CURVE_WITH_KNOTS('',2,(#65136,#65137,#65138),
 .UNSPECIFIED.,.F.,.F.,(3,3),(0.,1.),.UNSPECIFIED.);
#1248=B_SPLINE_CURVE_WITH_KNOTS('',2,(#65141,#65142,#65143),
 .UNSPECIFIED.,.F.,.F.,(3,3),(0.,1.),.UNSPECIFIED.);
#1249=B_SPLINE_CURVE_WITH_KNOTS('',2,(#65151,#65152,#65153),
 .UNSPECIFIED.,.F.,.F.,(3,3),(0.,1.),.UNSPECIFIED.);
#1250=B_SPLINE_CURVE_WITH_KNOTS('',2,(#65156,#65157,#65158),
 .UNSPECIFIED.,.F.,.F.,(3,3),(0.,1.),.UNSPECIFIED.);
#1251=B_SPLINE_CURVE_WITH_KNOTS('',2,(#65166,#65167,#65168),
 .UNSPECIFIED.,.F.,.F.,(3,3),(0.,1.),.UNSPECIFIED.);
#1252=B_SPLINE_CURVE_WITH_KNOTS('',2,(#65171,#65172,#65173),
 .UNSPECIFIED.,.F.,.F.,(3,3),(0.,1.),.UNSPECIFIED.);
#1253=B_SPLINE_CURVE_WITH_KNOTS('',2,(#65181,#65182,#65183),
 .UNSPECIFIED.,.F.,.F.,(3,3),(0.,1.),.UNSPECIFIED.);
#1254=B_SPLINE_CURVE_WITH_KNOTS('',2,(#65186,#65187,#65188),
 .UNSPECIFIED.,.F.,.F.,(3,3),(0.,1.),.UNSPECIFIED.);
#1255=B_SPLINE_CURVE_WITH_KNOTS('',2,(#65196,#65197,#65198),
 .UNSPECIFIED.,.F.,.F.,(3,3),(0.,1.),.UNSPECIFIED.);
#1256=B_SPLINE_CURVE_WITH_KNOTS('',2,(#65201,#65202,#65203),
 .UNSPECIFIED.,.F.,.F.,(3,3),(0.,1.),.UNSPECIFIED.);
#1257=B_SPLINE_CURVE_WITH_KNOTS('',2,(#65211,#65212,#65213),
 .UNSPECIFIED.,.F.,.F.,(3,3),(0.,1.),.UNSPECIFIED.);
#1258=B_SPLINE_CURVE_WITH_KNOTS('',2,(#65216,#65217,#65218),
 .UNSPECIFIED.,.F.,.F.,(3,3),(0.,1.),.UNSPECIFIED.);
#1259=B_SPLINE_CURVE_WITH_KNOTS('',2,(#65226,#65227,#65228),
 .UNSPECIFIED.,.F.,.F.,(3,3),(0.,1.),.UNSPECIFIED.);
#1260=B_SPLINE_CURVE_WITH_KNOTS('',2,(#65231,#65232,#65233),
 .UNSPECIFIED.,.F.,.F.,(3,3),(0.,1.),.UNSPECIFIED.);
#1261=B_SPLINE_CURVE_WITH_KNOTS('',2,(#65241,#65242,#65243),
 .UNSPECIFIED.,.F.,.F.,(3,3),(0.,1.),.UNSPECIFIED.);
#1262=B_SPLINE_CURVE_WITH_KNOTS('',2,(#65246,#65247,#65248),
 .UNSPECIFIED.,.F.,.F.,(3,3),(0.,1.),.UNSPECIFIED.);
#1263=B_SPLINE_CURVE_WITH_KNOTS('',2,(#65256,#65257,#65258),
 .UNSPECIFIED.,.F.,.F.,(3,3),(0.,1.),.UNSPECIFIED.);
#1264=B_SPLINE_CURVE_WITH_KNOTS('',2,(#65261,#65262,#65263),
 .UNSPECIFIED.,.F.,.F.,(3,3),(0.,1.),.UNSPECIFIED.);
#1265=B_SPLINE_CURVE_WITH_KNOTS('',2,(#65271,#65272,#65273),
 .UNSPECIFIED.,.F.,.F.,(3,3),(0.,1.),.UNSPECIFIED.);
#1266=B_SPLINE_CURVE_WITH_KNOTS('',2,(#65276,#65277,#65278),
 .UNSPECIFIED.,.F.,.F.,(3,3),(0.,1.),.UNSPECIFIED.);
#1267=B_SPLINE_CURVE_WITH_KNOTS('',2,(#65286,#65287,#65288),
 .UNSPECIFIED.,.F.,.F.,(3,3),(0.,1.),.UNSPECIFIED.);
#1268=B_SPLINE_CURVE_WITH_KNOTS('',2,(#65291,#65292,#65293),
 .UNSPECIFIED.,.F.,.F.,(3,3),(0.,1.),.UNSPECIFIED.);
#1269=B_SPLINE_CURVE_WITH_KNOTS('',2,(#65301,#65302,#65303),
 .UNSPECIFIED.,.F.,.F.,(3,3),(0.,1.),.UNSPECIFIED.);
#1270=B_SPLINE_CURVE_WITH_KNOTS('',2,(#65306,#65307,#65308),
 .UNSPECIFIED.,.F.,.F.,(3,3),(0.,1.),.UNSPECIFIED.);
#1271=B_SPLINE_CURVE_WITH_KNOTS('',2,(#65316,#65317,#65318),
 .UNSPECIFIED.,.F.,.F.,(3,3),(0.,1.),.UNSPECIFIED.);
#1272=B_SPLINE_CURVE_WITH_KNOTS('',2,(#65321,#65322,#65323),
 .UNSPECIFIED.,.F.,.F.,(3,3),(0.,1.),.UNSPECIFIED.);
#1273=B_SPLINE_CURVE_WITH_KNOTS('',2,(#65330,#65331,#65332),
 .UNSPECIFIED.,.F.,.F.,(3,3),(0.,1.),.UNSPECIFIED.);
#1274=B_SPLINE_CURVE_WITH_KNOTS('',2,(#65333,#65334,#65335),
 .UNSPECIFIED.,.F.,.F.,(3,3),(0.,1.),.UNSPECIFIED.);
#1275=B_SPLINE_CURVE_WITH_KNOTS('',2,(#65370,#65371,#65372),
 .UNSPECIFIED.,.F.,.F.,(3,3),(0.,1.),.UNSPECIFIED.);
#1276=B_SPLINE_CURVE_WITH_KNOTS('',2,(#65376,#65377,#65378),
 .UNSPECIFIED.,.F.,.F.,(3,3),(0.,1.),.UNSPECIFIED.);
#1277=B_SPLINE_CURVE_WITH_KNOTS('',2,(#65387,#65388,#65389),
 .UNSPECIFIED.,.F.,.F.,(3,3),(0.,1.),.UNSPECIFIED.);
#1278=B_SPLINE_CURVE_WITH_KNOTS('',2,(#65392,#65393,#65394),
 .UNSPECIFIED.,.F.,.F.,(3,3),(0.,1.),.UNSPECIFIED.);
#1279=B_SPLINE_CURVE_WITH_KNOTS('',2,(#65402,#65403,#65404),
 .UNSPECIFIED.,.F.,.F.,(3,3),(0.,1.),.UNSPECIFIED.);
#1280=B_SPLINE_CURVE_WITH_KNOTS('',2,(#65407,#65408,#65409),
 .UNSPECIFIED.,.F.,.F.,(3,3),(0.,1.),.UNSPECIFIED.);
#1281=B_SPLINE_CURVE_WITH_KNOTS('',2,(#65417,#65418,#65419),
 .UNSPECIFIED.,.F.,.F.,(3,3),(0.,1.),.UNSPECIFIED.);
#1282=B_SPLINE_CURVE_WITH_KNOTS('',2,(#65422,#65423,#65424),
 .UNSPECIFIED.,.F.,.F.,(3,3),(0.,1.),.UNSPECIFIED.);
#1283=B_SPLINE_CURVE_WITH_KNOTS('',2,(#65432,#65433,#65434),
 .UNSPECIFIED.,.F.,.F.,(3,3),(0.,1.),.UNSPECIFIED.);
#1284=B_SPLINE_CURVE_WITH_KNOTS('',2,(#65437,#65438,#65439),
 .UNSPECIFIED.,.F.,.F.,(3,3),(0.,1.),.UNSPECIFIED.);
#1285=B_SPLINE_CURVE_WITH_KNOTS('',2,(#65447,#65448,#65449),
 .UNSPECIFIED.,.F.,.F.,(3,3),(0.,1.),.UNSPECIFIED.);
#1286=B_SPLINE_CURVE_WITH_KNOTS('',2,(#65452,#65453,#65454),
 .UNSPECIFIED.,.F.,.F.,(3,3),(0.,1.),.UNSPECIFIED.);
#1287=B_SPLINE_CURVE_WITH_KNOTS('',2,(#65462,#65463,#65464),
 .UNSPECIFIED.,.F.,.F.,(3,3),(0.,1.),.UNSPECIFIED.);
#1288=B_SPLINE_CURVE_WITH_KNOTS('',2,(#65467,#65468,#65469),
 .UNSPECIFIED.,.F.,.F.,(3,3),(0.,1.),.UNSPECIFIED.);
#1289=B_SPLINE_CURVE_WITH_KNOTS('',2,(#65477,#65478,#65479),
 .UNSPECIFIED.,.F.,.F.,(3,3),(0.,1.),.UNSPECIFIED.);
#1290=B_SPLINE_CURVE_WITH_KNOTS('',2,(#65482,#65483,#65484),
 .UNSPECIFIED.,.F.,.F.,(3,3),(0.,1.),.UNSPECIFIED.);
#1291=B_SPLINE_CURVE_WITH_KNOTS('',2,(#65491,#65492,#65493),
 .UNSPECIFIED.,.F.,.F.,(3,3),(0.,1.),.UNSPECIFIED.);
#1292=B_SPLINE_CURVE_WITH_KNOTS('',2,(#65494,#65495,#65496),
 .UNSPECIFIED.,.F.,.F.,(3,3),(0.,1.),.UNSPECIFIED.);
#1293=B_SPLINE_CURVE_WITH_KNOTS('',2,(#65505,#65506,#65507),
 .UNSPECIFIED.,.F.,.F.,(3,3),(0.,1.),.UNSPECIFIED.);
#1294=B_SPLINE_CURVE_WITH_KNOTS('',2,(#65511,#65512,#65513),
 .UNSPECIFIED.,.F.,.F.,(3,3),(0.,1.),.UNSPECIFIED.);
#1295=B_SPLINE_CURVE_WITH_KNOTS('',2,(#65522,#65523,#65524),
 .UNSPECIFIED.,.F.,.F.,(3,3),(0.,1.),.UNSPECIFIED.);
#1296=B_SPLINE_CURVE_WITH_KNOTS('',2,(#65527,#65528,#65529),
 .UNSPECIFIED.,.F.,.F.,(3,3),(0.,1.),.UNSPECIFIED.);
#1297=B_SPLINE_CURVE_WITH_KNOTS('',2,(#65537,#65538,#65539),
 .UNSPECIFIED.,.F.,.F.,(3,3),(0.,1.),.UNSPECIFIED.);
#1298=B_SPLINE_CURVE_WITH_KNOTS('',2,(#65542,#65543,#65544),
 .UNSPECIFIED.,.F.,.F.,(3,3),(0.,1.),.UNSPECIFIED.);
#1299=B_SPLINE_CURVE_WITH_KNOTS('',2,(#65552,#65553,#65554),
 .UNSPECIFIED.,.F.,.F.,(3,3),(0.,1.),.UNSPECIFIED.);
#1300=B_SPLINE_CURVE_WITH_KNOTS('',2,(#65557,#65558,#65559),
 .UNSPECIFIED.,.F.,.F.,(3,3),(0.,1.),.UNSPECIFIED.);
#1301=B_SPLINE_CURVE_WITH_KNOTS('',2,(#65567,#65568,#65569),
 .UNSPECIFIED.,.F.,.F.,(3,3),(0.,1.),.UNSPECIFIED.);
#1302=B_SPLINE_CURVE_WITH_KNOTS('',2,(#65572,#65573,#65574),
 .UNSPECIFIED.,.F.,.F.,(3,3),(0.,1.),.UNSPECIFIED.);
#1303=B_SPLINE_CURVE_WITH_KNOTS('',2,(#65582,#65583,#65584),
 .UNSPECIFIED.,.F.,.F.,(3,3),(0.,1.),.UNSPECIFIED.);
#1304=B_SPLINE_CURVE_WITH_KNOTS('',2,(#65587,#65588,#65589),
 .UNSPECIFIED.,.F.,.F.,(3,3),(0.,1.),.UNSPECIFIED.);
#1305=B_SPLINE_CURVE_WITH_KNOTS('',2,(#65597,#65598,#65599),
 .UNSPECIFIED.,.F.,.F.,(3,3),(0.,1.),.UNSPECIFIED.);
#1306=B_SPLINE_CURVE_WITH_KNOTS('',2,(#65602,#65603,#65604),
 .UNSPECIFIED.,.F.,.F.,(3,3),(0.,1.),.UNSPECIFIED.);
#1307=B_SPLINE_CURVE_WITH_KNOTS('',2,(#65611,#65612,#65613),
 .UNSPECIFIED.,.F.,.F.,(3,3),(0.,1.),.UNSPECIFIED.);
#1308=B_SPLINE_CURVE_WITH_KNOTS('',2,(#65614,#65615,#65616),
 .UNSPECIFIED.,.F.,.F.,(3,3),(0.,1.),.UNSPECIFIED.);
#1309=B_SPLINE_CURVE_WITH_KNOTS('',2,(#65625,#65626,#65627),
 .UNSPECIFIED.,.F.,.F.,(3,3),(0.,1.),.UNSPECIFIED.);
#1310=B_SPLINE_CURVE_WITH_KNOTS('',2,(#65631,#65632,#65633),
 .UNSPECIFIED.,.F.,.F.,(3,3),(0.,1.),.UNSPECIFIED.);
#1311=B_SPLINE_CURVE_WITH_KNOTS('',2,(#65642,#65643,#65644),
 .UNSPECIFIED.,.F.,.F.,(3,3),(0.,1.),.UNSPECIFIED.);
#1312=B_SPLINE_CURVE_WITH_KNOTS('',2,(#65647,#65648,#65649),
 .UNSPECIFIED.,.F.,.F.,(3,3),(0.,1.),.UNSPECIFIED.);
#1313=B_SPLINE_CURVE_WITH_KNOTS('',2,(#65657,#65658,#65659),
 .UNSPECIFIED.,.F.,.F.,(3,3),(0.,1.),.UNSPECIFIED.);
#1314=B_SPLINE_CURVE_WITH_KNOTS('',2,(#65662,#65663,#65664),
 .UNSPECIFIED.,.F.,.F.,(3,3),(0.,1.),.UNSPECIFIED.);
#1315=B_SPLINE_CURVE_WITH_KNOTS('',2,(#65672,#65673,#65674),
 .UNSPECIFIED.,.F.,.F.,(3,3),(0.,1.),.UNSPECIFIED.);
#1316=B_SPLINE_CURVE_WITH_KNOTS('',2,(#65677,#65678,#65679),
 .UNSPECIFIED.,.F.,.F.,(3,3),(0.,1.),.UNSPECIFIED.);
#1317=B_SPLINE_CURVE_WITH_KNOTS('',2,(#65687,#65688,#65689),
 .UNSPECIFIED.,.F.,.F.,(3,3),(0.,1.),.UNSPECIFIED.);
#1318=B_SPLINE_CURVE_WITH_KNOTS('',2,(#65692,#65693,#65694),
 .UNSPECIFIED.,.F.,.F.,(3,3),(0.,1.),.UNSPECIFIED.);
#1319=B_SPLINE_CURVE_WITH_KNOTS('',2,(#65702,#65703,#65704),
 .UNSPECIFIED.,.F.,.F.,(3,3),(0.,1.),.UNSPECIFIED.);
#1320=B_SPLINE_CURVE_WITH_KNOTS('',2,(#65707,#65708,#65709),
 .UNSPECIFIED.,.F.,.F.,(3,3),(0.,1.),.UNSPECIFIED.);
#1321=B_SPLINE_CURVE_WITH_KNOTS('',2,(#65717,#65718,#65719),
 .UNSPECIFIED.,.F.,.F.,(3,3),(0.,1.),.UNSPECIFIED.);
#1322=B_SPLINE_CURVE_WITH_KNOTS('',2,(#65722,#65723,#65724),
 .UNSPECIFIED.,.F.,.F.,(3,3),(0.,1.),.UNSPECIFIED.);
#1323=B_SPLINE_CURVE_WITH_KNOTS('',2,(#65732,#65733,#65734),
 .UNSPECIFIED.,.F.,.F.,(3,3),(0.,1.),.UNSPECIFIED.);
#1324=B_SPLINE_CURVE_WITH_KNOTS('',2,(#65737,#65738,#65739),
 .UNSPECIFIED.,.F.,.F.,(3,3),(0.,1.),.UNSPECIFIED.);
#1325=B_SPLINE_CURVE_WITH_KNOTS('',2,(#65747,#65748,#65749),
 .UNSPECIFIED.,.F.,.F.,(3,3),(0.,1.),.UNSPECIFIED.);
#1326=B_SPLINE_CURVE_WITH_KNOTS('',2,(#65752,#65753,#65754),
 .UNSPECIFIED.,.F.,.F.,(3,3),(0.,1.),.UNSPECIFIED.);
#1327=B_SPLINE_CURVE_WITH_KNOTS('',2,(#65762,#65763,#65764),
 .UNSPECIFIED.,.F.,.F.,(3,3),(0.,1.),.UNSPECIFIED.);
#1328=B_SPLINE_CURVE_WITH_KNOTS('',2,(#65767,#65768,#65769),
 .UNSPECIFIED.,.F.,.F.,(3,3),(0.,1.),.UNSPECIFIED.);
#1329=B_SPLINE_CURVE_WITH_KNOTS('',2,(#65777,#65778,#65779),
 .UNSPECIFIED.,.F.,.F.,(3,3),(0.,1.),.UNSPECIFIED.);
#1330=B_SPLINE_CURVE_WITH_KNOTS('',2,(#65782,#65783,#65784),
 .UNSPECIFIED.,.F.,.F.,(3,3),(0.,1.),.UNSPECIFIED.);
#1331=B_SPLINE_CURVE_WITH_KNOTS('',2,(#65792,#65793,#65794),
 .UNSPECIFIED.,.F.,.F.,(3,3),(0.,1.),.UNSPECIFIED.);
#1332=B_SPLINE_CURVE_WITH_KNOTS('',2,(#65797,#65798,#65799),
 .UNSPECIFIED.,.F.,.F.,(3,3),(0.,1.),.UNSPECIFIED.);
#1333=B_SPLINE_CURVE_WITH_KNOTS('',2,(#65807,#65808,#65809),
 .UNSPECIFIED.,.F.,.F.,(3,3),(0.,1.),.UNSPECIFIED.);
#1334=B_SPLINE_CURVE_WITH_KNOTS('',2,(#65812,#65813,#65814),
 .UNSPECIFIED.,.F.,.F.,(3,3),(0.,1.),.UNSPECIFIED.);
#1335=B_SPLINE_CURVE_WITH_KNOTS('',2,(#65822,#65823,#65824),
 .UNSPECIFIED.,.F.,.F.,(3,3),(0.,1.),.UNSPECIFIED.);
#1336=B_SPLINE_CURVE_WITH_KNOTS('',2,(#65827,#65828,#65829),
 .UNSPECIFIED.,.F.,.F.,(3,3),(0.,1.),.UNSPECIFIED.);
#1337=B_SPLINE_CURVE_WITH_KNOTS('',2,(#65837,#65838,#65839),
 .UNSPECIFIED.,.F.,.F.,(3,3),(0.,1.),.UNSPECIFIED.);
#1338=B_SPLINE_CURVE_WITH_KNOTS('',2,(#65842,#65843,#65844),
 .UNSPECIFIED.,.F.,.F.,(3,3),(0.,1.),.UNSPECIFIED.);
#1339=B_SPLINE_CURVE_WITH_KNOTS('',2,(#65851,#65852,#65853),
 .UNSPECIFIED.,.F.,.F.,(3,3),(0.,1.),.UNSPECIFIED.);
#1340=B_SPLINE_CURVE_WITH_KNOTS('',2,(#65854,#65855,#65856),
 .UNSPECIFIED.,.F.,.F.,(3,3),(0.,1.),.UNSPECIFIED.);
#1341=B_SPLINE_CURVE_WITH_KNOTS('',3,(#65863,#65864,#65865,#65866,#65867,
#65868,#65869,#65870,#65871,#65872,#65873,#65874,#65875,#65876,#65877,#65878,
#65879,#65880,#65881,#65882,#65883,#65884,#65885,#65886,#65887,#65888,#65889,
#65890,#65891,#65892,#65893,#65894,#65895,#65896,#65897,#65898,#65899,#65900,
#65901,#65902,#65903,#65904,#65905,#65906,#65907,#65908,#65909,#65910,#65911,
#65912,#65913,#65914,#65915,#65916,#65917,#65918,#65919,#65920,#65921,#65922,
#65923,#65924,#65925,#65926,#65927,#65928,#65929,#65930,#65931,#65932,#65933,
#65934,#65935),.UNSPECIFIED.,.F.,.F.,(4,3,3,3,3,3,3,3,3,3,3,3,3,3,3,3,3,
3,3,3,3,3,3,3,4),(-1.53373699248747,-1.47998259246901,-1.39266174048304,
-1.36022791806051,-1.33444301006683,-1.23257109729599,-1.16841771032442,
-1.14505420412193,-1.13069918452514,-1.02732007613362,-0.923657890223372,
-0.893957590402323,-0.872515155528604,-0.767248151591737,-0.672999266808395,
-0.620634679909978,-0.597605365315507,-0.48985421101852,-0.390252612458368,
-0.338746494543295,-0.311332063159986,-0.288956015137301,-0.179727021085193,
-0.0696390475340457,0.),.UNSPECIFIED.);
#1342=B_SPLINE_CURVE_WITH_KNOTS('',3,(#65940,#65941,#65942,#65943,#65944,
#65945,#65946,#65947,#65948,#65949,#65950,#65951,#65952,#65953,#65954,#65955,
#65956,#65957,#65958,#65959,#65960,#65961,#65962,#65963,#65964,#65965,#65966,
#65967,#65968,#65969,#65970,#65971,#65972,#65973,#65974,#65975,#65976,#65977,
#65978,#65979,#65980,#65981,#65982,#65983,#65984,#65985,#65986,#65987,#65988,
#65989,#65990,#65991,#65992,#65993,#65994,#65995,#65996,#65997,#65998,#65999,
#66000,#66001,#66002,#66003,#66004,#66005,#66006,#66007,#66008,#66009,#66010,
#66011,#66012,#66013,#66014,#66015),.UNSPECIFIED.,.F.,.F.,(4,3,3,3,3,3,
3,3,3,3,3,3,3,3,3,3,3,3,3,3,3,3,3,3,3,4),(-1.52870610664506,-1.46664447796478,
-1.3700636136821,-1.32344222320383,-1.2949393095723,-1.18763016520319,-1.12106166313349,
-1.09619363797947,-1.08032102083408,-0.973278106620055,-0.867444501613014,
-0.829257794374334,-0.806280268847329,-0.706769958895532,-0.616721647432219,
-0.570817503182251,-0.543589420844949,-0.522682905689514,-0.420869349973873,
-0.346576713042279,-0.298085656104414,-0.273538172108159,-0.252565316088657,
-0.152507693175629,-0.0540854058072747,0.),.UNSPECIFIED.);
#1343=B_SPLINE_CURVE_WITH_KNOTS('',3,(#68168,#68169,#68170,#68171),
 .UNSPECIFIED.,.F.,.F.,(4,4),(371.831581829739,372.244171931201),
 .UNSPECIFIED.);
#1344=B_SPLINE_CURVE_WITH_KNOTS('',3,(#68173,#68174,#68175,#68176,#68177,
#68178,#68179,#68180,#68181,#68182,#68183,#68184,#68185,#68186,#68187,#68188,
#68189,#68190,#68191,#68192,#68193,#68194,#68195,#68196,#68197,#68198,#68199,
#68200,#68201,#68202,#68203,#68204,#68205,#68206,#68207,#68208,#68209,#68210,
#68211,#68212,#68213,#68214,#68215,#68216,#68217,#68218,#68219,#68220,#68221,
#68222,#68223,#68224,#68225,#68226,#68227,#68228,#68229,#68230,#68231,#68232,
#68233,#68234,#68235,#68236,#68237,#68238,#68239,#68240,#68241,#68242,#68243,
#68244,#68245),.UNSPECIFIED.,.F.,.F.,(4,3,3,3,3,3,3,3,3,3,3,3,3,3,3,3,3,
3,3,3,3,3,3,3,4),(-1.53373699248741,-1.47998259246889,-1.39266174048294,
-1.36022791797891,-1.33444300979088,-1.23257109715798,-1.16841771016461,
-1.14505420410101,-1.13069918452509,-1.02732007613401,-0.923657890214898,
-0.893957590232833,-0.872515155439738,-0.767248151591644,-0.672999266808298,
-0.620634679898911,-0.597605365440628,-0.489854211146256,-0.39025261245826,
-0.338746494550714,-0.31133206291671,-0.288956014985721,-0.179727020905079,
-0.069639047355687,0.),.UNSPECIFIED.);
#1345=B_SPLINE_CURVE_WITH_KNOTS('',3,(#68246,#68247,#68248,#68249,#68250,
#68251,#68252,#68253,#68254,#68255,#68256),.UNSPECIFIED.,.F.,.F.,(4,1,1,
1,1,1,1,1,4),(10.3761157273109,11.2956825218578,12.2938669442682,13.2920513666786,
13.7911435778838,14.2902357890889,14.7893280002941,15.2884202114993,15.7079632679497),
 .UNSPECIFIED.);
#1346=B_SPLINE_CURVE_WITH_KNOTS('',3,(#68262,#68263,#68264,#68265,#68266,
#68267,#68268,#68269,#68270,#68271,#68272,#68273,#68274,#68275,#68276,#68277,
#68278,#68279,#68280,#68281,#68282,#68283,#68284,#68285,#68286,#68287,#68288,
#68289,#68290,#68291,#68292,#68293,#68294,#68295,#68296,#68297,#68298,#68299,
#68300,#68301,#68302,#68303,#68304,#68305,#68306,#68307,#68308,#68309,#68310,
#68311,#68312,#68313,#68314,#68315,#68316,#68317,#68318,#68319,#68320,#68321,
#68322,#68323,#68324,#68325,#68326,#68327,#68328,#68329,#68330,#68331,#68332,
#68333,#68334,#68335,#68336,#68337),.UNSPECIFIED.,.F.,.F.,(4,3,3,3,3,3,
3,3,3,3,3,3,3,3,3,3,3,3,3,3,3,3,3,3,3,4),(-1.52870610664519,-1.46664447796486,
-1.37006361368218,-1.32344222320996,-1.29493930957835,-1.18763016520624,
-1.12106166311689,-1.09619363797475,-1.08032102083414,-0.973278106621115,
-0.867444501594008,-0.829257794543526,-0.806280268864396,-0.706769958895627,
-0.616721647432272,-0.570817503170463,-0.54358942061174,-0.52268290565152,
-0.420869349933775,-0.346576713042208,-0.29808565610603,-0.273538172313205,
-0.252565316556387,-0.152507693644889,-0.0540854062652702,0.),
 .UNSPECIFIED.);
#1347=B_SPLINE_CURVE_WITH_KNOTS('',3,(#68340,#68341,#68342,#68343,#68344,
#68345,#68346,#68347,#68348,#68349),.UNSPECIFIED.,.F.,.F.,(4,1,1,1,1,1,
1,4),(11.6150328478189,12.1141250590241,12.6132172702293,13.1123094814345,
13.6114016926397,14.60958611505,15.6077705374604,15.7079632679496),
 .UNSPECIFIED.);
#1464=B_SPLINE_SURFACE_WITH_KNOTS('',2,1,((#64841,#64842),(#64843,#64844),
(#64845,#64846)),.UNSPECIFIED.,.F.,.F.,.F.,(3,3),(2,2),(0.,1.),(0.,0.04),
 .UNSPECIFIED.);
#1465=B_SPLINE_SURFACE_WITH_KNOTS('',2,1,((#64859,#64860),(#64861,#64862),
(#64863,#64864)),.UNSPECIFIED.,.F.,.F.,.F.,(3,3),(2,2),(0.,1.),(0.,0.04),
 .UNSPECIFIED.);
#1466=B_SPLINE_SURFACE_WITH_KNOTS('',2,1,((#64874,#64875),(#64876,#64877),
(#64878,#64879)),.UNSPECIFIED.,.F.,.F.,.F.,(3,3),(2,2),(0.,1.),(0.,0.04),
 .UNSPECIFIED.);
#1467=B_SPLINE_SURFACE_WITH_KNOTS('',2,1,((#64889,#64890),(#64891,#64892),
(#64893,#64894)),.UNSPECIFIED.,.F.,.F.,.F.,(3,3),(2,2),(0.,1.),(0.,0.04),
 .UNSPECIFIED.);
#1468=B_SPLINE_SURFACE_WITH_KNOTS('',2,1,((#64904,#64905),(#64906,#64907),
(#64908,#64909)),.UNSPECIFIED.,.F.,.F.,.F.,(3,3),(2,2),(0.,1.),(0.,0.04),
 .UNSPECIFIED.);
#1469=B_SPLINE_SURFACE_WITH_KNOTS('',2,1,((#64919,#64920),(#64921,#64922),
(#64923,#64924)),.UNSPECIFIED.,.F.,.F.,.F.,(3,3),(2,2),(0.,1.),(0.,0.04),
 .UNSPECIFIED.);
#1470=B_SPLINE_SURFACE_WITH_KNOTS('',2,1,((#64934,#64935),(#64936,#64937),
(#64938,#64939)),.UNSPECIFIED.,.F.,.F.,.F.,(3,3),(2,2),(0.,1.),(0.,0.04),
 .UNSPECIFIED.);
#1471=B_SPLINE_SURFACE_WITH_KNOTS('',2,1,((#64949,#64950),(#64951,#64952),
(#64953,#64954)),.UNSPECIFIED.,.F.,.F.,.F.,(3,3),(2,2),(0.,1.),(0.,0.04),
 .UNSPECIFIED.);
#1472=B_SPLINE_SURFACE_WITH_KNOTS('',2,1,((#64964,#64965),(#64966,#64967),
(#64968,#64969)),.UNSPECIFIED.,.F.,.F.,.F.,(3,3),(2,2),(0.,1.),(0.,0.04),
 .UNSPECIFIED.);
#1473=B_SPLINE_SURFACE_WITH_KNOTS('',2,1,((#64976,#64977),(#64978,#64979),
(#64980,#64981)),.UNSPECIFIED.,.F.,.F.,.F.,(3,3),(2,2),(0.,1.),(0.,0.04),
 .UNSPECIFIED.);
#1474=B_SPLINE_SURFACE_WITH_KNOTS('',2,1,((#64994,#64995),(#64996,#64997),
(#64998,#64999)),.UNSPECIFIED.,.F.,.F.,.F.,(3,3),(2,2),(0.,1.),(0.,0.04),
 .UNSPECIFIED.);
#1475=B_SPLINE_SURFACE_WITH_KNOTS('',2,1,((#65009,#65010),(#65011,#65012),
(#65013,#65014)),.UNSPECIFIED.,.F.,.F.,.F.,(3,3),(2,2),(0.,1.),(0.,0.04),
 .UNSPECIFIED.);
#1476=B_SPLINE_SURFACE_WITH_KNOTS('',2,1,((#65024,#65025),(#65026,#65027),
(#65028,#65029)),.UNSPECIFIED.,.F.,.F.,.F.,(3,3),(2,2),(0.,1.),(0.,0.04),
 .UNSPECIFIED.);
#1477=B_SPLINE_SURFACE_WITH_KNOTS('',2,1,((#65039,#65040),(#65041,#65042),
(#65043,#65044)),.UNSPECIFIED.,.F.,.F.,.F.,(3,3),(2,2),(0.,1.),(0.,0.04),
 .UNSPECIFIED.);
#1478=B_SPLINE_SURFACE_WITH_KNOTS('',2,1,((#65054,#65055),(#65056,#65057),
(#65058,#65059)),.UNSPECIFIED.,.F.,.F.,.F.,(3,3),(2,2),(0.,1.),(0.,0.04),
 .UNSPECIFIED.);
#1479=B_SPLINE_SURFACE_WITH_KNOTS('',2,1,((#65069,#65070),(#65071,#65072),
(#65073,#65074)),.UNSPECIFIED.,.F.,.F.,.F.,(3,3),(2,2),(0.,1.),(0.,0.04),
 .UNSPECIFIED.);
#1480=B_SPLINE_SURFACE_WITH_KNOTS('',2,1,((#65084,#65085),(#65086,#65087),
(#65088,#65089)),.UNSPECIFIED.,.F.,.F.,.F.,(3,3),(2,2),(0.,1.),(0.,0.04),
 .UNSPECIFIED.);
#1481=B_SPLINE_SURFACE_WITH_KNOTS('',2,1,((#65096,#65097),(#65098,#65099),
(#65100,#65101)),.UNSPECIFIED.,.F.,.F.,.F.,(3,3),(2,2),(0.,1.),(0.,0.04),
 .UNSPECIFIED.);
#1482=B_SPLINE_SURFACE_WITH_KNOTS('',2,1,((#65114,#65115),(#65116,#65117),
(#65118,#65119)),.UNSPECIFIED.,.F.,.F.,.F.,(3,3),(2,2),(0.,1.),(0.,0.04),
 .UNSPECIFIED.);
#1483=B_SPLINE_SURFACE_WITH_KNOTS('',2,1,((#65129,#65130),(#65131,#65132),
(#65133,#65134)),.UNSPECIFIED.,.F.,.F.,.F.,(3,3),(2,2),(0.,1.),(0.,0.04),
 .UNSPECIFIED.);
#1484=B_SPLINE_SURFACE_WITH_KNOTS('',2,1,((#65144,#65145),(#65146,#65147),
(#65148,#65149)),.UNSPECIFIED.,.F.,.F.,.F.,(3,3),(2,2),(0.,1.),(0.,0.04),
 .UNSPECIFIED.);
#1485=B_SPLINE_SURFACE_WITH_KNOTS('',2,1,((#65159,#65160),(#65161,#65162),
(#65163,#65164)),.UNSPECIFIED.,.F.,.F.,.F.,(3,3),(2,2),(0.,1.),(0.,0.04),
 .UNSPECIFIED.);
#1486=B_SPLINE_SURFACE_WITH_KNOTS('',2,1,((#65174,#65175),(#65176,#65177),
(#65178,#65179)),.UNSPECIFIED.,.F.,.F.,.F.,(3,3),(2,2),(0.,1.),(0.,0.04),
 .UNSPECIFIED.);
#1487=B_SPLINE_SURFACE_WITH_KNOTS('',2,1,((#65189,#65190),(#65191,#65192),
(#65193,#65194)),.UNSPECIFIED.,.F.,.F.,.F.,(3,3),(2,2),(0.,1.),(0.,0.04),
 .UNSPECIFIED.);
#1488=B_SPLINE_SURFACE_WITH_KNOTS('',2,1,((#65204,#65205),(#65206,#65207),
(#65208,#65209)),.UNSPECIFIED.,.F.,.F.,.F.,(3,3),(2,2),(0.,1.),(0.,0.04),
 .UNSPECIFIED.);
#1489=B_SPLINE_SURFACE_WITH_KNOTS('',2,1,((#65219,#65220),(#65221,#65222),
(#65223,#65224)),.UNSPECIFIED.,.F.,.F.,.F.,(3,3),(2,2),(0.,1.),(0.,0.04),
 .UNSPECIFIED.);
#1490=B_SPLINE_SURFACE_WITH_KNOTS('',2,1,((#65234,#65235),(#65236,#65237),
(#65238,#65239)),.UNSPECIFIED.,.F.,.F.,.F.,(3,3),(2,2),(0.,1.),(0.,0.04),
 .UNSPECIFIED.);
#1491=B_SPLINE_SURFACE_WITH_KNOTS('',2,1,((#65249,#65250),(#65251,#65252),
(#65253,#65254)),.UNSPECIFIED.,.F.,.F.,.F.,(3,3),(2,2),(0.,1.),(0.,0.04),
 .UNSPECIFIED.);
#1492=B_SPLINE_SURFACE_WITH_KNOTS('',2,1,((#65264,#65265),(#65266,#65267),
(#65268,#65269)),.UNSPECIFIED.,.F.,.F.,.F.,(3,3),(2,2),(0.,1.),(0.,0.04),
 .UNSPECIFIED.);
#1493=B_SPLINE_SURFACE_WITH_KNOTS('',2,1,((#65279,#65280),(#65281,#65282),
(#65283,#65284)),.UNSPECIFIED.,.F.,.F.,.F.,(3,3),(2,2),(0.,1.),(0.,0.04),
 .UNSPECIFIED.);
#1494=B_SPLINE_SURFACE_WITH_KNOTS('',2,1,((#65294,#65295),(#65296,#65297),
(#65298,#65299)),.UNSPECIFIED.,.F.,.F.,.F.,(3,3),(2,2),(0.,1.),(0.,0.04),
 .UNSPECIFIED.);
#1495=B_SPLINE_SURFACE_WITH_KNOTS('',2,1,((#65309,#65310),(#65311,#65312),
(#65313,#65314)),.UNSPECIFIED.,.F.,.F.,.F.,(3,3),(2,2),(0.,1.),(0.,0.04),
 .UNSPECIFIED.);
#1496=B_SPLINE_SURFACE_WITH_KNOTS('',2,1,((#65324,#65325),(#65326,#65327),
(#65328,#65329)),.UNSPECIFIED.,.F.,.F.,.F.,(3,3),(2,2),(0.,1.),(0.,0.04),
 .UNSPECIFIED.);
#1497=B_SPLINE_SURFACE_WITH_KNOTS('',2,1,((#65362,#65363),(#65364,#65365),
(#65366,#65367)),.UNSPECIFIED.,.F.,.F.,.F.,(3,3),(2,2),(0.,1.),(0.,0.04),
 .UNSPECIFIED.);
#1498=B_SPLINE_SURFACE_WITH_KNOTS('',2,1,((#65380,#65381),(#65382,#65383),
(#65384,#65385)),.UNSPECIFIED.,.F.,.F.,.F.,(3,3),(2,2),(0.,1.),(0.,0.04),
 .UNSPECIFIED.);
#1499=B_SPLINE_SURFACE_WITH_KNOTS('',2,1,((#65395,#65396),(#65397,#65398),
(#65399,#65400)),.UNSPECIFIED.,.F.,.F.,.F.,(3,3),(2,2),(0.,1.),(0.,0.04),
 .UNSPECIFIED.);
#1500=B_SPLINE_SURFACE_WITH_KNOTS('',2,1,((#65410,#65411),(#65412,#65413),
(#65414,#65415)),.UNSPECIFIED.,.F.,.F.,.F.,(3,3),(2,2),(0.,1.),(0.,0.04),
 .UNSPECIFIED.);
#1501=B_SPLINE_SURFACE_WITH_KNOTS('',2,1,((#65425,#65426),(#65427,#65428),
(#65429,#65430)),.UNSPECIFIED.,.F.,.F.,.F.,(3,3),(2,2),(0.,1.),(0.,0.04),
 .UNSPECIFIED.);
#1502=B_SPLINE_SURFACE_WITH_KNOTS('',2,1,((#65440,#65441),(#65442,#65443),
(#65444,#65445)),.UNSPECIFIED.,.F.,.F.,.F.,(3,3),(2,2),(0.,1.),(0.,0.04),
 .UNSPECIFIED.);
#1503=B_SPLINE_SURFACE_WITH_KNOTS('',2,1,((#65455,#65456),(#65457,#65458),
(#65459,#65460)),.UNSPECIFIED.,.F.,.F.,.F.,(3,3),(2,2),(0.,1.),(0.,0.04),
 .UNSPECIFIED.);
#1504=B_SPLINE_SURFACE_WITH_KNOTS('',2,1,((#65470,#65471),(#65472,#65473),
(#65474,#65475)),.UNSPECIFIED.,.F.,.F.,.F.,(3,3),(2,2),(0.,1.),(0.,0.04),
 .UNSPECIFIED.);
#1505=B_SPLINE_SURFACE_WITH_KNOTS('',2,1,((#65485,#65486),(#65487,#65488),
(#65489,#65490)),.UNSPECIFIED.,.F.,.F.,.F.,(3,3),(2,2),(0.,1.),(0.,0.04),
 .UNSPECIFIED.);
#1506=B_SPLINE_SURFACE_WITH_KNOTS('',2,1,((#65497,#65498),(#65499,#65500),
(#65501,#65502)),.UNSPECIFIED.,.F.,.F.,.F.,(3,3),(2,2),(0.,1.),(0.,0.04),
 .UNSPECIFIED.);
#1507=B_SPLINE_SURFACE_WITH_KNOTS('',2,1,((#65515,#65516),(#65517,#65518),
(#65519,#65520)),.UNSPECIFIED.,.F.,.F.,.F.,(3,3),(2,2),(0.,1.),(0.,0.04),
 .UNSPECIFIED.);
#1508=B_SPLINE_SURFACE_WITH_KNOTS('',2,1,((#65530,#65531),(#65532,#65533),
(#65534,#65535)),.UNSPECIFIED.,.F.,.F.,.F.,(3,3),(2,2),(0.,1.),(0.,0.04),
 .UNSPECIFIED.);
#1509=B_SPLINE_SURFACE_WITH_KNOTS('',2,1,((#65545,#65546),(#65547,#65548),
(#65549,#65550)),.UNSPECIFIED.,.F.,.F.,.F.,(3,3),(2,2),(0.,1.),(0.,0.04),
 .UNSPECIFIED.);
#1510=B_SPLINE_SURFACE_WITH_KNOTS('',2,1,((#65560,#65561),(#65562,#65563),
(#65564,#65565)),.UNSPECIFIED.,.F.,.F.,.F.,(3,3),(2,2),(0.,1.),(0.,0.04),
 .UNSPECIFIED.);
#1511=B_SPLINE_SURFACE_WITH_KNOTS('',2,1,((#65575,#65576),(#65577,#65578),
(#65579,#65580)),.UNSPECIFIED.,.F.,.F.,.F.,(3,3),(2,2),(0.,1.),(0.,0.04),
 .UNSPECIFIED.);
#1512=B_SPLINE_SURFACE_WITH_KNOTS('',2,1,((#65590,#65591),(#65592,#65593),
(#65594,#65595)),.UNSPECIFIED.,.F.,.F.,.F.,(3,3),(2,2),(0.,1.),(0.,0.04),
 .UNSPECIFIED.);
#1513=B_SPLINE_SURFACE_WITH_KNOTS('',2,1,((#65605,#65606),(#65607,#65608),
(#65609,#65610)),.UNSPECIFIED.,.F.,.F.,.F.,(3,3),(2,2),(0.,1.),(0.,0.04),
 .UNSPECIFIED.);
#1514=B_SPLINE_SURFACE_WITH_KNOTS('',2,1,((#65617,#65618),(#65619,#65620),
(#65621,#65622)),.UNSPECIFIED.,.F.,.F.,.F.,(3,3),(2,2),(0.,1.),(0.,0.04),
 .UNSPECIFIED.);
#1515=B_SPLINE_SURFACE_WITH_KNOTS('',2,1,((#65635,#65636),(#65637,#65638),
(#65639,#65640)),.UNSPECIFIED.,.F.,.F.,.F.,(3,3),(2,2),(0.,1.),(0.,0.04),
 .UNSPECIFIED.);
#1516=B_SPLINE_SURFACE_WITH_KNOTS('',2,1,((#65650,#65651),(#65652,#65653),
(#65654,#65655)),.UNSPECIFIED.,.F.,.F.,.F.,(3,3),(2,2),(0.,1.),(0.,0.04),
 .UNSPECIFIED.);
#1517=B_SPLINE_SURFACE_WITH_KNOTS('',2,1,((#65665,#65666),(#65667,#65668),
(#65669,#65670)),.UNSPECIFIED.,.F.,.F.,.F.,(3,3),(2,2),(0.,1.),(0.,0.04),
 .UNSPECIFIED.);
#1518=B_SPLINE_SURFACE_WITH_KNOTS('',2,1,((#65680,#65681),(#65682,#65683),
(#65684,#65685)),.UNSPECIFIED.,.F.,.F.,.F.,(3,3),(2,2),(0.,1.),(0.,0.04),
 .UNSPECIFIED.);
#1519=B_SPLINE_SURFACE_WITH_KNOTS('',2,1,((#65695,#65696),(#65697,#65698),
(#65699,#65700)),.UNSPECIFIED.,.F.,.F.,.F.,(3,3),(2,2),(0.,1.),(0.,0.04),
 .UNSPECIFIED.);
#1520=B_SPLINE_SURFACE_WITH_KNOTS('',2,1,((#65710,#65711),(#65712,#65713),
(#65714,#65715)),.UNSPECIFIED.,.F.,.F.,.F.,(3,3),(2,2),(0.,1.),(0.,0.04),
 .UNSPECIFIED.);
#1521=B_SPLINE_SURFACE_WITH_KNOTS('',2,1,((#65725,#65726),(#65727,#65728),
(#65729,#65730)),.UNSPECIFIED.,.F.,.F.,.F.,(3,3),(2,2),(0.,1.),(0.,0.04),
 .UNSPECIFIED.);
#1522=B_SPLINE_SURFACE_WITH_KNOTS('',2,1,((#65740,#65741),(#65742,#65743),
(#65744,#65745)),.UNSPECIFIED.,.F.,.F.,.F.,(3,3),(2,2),(0.,1.),(0.,0.04),
 .UNSPECIFIED.);
#1523=B_SPLINE_SURFACE_WITH_KNOTS('',2,1,((#65755,#65756),(#65757,#65758),
(#65759,#65760)),.UNSPECIFIED.,.F.,.F.,.F.,(3,3),(2,2),(0.,1.),(0.,0.04),
 .UNSPECIFIED.);
#1524=B_SPLINE_SURFACE_WITH_KNOTS('',2,1,((#65770,#65771),(#65772,#65773),
(#65774,#65775)),.UNSPECIFIED.,.F.,.F.,.F.,(3,3),(2,2),(0.,1.),(0.,0.04),
 .UNSPECIFIED.);
#1525=B_SPLINE_SURFACE_WITH_KNOTS('',2,1,((#65785,#65786),(#65787,#65788),
(#65789,#65790)),.UNSPECIFIED.,.F.,.F.,.F.,(3,3),(2,2),(0.,1.),(0.,0.04),
 .UNSPECIFIED.);
#1526=B_SPLINE_SURFACE_WITH_KNOTS('',2,1,((#65800,#65801),(#65802,#65803),
(#65804,#65805)),.UNSPECIFIED.,.F.,.F.,.F.,(3,3),(2,2),(0.,1.),(0.,0.04),
 .UNSPECIFIED.);
#1527=B_SPLINE_SURFACE_WITH_KNOTS('',2,1,((#65815,#65816),(#65817,#65818),
(#65819,#65820)),.UNSPECIFIED.,.F.,.F.,.F.,(3,3),(2,2),(0.,1.),(0.,0.04),
 .UNSPECIFIED.);
#1528=B_SPLINE_SURFACE_WITH_KNOTS('',2,1,((#65830,#65831),(#65832,#65833),
(#65834,#65835)),.UNSPECIFIED.,.F.,.F.,.F.,(3,3),(2,2),(0.,1.),(0.,0.04),
 .UNSPECIFIED.);
#1529=B_SPLINE_SURFACE_WITH_KNOTS('',2,1,((#65845,#65846),(#65847,#65848),
(#65849,#65850)),.UNSPECIFIED.,.F.,.F.,.F.,(3,3),(2,2),(0.,1.),(0.,0.04),
 .UNSPECIFIED.);
#1530=B_SPLINE_SURFACE_WITH_KNOTS('',3,3,((#66016,#66017,#66018,#66019,
#66020,#66021,#66022,#66023,#66024,#66025,#66026,#66027,#66028,#66029,#66030,
#66031,#66032,#66033,#66034,#66035,#66036,#66037,#66038,#66039,#66040,#66041,
#66042,#66043,#66044,#66045,#66046,#66047,#66048,#66049,#66050,#66051,#66052,
#66053,#66054,#66055,#66056,#66057,#66058,#66059,#66060,#66061,#66062,#66063,
#66064,#66065,#66066,#66067,#66068,#66069,#66070,#66071,#66072,#66073,#66074,
#66075,#66076,#66077,#66078,#66079,#66080,#66081,#66082,#66083,#66084,#66085,
#66086,#66087,#66088,#66089,#66090,#66091,#66092,#66093,#66094,#66095,#66096,
#66097,#66098,#66099,#66100,#66101,#66102,#66103,#66104,#66105,#66106,#66107,
#66108,#66109,#66110,#66111,#66112,#66113,#66114,#66115,#66116,#66117,#66118,
#66119,#66120,#66121,#66122,#66123,#66124,#66125,#66126,#66127,#66128,#66129,
#66130,#66131,#66132,#66133,#66134,#66135,#66136,#66137,#66138,#66139,#66140,
#66141,#66142,#66143,#66144,#66145,#66146,#66147,#66148,#66149,#66150,#66151,
#66152,#66153,#66154,#66155,#66156,#66157,#66158,#66159,#66160,#66161,#66162,
#66163,#66164,#66165,#66166,#66167,#66168,#66169,#66170,#66171,#66172,#66173,
#66174,#66175,#66176,#66177,#66178,#66179,#66180,#66181,#66182,#66183,#66184,
#66185,#66186,#66187,#66188,#66189,#66190,#66191,#66192,#66193,#66194,#66195,
#66196,#66197,#66198,#66199,#66200,#66201,#66202,#66203,#66204,#66205,#66206,
#66207,#66208,#66209,#66210,#66211,#66212,#66213,#66214,#66215,#66216,#66217,
#66218,#66219,#66220,#66221,#66222,#66223,#66224,#66225,#66226,#66227,#66228,
#66229,#66230,#66231,#66232,#66233,#66234,#66235,#66236,#66237,#66238,#66239,
#66240,#66241,#66242,#66243,#66244,#66245,#66246,#66247,#66248,#66249,#66250,
#66251,#66252,#66253,#66254,#66255,#66256,#66257,#66258,#66259,#66260,#66261,
#66262,#66263,#66264,#66265,#66266,#66267,#66268,#66269,#66270,#66271,#66272,
#66273,#66274,#66275,#66276,#66277,#66278,#66279,#66280,#66281,#66282,#66283,
#66284,#66285,#66286,#66287,#66288,#66289,#66290,#66291,#66292,#66293,#66294,
#66295,#66296,#66297,#66298,#66299,#66300,#66301,#66302,#66303,#66304,#66305,
#66306,#66307,#66308,#66309,#66310,#66311,#66312,#66313,#66314,#66315,#66316,
#66317,#66318,#66319,#66320,#66321,#66322,#66323,#66324,#66325,#66326,#66327,
#66328,#66329,#66330,#66331,#66332,#66333,#66334,#66335,#66336,#66337,#66338,
#66339,#66340,#66341,#66342,#66343,#66344,#66345,#66346,#66347,#66348,#66349,
#66350,#66351,#66352,#66353,#66354,#66355,#66356,#66357,#66358,#66359,#66360,
#66361,#66362,#66363,#66364,#66365,#66366,#66367,#66368,#66369,#66370,#66371,
#66372,#66373,#66374,#66375,#66376,#66377,#66378,#66379,#66380,#66381,#66382,
#66383,#66384,#66385,#66386,#66387,#66388,#66389,#66390,#66391,#66392,#66393,
#66394,#66395,#66396,#66397,#66398,#66399,#66400,#66401,#66402,#66403,#66404,
#66405,#66406,#66407,#66408,#66409,#66410,#66411,#66412,#66413,#66414,#66415,
#66416,#66417,#66418,#66419,#66420,#66421,#66422,#66423,#66424,#66425,#66426,
#66427,#66428,#66429,#66430,#66431,#66432,#66433,#66434,#66435,#66436,#66437,
#66438,#66439,#66440,#66441,#66442,#66443,#66444,#66445,#66446,#66447,#66448,
#66449,#66450,#66451,#66452,#66453,#66454,#66455,#66456,#66457,#66458,#66459,
#66460,#66461,#66462,#66463,#66464,#66465,#66466,#66467,#66468,#66469,#66470,
#66471,#66472,#66473,#66474,#66475,#66476,#66477,#66478,#66479,#66480,#66481,
#66482,#66483,#66484,#66485,#66486,#66487,#66488,#66489,#66490,#66491,#66492,
#66493,#66494,#66495,#66496,#66497,#66498,#66499,#66500,#66501,#66502,#66503,
#66504,#66505,#66506,#66507,#66508,#66509,#66510,#66511,#66512,#66513,#66514,
#66515,#66516,#66517,#66518,#66519,#66520,#66521,#66522,#66523,#66524,#66525,
#66526,#66527,#66528,#66529,#66530,#66531,#66532,#66533,#66534,#66535,#66536,
#66537,#66538,#66539,#66540,#66541,#66542,#66543,#66544,#66545,#66546,#66547,
#66548,#66549,#66550,#66551,#66552,#66553),(#66554,#66555,#66556,#66557,
#66558,#66559,#66560,#66561,#66562,#66563,#66564,#66565,#66566,#66567,#66568,
#66569,#66570,#66571,#66572,#66573,#66574,#66575,#66576,#66577,#66578,#66579,
#66580,#66581,#66582,#66583,#66584,#66585,#66586,#66587,#66588,#66589,#66590,
#66591,#66592,#66593,#66594,#66595,#66596,#66597,#66598,#66599,#66600,#66601,
#66602,#66603,#66604,#66605,#66606,#66607,#66608,#66609,#66610,#66611,#66612,
#66613,#66614,#66615,#66616,#66617,#66618,#66619,#66620,#66621,#66622,#66623,
#66624,#66625,#66626,#66627,#66628,#66629,#66630,#66631,#66632,#66633,#66634,
#66635,#66636,#66637,#66638,#66639,#66640,#66641,#66642,#66643,#66644,#66645,
#66646,#66647,#66648,#66649,#66650,#66651,#66652,#66653,#66654,#66655,#66656,
#66657,#66658,#66659,#66660,#66661,#66662,#66663,#66664,#66665,#66666,#66667,
#66668,#66669,#66670,#66671,#66672,#66673,#66674,#66675,#66676,#66677,#66678,
#66679,#66680,#66681,#66682,#66683,#66684,#66685,#66686,#66687,#66688,#66689,
#66690,#66691,#66692,#66693,#66694,#66695,#66696,#66697,#66698,#66699,#66700,
#66701,#66702,#66703,#66704,#66705,#66706,#66707,#66708,#66709,#66710,#66711,
#66712,#66713,#66714,#66715,#66716,#66717,#66718,#66719,#66720,#66721,#66722,
#66723,#66724,#66725,#66726,#66727,#66728,#66729,#66730,#66731,#66732,#66733,
#66734,#66735,#66736,#66737,#66738,#66739,#66740,#66741,#66742,#66743,#66744,
#66745,#66746,#66747,#66748,#66749,#66750,#66751,#66752,#66753,#66754,#66755,
#66756,#66757,#66758,#66759,#66760,#66761,#66762,#66763,#66764,#66765,#66766,
#66767,#66768,#66769,#66770,#66771,#66772,#66773,#66774,#66775,#66776,#66777,
#66778,#66779,#66780,#66781,#66782,#66783,#66784,#66785,#66786,#66787,#66788,
#66789,#66790,#66791,#66792,#66793,#66794,#66795,#66796,#66797,#66798,#66799,
#66800,#66801,#66802,#66803,#66804,#66805,#66806,#66807,#66808,#66809,#66810,
#66811,#66812,#66813,#66814,#66815,#66816,#66817,#66818,#66819,#66820,#66821,
#66822,#66823,#66824,#66825,#66826,#66827,#66828,#66829,#66830,#66831,#66832,
#66833,#66834,#66835,#66836,#66837,#66838,#66839,#66840,#66841,#66842,#66843,
#66844,#66845,#66846,#66847,#66848,#66849,#66850,#66851,#66852,#66853,#66854,
#66855,#66856,#66857,#66858,#66859,#66860,#66861,#66862,#66863,#66864,#66865,
#66866,#66867,#66868,#66869,#66870,#66871,#66872,#66873,#66874,#66875,#66876,
#66877,#66878,#66879,#66880,#66881,#66882,#66883,#66884,#66885,#66886,#66887,
#66888,#66889,#66890,#66891,#66892,#66893,#66894,#66895,#66896,#66897,#66898,
#66899,#66900,#66901,#66902,#66903,#66904,#66905,#66906,#66907,#66908,#66909,
#66910,#66911,#66912,#66913,#66914,#66915,#66916,#66917,#66918,#66919,#66920,
#66921,#66922,#66923,#66924,#66925,#66926,#66927,#66928,#66929,#66930,#66931,
#66932,#66933,#66934,#66935,#66936,#66937,#66938,#66939,#66940,#66941,#66942,
#66943,#66944,#66945,#66946,#66947,#66948,#66949,#66950,#66951,#66952,#66953,
#66954,#66955,#66956,#66957,#66958,#66959,#66960,#66961,#66962,#66963,#66964,
#66965,#66966,#66967,#66968,#66969,#66970,#66971,#66972,#66973,#66974,#66975,
#66976,#66977,#66978,#66979,#66980,#66981,#66982,#66983,#66984,#66985,#66986,
#66987,#66988,#66989,#66990,#66991,#66992,#66993,#66994,#66995,#66996,#66997,
#66998,#66999,#67000,#67001,#67002,#67003,#67004,#67005,#67006,#67007,#67008,
#67009,#67010,#67011,#67012,#67013,#67014,#67015,#67016,#67017,#67018,#67019,
#67020,#67021,#67022,#67023,#67024,#67025,#67026,#67027,#67028,#67029,#67030,
#67031,#67032,#67033,#67034,#67035,#67036,#67037,#67038,#67039,#67040,#67041,
#67042,#67043,#67044,#67045,#67046,#67047,#67048,#67049,#67050,#67051,#67052,
#67053,#67054,#67055,#67056,#67057,#67058,#67059,#67060,#67061,#67062,#67063,
#67064,#67065,#67066,#67067,#67068,#67069,#67070,#67071,#67072,#67073,#67074,
#67075,#67076,#67077,#67078,#67079,#67080,#67081,#67082,#67083,#67084,#67085,
#67086,#67087,#67088,#67089,#67090,#67091),(#67092,#67093,#67094,#67095,
#67096,#67097,#67098,#67099,#67100,#67101,#67102,#67103,#67104,#67105,#67106,
#67107,#67108,#67109,#67110,#67111,#67112,#67113,#67114,#67115,#67116,#67117,
#67118,#67119,#67120,#67121,#67122,#67123,#67124,#67125,#67126,#67127,#67128,
#67129,#67130,#67131,#67132,#67133,#67134,#67135,#67136,#67137,#67138,#67139,
#67140,#67141,#67142,#67143,#67144,#67145,#67146,#67147,#67148,#67149,#67150,
#67151,#67152,#67153,#67154,#67155,#67156,#67157,#67158,#67159,#67160,#67161,
#67162,#67163,#67164,#67165,#67166,#67167,#67168,#67169,#67170,#67171,#67172,
#67173,#67174,#67175,#67176,#67177,#67178,#67179,#67180,#67181,#67182,#67183,
#67184,#67185,#67186,#67187,#67188,#67189,#67190,#67191,#67192,#67193,#67194,
#67195,#67196,#67197,#67198,#67199,#67200,#67201,#67202,#67203,#67204,#67205,
#67206,#67207,#67208,#67209,#67210,#67211,#67212,#67213,#67214,#67215,#67216,
#67217,#67218,#67219,#67220,#67221,#67222,#67223,#67224,#67225,#67226,#67227,
#67228,#67229,#67230,#67231,#67232,#67233,#67234,#67235,#67236,#67237,#67238,
#67239,#67240,#67241,#67242,#67243,#67244,#67245,#67246,#67247,#67248,#67249,
#67250,#67251,#67252,#67253,#67254,#67255,#67256,#67257,#67258,#67259,#67260,
#67261,#67262,#67263,#67264,#67265,#67266,#67267,#67268,#67269,#67270,#67271,
#67272,#67273,#67274,#67275,#67276,#67277,#67278,#67279,#67280,#67281,#67282,
#67283,#67284,#67285,#67286,#67287,#67288,#67289,#67290,#67291,#67292,#67293,
#67294,#67295,#67296,#67297,#67298,#67299,#67300,#67301,#67302,#67303,#67304,
#67305,#67306,#67307,#67308,#67309,#67310,#67311,#67312,#67313,#67314,#67315,
#67316,#67317,#67318,#67319,#67320,#67321,#67322,#67323,#67324,#67325,#67326,
#67327,#67328,#67329,#67330,#67331,#67332,#67333,#67334,#67335,#67336,#67337,
#67338,#67339,#67340,#67341,#67342,#67343,#67344,#67345,#67346,#67347,#67348,
#67349,#67350,#67351,#67352,#67353,#67354,#67355,#67356,#67357,#67358,#67359,
#67360,#67361,#67362,#67363,#67364,#67365,#67366,#67367,#67368,#67369,#67370,
#67371,#67372,#67373,#67374,#67375,#67376,#67377,#67378,#67379,#67380,#67381,
#67382,#67383,#67384,#67385,#67386,#67387,#67388,#67389,#67390,#67391,#67392,
#67393,#67394,#67395,#67396,#67397,#67398,#67399,#67400,#67401,#67402,#67403,
#67404,#67405,#67406,#67407,#67408,#67409,#67410,#67411,#67412,#67413,#67414,
#67415,#67416,#67417,#67418,#67419,#67420,#67421,#67422,#67423,#67424,#67425,
#67426,#67427,#67428,#67429,#67430,#67431,#67432,#67433,#67434,#67435,#67436,
#67437,#67438,#67439,#67440,#67441,#67442,#67443,#67444,#67445,#67446,#67447,
#67448,#67449,#67450,#67451,#67452,#67453,#67454,#67455,#67456,#67457,#67458,
#67459,#67460,#67461,#67462,#67463,#67464,#67465,#67466,#67467,#67468,#67469,
#67470,#67471,#67472,#67473,#67474,#67475,#67476,#67477,#67478,#67479,#67480,
#67481,#67482,#67483,#67484,#67485,#67486,#67487,#67488,#67489,#67490,#67491,
#67492,#67493,#67494,#67495,#67496,#67497,#67498,#67499,#67500,#67501,#67502,
#67503,#67504,#67505,#67506,#67507,#67508,#67509,#67510,#67511,#67512,#67513,
#67514,#67515,#67516,#67517,#67518,#67519,#67520,#67521,#67522,#67523,#67524,
#67525,#67526,#67527,#67528,#67529,#67530,#67531,#67532,#67533,#67534,#67535,
#67536,#67537,#67538,#67539,#67540,#67541,#67542,#67543,#67544,#67545,#67546,
#67547,#67548,#67549,#67550,#67551,#67552,#67553,#67554,#67555,#67556,#67557,
#67558,#67559,#67560,#67561,#67562,#67563,#67564,#67565,#67566,#67567,#67568,
#67569,#67570,#67571,#67572,#67573,#67574,#67575,#67576,#67577,#67578,#67579,
#67580,#67581,#67582,#67583,#67584,#67585,#67586,#67587,#67588,#67589,#67590,
#67591,#67592,#67593,#67594,#67595,#67596,#67597,#67598,#67599,#67600,#67601,
#67602,#67603,#67604,#67605,#67606,#67607,#67608,#67609,#67610,#67611,#67612,
#67613,#67614,#67615,#67616,#67617,#67618,#67619,#67620,#67621,#67622,#67623,
#67624,#67625,#67626,#67627,#67628,#67629),(#67630,#67631,#67632,#67633,
#67634,#67635,#67636,#67637,#67638,#67639,#67640,#67641,#67642,#67643,#67644,
#67645,#67646,#67647,#67648,#67649,#67650,#67651,#67652,#67653,#67654,#67655,
#67656,#67657,#67658,#67659,#67660,#67661,#67662,#67663,#67664,#67665,#67666,
#67667,#67668,#67669,#67670,#67671,#67672,#67673,#67674,#67675,#67676,#67677,
#67678,#67679,#67680,#67681,#67682,#67683,#67684,#67685,#67686,#67687,#67688,
#67689,#67690,#67691,#67692,#67693,#67694,#67695,#67696,#67697,#67698,#67699,
#67700,#67701,#67702,#67703,#67704,#67705,#67706,#67707,#67708,#67709,#67710,
#67711,#67712,#67713,#67714,#67715,#67716,#67717,#67718,#67719,#67720,#67721,
#67722,#67723,#67724,#67725,#67726,#67727,#67728,#67729,#67730,#67731,#67732,
#67733,#67734,#67735,#67736,#67737,#67738,#67739,#67740,#67741,#67742,#67743,
#67744,#67745,#67746,#67747,#67748,#67749,#67750,#67751,#67752,#67753,#67754,
#67755,#67756,#67757,#67758,#67759,#67760,#67761,#67762,#67763,#67764,#67765,
#67766,#67767,#67768,#67769,#67770,#67771,#67772,#67773,#67774,#67775,#67776,
#67777,#67778,#67779,#67780,#67781,#67782,#67783,#67784,#67785,#67786,#67787,
#67788,#67789,#67790,#67791,#67792,#67793,#67794,#67795,#67796,#67797,#67798,
#67799,#67800,#67801,#67802,#67803,#67804,#67805,#67806,#67807,#67808,#67809,
#67810,#67811,#67812,#67813,#67814,#67815,#67816,#67817,#67818,#67819,#67820,
#67821,#67822,#67823,#67824,#67825,#67826,#67827,#67828,#67829,#67830,#67831,
#67832,#67833,#67834,#67835,#67836,#67837,#67838,#67839,#67840,#67841,#67842,
#67843,#67844,#67845,#67846,#67847,#67848,#67849,#67850,#67851,#67852,#67853,
#67854,#67855,#67856,#67857,#67858,#67859,#67860,#67861,#67862,#67863,#67864,
#67865,#67866,#67867,#67868,#67869,#67870,#67871,#67872,#67873,#67874,#67875,
#67876,#67877,#67878,#67879,#67880,#67881,#67882,#67883,#67884,#67885,#67886,
#67887,#67888,#67889,#67890,#67891,#67892,#67893,#67894,#67895,#67896,#67897,
#67898,#67899,#67900,#67901,#67902,#67903,#67904,#67905,#67906,#67907,#67908,
#67909,#67910,#67911,#67912,#67913,#67914,#67915,#67916,#67917,#67918,#67919,
#67920,#67921,#67922,#67923,#67924,#67925,#67926,#67927,#67928,#67929,#67930,
#67931,#67932,#67933,#67934,#67935,#67936,#67937,#67938,#67939,#67940,#67941,
#67942,#67943,#67944,#67945,#67946,#67947,#67948,#67949,#67950,#67951,#67952,
#67953,#67954,#67955,#67956,#67957,#67958,#67959,#67960,#67961,#67962,#67963,
#67964,#67965,#67966,#67967,#67968,#67969,#67970,#67971,#67972,#67973,#67974,
#67975,#67976,#67977,#67978,#67979,#67980,#67981,#67982,#67983,#67984,#67985,
#67986,#67987,#67988,#67989,#67990,#67991,#67992,#67993,#67994,#67995,#67996,
#67997,#67998,#67999,#68000,#68001,#68002,#68003,#68004,#68005,#68006,#68007,
#68008,#68009,#68010,#68011,#68012,#68013,#68014,#68015,#68016,#68017,#68018,
#68019,#68020,#68021,#68022,#68023,#68024,#68025,#68026,#68027,#68028,#68029,
#68030,#68031,#68032,#68033,#68034,#68035,#68036,#68037,#68038,#68039,#68040,
#68041,#68042,#68043,#68044,#68045,#68046,#68047,#68048,#68049,#68050,#68051,
#68052,#68053,#68054,#68055,#68056,#68057,#68058,#68059,#68060,#68061,#68062,
#68063,#68064,#68065,#68066,#68067,#68068,#68069,#68070,#68071,#68072,#68073,
#68074,#68075,#68076,#68077,#68078,#68079,#68080,#68081,#68082,#68083,#68084,
#68085,#68086,#68087,#68088,#68089,#68090,#68091,#68092,#68093,#68094,#68095,
#68096,#68097,#68098,#68099,#68100,#68101,#68102,#68103,#68104,#68105,#68106,
#68107,#68108,#68109,#68110,#68111,#68112,#68113,#68114,#68115,#68116,#68117,
#68118,#68119,#68120,#68121,#68122,#68123,#68124,#68125,#68126,#68127,#68128,
#68129,#68130,#68131,#68132,#68133,#68134,#68135,#68136,#68137,#68138,#68139,
#68140,#68141,#68142,#68143,#68144,#68145,#68146,#68147,#68148,#68149,#68150,
#68151,#68152,#68153,#68154,#68155,#68156,#68157,#68158,#68159,#68160,#68161,
#68162,#68163,#68164,#68165,#68166,#68167)),.UNSPECIFIED.,.F.,.F.,.F.,(4,
4),(4,1,1,1,1,1,1,1,1,1,1,1,1,1,1,1,1,1,1,1,1,1,1,1,1,1,1,1,1,1,1,1,1,1,
1,1,1,1,1,1,1,1,1,1,1,1,1,1,1,1,1,1,1,1,1,1,1,1,1,1,1,1,1,1,1,1,1,1,1,1,
1,1,1,1,1,1,1,1,1,1,1,1,1,1,1,1,1,1,1,1,1,1,1,1,1,1,1,1,1,1,1,1,1,1,1,1,
1,1,1,1,1,1,1,1,1,1,1,1,1,1,1,1,1,1,1,1,1,1,1,1,1,1,1,1,1,1,1,1,1,1,1,1,
1,1,1,1,1,1,1,1,1,1,1,1,1,1,1,1,1,1,1,1,1,1,1,1,1,1,1,1,1,1,1,1,1,1,1,1,
1,1,1,1,1,1,1,1,1,1,1,1,1,1,1,1,1,1,1,1,1,1,1,1,1,1,1,1,1,1,1,1,1,1,1,1,
1,1,1,1,1,1,1,1,1,1,1,1,1,1,1,1,1,1,1,1,1,1,1,1,1,1,1,1,1,1,1,1,1,1,1,1,
1,1,1,1,1,1,1,1,1,1,1,1,1,1,1,1,1,1,1,1,1,1,1,1,1,1,1,1,1,1,1,1,1,1,1,1,
1,1,1,1,1,1,1,1,1,1,1,1,1,1,1,1,1,1,1,1,1,1,1,1,1,1,1,1,1,1,1,1,1,1,1,1,
1,1,1,1,1,1,1,1,1,1,1,1,1,1,1,1,1,1,1,1,1,1,1,1,1,1,1,1,1,1,1,1,1,1,1,1,
1,1,1,1,1,1,1,1,1,1,1,1,1,1,1,1,1,1,1,1,1,1,1,1,1,1,1,1,1,1,1,1,1,1,1,1,
1,1,1,1,1,1,1,1,1,1,1,1,1,1,1,1,1,1,1,1,1,1,1,1,1,1,1,1,1,1,1,1,1,1,1,1,
1,1,1,1,1,1,1,1,1,1,1,1,1,1,1,1,1,1,1,1,1,1,1,1,1,1,1,1,1,1,1,1,1,1,1,1,
1,1,1,1,1,1,1,1,1,1,1,1,1,1,1,1,1,1,1,1,1,1,1,1,1,1,1,1,1,1,1,1,1,1,1,1,
1,1,1,1,1,1,1,1,1,1,1,1,1,1,1,1,1,1,1,1,1,1,1,1,1,1,1,1,1,1,1,1,1,4),(0.,
0.132097741590587),(8.30112925462677,8.80022146583195,9.29931367703713,
9.79840588824231,10.2974980994475,11.2956825218578,12.2938669442682,13.2920513666786,
13.7911435778838,14.2902357890889,14.7893280002941,15.2884202114993,16.2866046339097,
16.7856968451148,17.28478905632,18.2829734787304,19.2811579011407,20.2793423235511,
20.7784345347563,21.2775267459615,21.7766189571666,22.2757111683718,23.2738955907822,
23.7729878019874,24.2720800131925,25.2702644356029,26.2684488580133,27.2666332804236,
27.7657254916288,28.264817702834,28.7639099140392,29.2630021252443,30.2611865476547,
30.7602787588599,31.2593709700651,32.2575553924754,33.2557398148858,34.2539242372961,
34.7530164485013,35.2521086597065,35.7512008709117,36.2502930821169,37.2484775045272,
37.7475697157324,38.2466619269376,39.2448463493479,40.2430307717583,41.2412151941687,
41.7403074053738,42.239399616579,42.7384918277842,43.2375840389894,44.2357684613998,
44.7348606726049,45.2339528838101,46.2321373062205,47.2303217286308,48.2285061510412,
48.7275983622464,49.2266905734515,49.7257827846567,50.2248749958619,51.2230594182723,
51.7221516294775,52.2212438406826,53.219428263093,54.2176126855034,55.2157971079137,
55.7148893191189,56.2139815303241,56.7130737415293,57.2121659527344,58.2103503751448,
58.70944258635,59.2085347975552,60.2067192199655,61.2049036423759,62.2030880647862,
62.7021802759914,63.2012724871966,63.7003646984018,64.199456909607,65.1976413320173,
65.6967335432225,66.1958257544277,67.194010176838,68.1921945992484,69.1903790216588,
69.689471232864,70.1885634440691,70.6876556552743,71.1867478664795,72.1849322888899,
72.684024500095,73.1831167113002,74.1813011337106,75.1794855561209,76.1776699785313,
76.6767621897365,77.1758544009417,77.6749466121468,78.174038823352,79.1722232457624,
79.6713154569676,80.1704076681727,81.1685920905831,82.1667765129935,83.1649609354038,
83.664053146609,84.1631453578142,84.6622375690194,85.1613297802245,86.1595142026349,
86.6586064138401,87.1576986250453,88.1558830474556,89.154067469866,90.1522518922763,
90.6513441034815,91.1504363146867,91.6495285258919,92.1486207370971,93.1468051595074,
93.6458973707126,94.1449895819178,95.1431740043281,96.1413584267385,97.1395428491489,
97.638635060354,98.1377272715592,98.6368194827644,99.1359116939696,100.13409611638,
100.633188327585,101.13228053879,102.130464961201,103.128649383611,104.126833806021,
104.625926017227,105.125018228432,105.624110439637,106.123202650842,107.121387073252,
107.620479284458,108.119571495663,109.117755918073,110.115940340484,111.114124762894,
111.613216974099,112.112309185304,112.611401396509,113.110493607715,114.108678030125,
114.60777024133,115.106862452535,116.105046874946,117.103231297356,118.101415719766,
118.600507930972,119.099600142177,119.598692353382,120.097784564587,121.095968986998,
121.595061198203,122.094153409408,123.092337831818,124.090522254229,125.088706676639,
125.587798887844,126.086891099049,126.585983310255,127.08507552146,128.08325994387,
128.582352155075,129.08144436628,130.079628788691,131.077813211101,132.075997633511,
132.575089844717,133.074182055922,133.573274267127,134.072366478332,135.070550900743,
135.569643111948,136.068735323153,137.066919745563,138.065104167974,139.063288590384,
139.562380801589,140.061473012794,140.560565224,141.059657435205,142.057841857615,
142.55693406882,143.056026280025,144.054210702436,145.052395124846,146.050579547257,
146.549671758462,147.048763969667,147.547856180872,148.046948392077,149.045132814488,
149.544225025693,150.043317236898,151.041501659308,152.039686081719,153.037870504129,
153.536962715334,154.036054926539,154.535147137745,155.03423934895,156.03242377136,
156.531515982565,157.030608193771,158.028792616181,159.026977038591,160.025161461002,
160.524253672207,161.023345883412,161.522438094617,162.021530305822,163.019714728233,
163.518806939438,164.017899150643,165.016083573053,166.014267995464,167.012452417874,
167.511544629079,168.010636840284,168.50972905149,169.008821262695,170.007005685105,
170.50609789631,171.005190107516,172.003374529926,173.001558952336,173.999743374747,
174.498835585952,174.997927797157,175.497020008362,175.996112219567,176.994296641978,
177.493388853183,177.992481064388,178.990665486798,179.988849909209,180.987034331619,
181.486126542824,181.98521875403,182.484310965235,182.98340317644,183.98158759885,
184.480679810055,184.979772021261,185.977956443671,186.976140866081,187.974325288492,
188.473417499697,188.972509710902,189.471601922107,189.970694133312,190.968878555723,
191.467970766928,191.967062978133,192.965247400543,193.963431822954,194.961616245364,
195.959800667775,196.957985090185,197.956169512595,198.954353935006,199.453446146211,
199.952538357416,200.950722779826,201.449814991032,201.948907202237,202.447999413442,
202.947091624647,203.945276047057,204.943460469468,205.941644891878,206.440737103083,
206.939829314289,207.938013736699,208.437105947904,208.936198159109,209.435290370314,
209.93438258152,210.93256700393,211.93075142634,212.928935848751,213.428028059956,
213.927120271161,214.925304693571,215.424396904777,215.923489115982,216.422581327187,
216.921673538392,217.919857960803,218.918042383213,219.916226805623,220.415319016828,
220.914411228034,221.912595650444,222.411687861649,222.910780072854,223.40987228406,
223.908964495265,224.907148917675,225.905333340085,226.903517762496,227.402609973701,
227.901702184906,228.899886607316,229.398978818522,229.898071029727,230.397163240932,
230.896255452137,231.894439874548,232.892624296958,233.890808719368,234.389900930573,
234.888993141779,235.887177564189,236.386269775394,236.885361986599,237.384454197805,
237.88354640901,238.88173083142,239.87991525383,240.878099676241,241.377191887446,
241.876284098651,242.874468521062,243.373560732267,243.872652943472,244.371745154677,
244.870837365882,245.869021788293,246.867206210703,247.865390633113,248.364482844319,
248.863575055524,249.861759477934,250.360851689139,250.859943900344,251.35903611155,
251.858128322755,252.856312745165,253.854497167575,254.852681589986,255.351773801191,
255.850866012396,256.849050434807,257.348142646012,257.847234857217,258.346327068422,
258.845419279627,259.843603702038,260.841788124448,261.839972546858,262.339064758064,
262.838156969269,263.836341391679,264.335433602884,264.834525814089,265.333618025295,
265.8327102365,266.83089465891,267.829079081321,268.827263503731,269.326355714936,
269.825447926141,270.823632348552,271.322724559757,271.821816770962,272.320908982167,
272.820001193372,273.818185615783,274.816370038193,275.814554460603,276.313646671809,
276.812738883014,277.810923305424,278.310015516629,278.809107727834,279.30819993904,
279.807292150245,280.805476572655,281.803660995066,282.801845417476,283.300937628681,
283.800029839886,284.798214262297,285.297306473502,285.796398684707,286.295490895912,
286.794583107117,287.792767529528,288.790951951938,289.789136374348,290.288228585554,
290.787320796759,291.785505219169,292.284597430374,292.78368964158,293.282781852785,
293.78187406399,294.7800584864,295.778242908811,296.776427331221,297.275519542426,
297.774611753631,298.772796176042,299.271888387247,299.770980598452,300.270072809657,
300.769165020862,301.767349443273,302.765533865683,303.763718288094,304.262810499299,
304.761902710504,305.760087132914,306.259179344119,306.758271555325,307.25736376653,
307.756455977735,308.754640400145,309.752824822556,310.751009244966,311.250101456171,
311.749193667376,312.747378089787,313.246470300992,313.745562512197,314.244654723402,
314.743746934607,315.741931357018,316.740115779428,317.738300201839,318.237392413044,
318.736484624249,319.734669046659,320.233761257864,320.73285346907,321.231945680275,
321.73103789148,322.72922231389,323.727406736301,324.725591158711,325.224683369916,
325.723775581121,326.721960003532,327.221052214737,327.720144425942,328.219236637147,
328.718328848352,329.716513270763,330.714697693173,331.712882115584,332.211974326789,
332.711066537994,333.709250960404,334.208343171609,334.707435382815,335.20652759402,
335.705619805225,336.703804227635,337.701988650046,338.700173072456,339.199265283661,
339.698357494866,340.696541917277,341.195634128482,341.694726339687,342.193818550892,
342.692910762098,343.691095184508,344.689279606918,345.687464029329,346.186556240534,
346.685648451739,347.683832874149,348.182925085355,348.68201729656,349.181109507765,
349.68020171897,350.67838614138,351.676570563791,352.674754986201,353.173847197406,
353.672939408612,354.671123831022,355.170216042227,355.669308253432,356.168400464637,
356.667492675843,357.665677098253,358.663861520663,359.662045943074,360.161138154279,
360.660230365484,361.658414787894,362.1575069991,362.656599210305,363.15569142151,
363.654783632715,364.652968055125,365.651152477536,366.649336899946,367.148429111151,
367.647521322357,368.645705744767,369.144797955972,369.643890167177,370.142982378382,
370.642074589588,371.640259011998,372.638443434408,373.636627856819,374.135720068024,
374.634812279229,375.632996701639,376.132088912845,376.63118112405,377.130273335255,
377.62936554646,378.627549968871,379.625734391281,380.623918813691,381.123011024896,
381.622103236102,382.121195447307,382.620287658512),.UNSPECIFIED.);
#1531=B_SPLINE_SURFACE_WITH_KNOTS('',3,3,((#68350,#68351,#68352,#68353,
#68354,#68355,#68356,#68357,#68358,#68359,#68360,#68361,#68362,#68363,#68364,
#68365,#68366,#68367,#68368,#68369,#68370,#68371,#68372,#68373,#68374,#68375,
#68376,#68377,#68378,#68379,#68380,#68381,#68382,#68383,#68384,#68385,#68386,
#68387,#68388,#68389,#68390,#68391,#68392,#68393,#68394,#68395,#68396,#68397,
#68398,#68399,#68400,#68401,#68402,#68403,#68404,#68405,#68406,#68407,#68408,
#68409,#68410,#68411,#68412,#68413,#68414,#68415,#68416,#68417,#68418,#68419,
#68420,#68421,#68422,#68423,#68424,#68425,#68426,#68427,#68428,#68429,#68430,
#68431,#68432,#68433,#68434,#68435,#68436,#68437,#68438,#68439,#68440,#68441,
#68442,#68443,#68444,#68445,#68446,#68447,#68448,#68449,#68450,#68451,#68452,
#68453,#68454,#68455,#68456,#68457,#68458,#68459,#68460,#68461,#68462,#68463,
#68464,#68465,#68466,#68467,#68468,#68469,#68470,#68471,#68472,#68473,#68474,
#68475,#68476,#68477,#68478,#68479,#68480,#68481,#68482,#68483,#68484,#68485,
#68486,#68487,#68488,#68489,#68490,#68491,#68492,#68493,#68494,#68495,#68496,
#68497,#68498,#68499,#68500,#68501,#68502,#68503,#68504,#68505,#68506,#68507,
#68508,#68509,#68510,#68511,#68512,#68513,#68514,#68515,#68516,#68517,#68518,
#68519,#68520,#68521,#68522,#68523,#68524,#68525,#68526,#68527,#68528,#68529,
#68530,#68531,#68532,#68533,#68534,#68535,#68536,#68537,#68538,#68539,#68540,
#68541,#68542,#68543,#68544,#68545,#68546,#68547,#68548,#68549,#68550,#68551,
#68552,#68553,#68554,#68555,#68556,#68557,#68558,#68559,#68560,#68561,#68562,
#68563,#68564,#68565,#68566,#68567,#68568,#68569,#68570,#68571,#68572,#68573,
#68574,#68575,#68576,#68577,#68578,#68579,#68580,#68581,#68582,#68583,#68584,
#68585,#68586,#68587,#68588,#68589,#68590,#68591,#68592,#68593,#68594,#68595,
#68596,#68597,#68598,#68599,#68600,#68601,#68602,#68603,#68604,#68605,#68606,
#68607,#68608,#68609,#68610,#68611,#68612,#68613,#68614,#68615,#68616,#68617,
#68618,#68619,#68620,#68621,#68622,#68623,#68624,#68625,#68626,#68627,#68628,
#68629,#68630,#68631,#68632,#68633,#68634,#68635,#68636,#68637,#68638,#68639,
#68640,#68641,#68642,#68643,#68644,#68645,#68646,#68647,#68648,#68649,#68650,
#68651,#68652,#68653,#68654,#68655,#68656,#68657,#68658,#68659,#68660,#68661,
#68662,#68663,#68664,#68665,#68666,#68667,#68668,#68669,#68670,#68671,#68672,
#68673,#68674,#68675,#68676,#68677,#68678,#68679,#68680,#68681,#68682,#68683,
#68684,#68685,#68686,#68687,#68688,#68689,#68690,#68691,#68692,#68693,#68694,
#68695,#68696,#68697,#68698,#68699,#68700,#68701,#68702,#68703,#68704,#68705,
#68706,#68707,#68708,#68709,#68710,#68711,#68712,#68713,#68714,#68715,#68716,
#68717,#68718,#68719,#68720,#68721,#68722,#68723,#68724,#68725,#68726,#68727,
#68728,#68729,#68730,#68731,#68732,#68733,#68734,#68735,#68736,#68737,#68738,
#68739,#68740,#68741,#68742,#68743,#68744,#68745,#68746,#68747,#68748,#68749,
#68750,#68751,#68752,#68753,#68754,#68755,#68756,#68757,#68758,#68759,#68760,
#68761,#68762,#68763,#68764,#68765,#68766,#68767,#68768,#68769,#68770,#68771,
#68772,#68773,#68774,#68775,#68776,#68777,#68778,#68779,#68780,#68781,#68782,
#68783,#68784,#68785,#68786,#68787,#68788,#68789,#68790,#68791,#68792,#68793,
#68794,#68795,#68796,#68797,#68798,#68799,#68800,#68801,#68802,#68803,#68804,
#68805,#68806,#68807,#68808,#68809,#68810,#68811,#68812,#68813,#68814,#68815,
#68816,#68817,#68818,#68819,#68820,#68821,#68822,#68823,#68824,#68825,#68826,
#68827,#68828,#68829,#68830,#68831,#68832,#68833,#68834,#68835,#68836,#68837,
#68838,#68839,#68840,#68841,#68842,#68843,#68844,#68845,#68846,#68847,#68848,
#68849,#68850,#68851,#68852,#68853,#68854,#68855,#68856,#68857,#68858,#68859,
#68860,#68861,#68862,#68863,#68864,#68865,#68866,#68867,#68868,#68869,#68870,
#68871,#68872,#68873,#68874,#68875,#68876,#68877,#68878,#68879,#68880,#68881,
#68882,#68883,#68884,#68885,#68886,#68887),(#68888,#68889,#68890,#68891,
#68892,#68893,#68894,#68895,#68896,#68897,#68898,#68899,#68900,#68901,#68902,
#68903,#68904,#68905,#68906,#68907,#68908,#68909,#68910,#68911,#68912,#68913,
#68914,#68915,#68916,#68917,#68918,#68919,#68920,#68921,#68922,#68923,#68924,
#68925,#68926,#68927,#68928,#68929,#68930,#68931,#68932,#68933,#68934,#68935,
#68936,#68937,#68938,#68939,#68940,#68941,#68942,#68943,#68944,#68945,#68946,
#68947,#68948,#68949,#68950,#68951,#68952,#68953,#68954,#68955,#68956,#68957,
#68958,#68959,#68960,#68961,#68962,#68963,#68964,#68965,#68966,#68967,#68968,
#68969,#68970,#68971,#68972,#68973,#68974,#68975,#68976,#68977,#68978,#68979,
#68980,#68981,#68982,#68983,#68984,#68985,#68986,#68987,#68988,#68989,#68990,
#68991,#68992,#68993,#68994,#68995,#68996,#68997,#68998,#68999,#69000,#69001,
#69002,#69003,#69004,#69005,#69006,#69007,#69008,#69009,#69010,#69011,#69012,
#69013,#69014,#69015,#69016,#69017,#69018,#69019,#69020,#69021,#69022,#69023,
#69024,#69025,#69026,#69027,#69028,#69029,#69030,#69031,#69032,#69033,#69034,
#69035,#69036,#69037,#69038,#69039,#69040,#69041,#69042,#69043,#69044,#69045,
#69046,#69047,#69048,#69049,#69050,#69051,#69052,#69053,#69054,#69055,#69056,
#69057,#69058,#69059,#69060,#69061,#69062,#69063,#69064,#69065,#69066,#69067,
#69068,#69069,#69070,#69071,#69072,#69073,#69074,#69075,#69076,#69077,#69078,
#69079,#69080,#69081,#69082,#69083,#69084,#69085,#69086,#69087,#69088,#69089,
#69090,#69091,#69092,#69093,#69094,#69095,#69096,#69097,#69098,#69099,#69100,
#69101,#69102,#69103,#69104,#69105,#69106,#69107,#69108,#69109,#69110,#69111,
#69112,#69113,#69114,#69115,#69116,#69117,#69118,#69119,#69120,#69121,#69122,
#69123,#69124,#69125,#69126,#69127,#69128,#69129,#69130,#69131,#69132,#69133,
#69134,#69135,#69136,#69137,#69138,#69139,#69140,#69141,#69142,#69143,#69144,
#69145,#69146,#69147,#69148,#69149,#69150,#69151,#69152,#69153,#69154,#69155,
#69156,#69157,#69158,#69159,#69160,#69161,#69162,#69163,#69164,#69165,#69166,
#69167,#69168,#69169,#69170,#69171,#69172,#69173,#69174,#69175,#69176,#69177,
#69178,#69179,#69180,#69181,#69182,#69183,#69184,#69185,#69186,#69187,#69188,
#69189,#69190,#69191,#69192,#69193,#69194,#69195,#69196,#69197,#69198,#69199,
#69200,#69201,#69202,#69203,#69204,#69205,#69206,#69207,#69208,#69209,#69210,
#69211,#69212,#69213,#69214,#69215,#69216,#69217,#69218,#69219,#69220,#69221,
#69222,#69223,#69224,#69225,#69226,#69227,#69228,#69229,#69230,#69231,#69232,
#69233,#69234,#69235,#69236,#69237,#69238,#69239,#69240,#69241,#69242,#69243,
#69244,#69245,#69246,#69247,#69248,#69249,#69250,#69251,#69252,#69253,#69254,
#69255,#69256,#69257,#69258,#69259,#69260,#69261,#69262,#69263,#69264,#69265,
#69266,#69267,#69268,#69269,#69270,#69271,#69272,#69273,#69274,#69275,#69276,
#69277,#69278,#69279,#69280,#69281,#69282,#69283,#69284,#69285,#69286,#69287,
#69288,#69289,#69290,#69291,#69292,#69293,#69294,#69295,#69296,#69297,#69298,
#69299,#69300,#69301,#69302,#69303,#69304,#69305,#69306,#69307,#69308,#69309,
#69310,#69311,#69312,#69313,#69314,#69315,#69316,#69317,#69318,#69319,#69320,
#69321,#69322,#69323,#69324,#69325,#69326,#69327,#69328,#69329,#69330,#69331,
#69332,#69333,#69334,#69335,#69336,#69337,#69338,#69339,#69340,#69341,#69342,
#69343,#69344,#69345,#69346,#69347,#69348,#69349,#69350,#69351,#69352,#69353,
#69354,#69355,#69356,#69357,#69358,#69359,#69360,#69361,#69362,#69363,#69364,
#69365,#69366,#69367,#69368,#69369,#69370,#69371,#69372,#69373,#69374,#69375,
#69376,#69377,#69378,#69379,#69380,#69381,#69382,#69383,#69384,#69385,#69386,
#69387,#69388,#69389,#69390,#69391,#69392,#69393,#69394,#69395,#69396,#69397,
#69398,#69399,#69400,#69401,#69402,#69403,#69404,#69405,#69406,#69407,#69408,
#69409,#69410,#69411,#69412,#69413,#69414,#69415,#69416,#69417,#69418,#69419,
#69420,#69421,#69422,#69423,#69424,#69425),(#69426,#69427,#69428,#69429,
#69430,#69431,#69432,#69433,#69434,#69435,#69436,#69437,#69438,#69439,#69440,
#69441,#69442,#69443,#69444,#69445,#69446,#69447,#69448,#69449,#69450,#69451,
#69452,#69453,#69454,#69455,#69456,#69457,#69458,#69459,#69460,#69461,#69462,
#69463,#69464,#69465,#69466,#69467,#69468,#69469,#69470,#69471,#69472,#69473,
#69474,#69475,#69476,#69477,#69478,#69479,#69480,#69481,#69482,#69483,#69484,
#69485,#69486,#69487,#69488,#69489,#69490,#69491,#69492,#69493,#69494,#69495,
#69496,#69497,#69498,#69499,#69500,#69501,#69502,#69503,#69504,#69505,#69506,
#69507,#69508,#69509,#69510,#69511,#69512,#69513,#69514,#69515,#69516,#69517,
#69518,#69519,#69520,#69521,#69522,#69523,#69524,#69525,#69526,#69527,#69528,
#69529,#69530,#69531,#69532,#69533,#69534,#69535,#69536,#69537,#69538,#69539,
#69540,#69541,#69542,#69543,#69544,#69545,#69546,#69547,#69548,#69549,#69550,
#69551,#69552,#69553,#69554,#69555,#69556,#69557,#69558,#69559,#69560,#69561,
#69562,#69563,#69564,#69565,#69566,#69567,#69568,#69569,#69570,#69571,#69572,
#69573,#69574,#69575,#69576,#69577,#69578,#69579,#69580,#69581,#69582,#69583,
#69584,#69585,#69586,#69587,#69588,#69589,#69590,#69591,#69592,#69593,#69594,
#69595,#69596,#69597,#69598,#69599,#69600,#69601,#69602,#69603,#69604,#69605,
#69606,#69607,#69608,#69609,#69610,#69611,#69612,#69613,#69614,#69615,#69616,
#69617,#69618,#69619,#69620,#69621,#69622,#69623,#69624,#69625,#69626,#69627,
#69628,#69629,#69630,#69631,#69632,#69633,#69634,#69635,#69636,#69637,#69638,
#69639,#69640,#69641,#69642,#69643,#69644,#69645,#69646,#69647,#69648,#69649,
#69650,#69651,#69652,#69653,#69654,#69655,#69656,#69657,#69658,#69659,#69660,
#69661,#69662,#69663,#69664,#69665,#69666,#69667,#69668,#69669,#69670,#69671,
#69672,#69673,#69674,#69675,#69676,#69677,#69678,#69679,#69680,#69681,#69682,
#69683,#69684,#69685,#69686,#69687,#69688,#69689,#69690,#69691,#69692,#69693,
#69694,#69695,#69696,#69697,#69698,#69699,#69700,#69701,#69702,#69703,#69704,
#69705,#69706,#69707,#69708,#69709,#69710,#69711,#69712,#69713,#69714,#69715,
#69716,#69717,#69718,#69719,#69720,#69721,#69722,#69723,#69724,#69725,#69726,
#69727,#69728,#69729,#69730,#69731,#69732,#69733,#69734,#69735,#69736,#69737,
#69738,#69739,#69740,#69741,#69742,#69743,#69744,#69745,#69746,#69747,#69748,
#69749,#69750,#69751,#69752,#69753,#69754,#69755,#69756,#69757,#69758,#69759,
#69760,#69761,#69762,#69763,#69764,#69765,#69766,#69767,#69768,#69769,#69770,
#69771,#69772,#69773,#69774,#69775,#69776,#69777,#69778,#69779,#69780,#69781,
#69782,#69783,#69784,#69785,#69786,#69787,#69788,#69789,#69790,#69791,#69792,
#69793,#69794,#69795,#69796,#69797,#69798,#69799,#69800,#69801,#69802,#69803,
#69804,#69805,#69806,#69807,#69808,#69809,#69810,#69811,#69812,#69813,#69814,
#69815,#69816,#69817,#69818,#69819,#69820,#69821,#69822,#69823,#69824,#69825,
#69826,#69827,#69828,#69829,#69830,#69831,#69832,#69833,#69834,#69835,#69836,
#69837,#69838,#69839,#69840,#69841,#69842,#69843,#69844,#69845,#69846,#69847,
#69848,#69849,#69850,#69851,#69852,#69853,#69854,#69855,#69856,#69857,#69858,
#69859,#69860,#69861,#69862,#69863,#69864,#69865,#69866,#69867,#69868,#69869,
#69870,#69871,#69872,#69873,#69874,#69875,#69876,#69877,#69878,#69879,#69880,
#69881,#69882,#69883,#69884,#69885,#69886,#69887,#69888,#69889,#69890,#69891,
#69892,#69893,#69894,#69895,#69896,#69897,#69898,#69899,#69900,#69901,#69902,
#69903,#69904,#69905,#69906,#69907,#69908,#69909,#69910,#69911,#69912,#69913,
#69914,#69915,#69916,#69917,#69918,#69919,#69920,#69921,#69922,#69923,#69924,
#69925,#69926,#69927,#69928,#69929,#69930,#69931,#69932,#69933,#69934,#69935,
#69936,#69937,#69938,#69939,#69940,#69941,#69942,#69943,#69944,#69945,#69946,
#69947,#69948,#69949,#69950,#69951,#69952,#69953,#69954,#69955,#69956,#69957,
#69958,#69959,#69960,#69961,#69962,#69963),(#69964,#69965,#69966,#69967,
#69968,#69969,#69970,#69971,#69972,#69973,#69974,#69975,#69976,#69977,#69978,
#69979,#69980,#69981,#69982,#69983,#69984,#69985,#69986,#69987,#69988,#69989,
#69990,#69991,#69992,#69993,#69994,#69995,#69996,#69997,#69998,#69999,#70000,
#70001,#70002,#70003,#70004,#70005,#70006,#70007,#70008,#70009,#70010,#70011,
#70012,#70013,#70014,#70015,#70016,#70017,#70018,#70019,#70020,#70021,#70022,
#70023,#70024,#70025,#70026,#70027,#70028,#70029,#70030,#70031,#70032,#70033,
#70034,#70035,#70036,#70037,#70038,#70039,#70040,#70041,#70042,#70043,#70044,
#70045,#70046,#70047,#70048,#70049,#70050,#70051,#70052,#70053,#70054,#70055,
#70056,#70057,#70058,#70059,#70060,#70061,#70062,#70063,#70064,#70065,#70066,
#70067,#70068,#70069,#70070,#70071,#70072,#70073,#70074,#70075,#70076,#70077,
#70078,#70079,#70080,#70081,#70082,#70083,#70084,#70085,#70086,#70087,#70088,
#70089,#70090,#70091,#70092,#70093,#70094,#70095,#70096,#70097,#70098,#70099,
#70100,#70101,#70102,#70103,#70104,#70105,#70106,#70107,#70108,#70109,#70110,
#70111,#70112,#70113,#70114,#70115,#70116,#70117,#70118,#70119,#70120,#70121,
#70122,#70123,#70124,#70125,#70126,#70127,#70128,#70129,#70130,#70131,#70132,
#70133,#70134,#70135,#70136,#70137,#70138,#70139,#70140,#70141,#70142,#70143,
#70144,#70145,#70146,#70147,#70148,#70149,#70150,#70151,#70152,#70153,#70154,
#70155,#70156,#70157,#70158,#70159,#70160,#70161,#70162,#70163,#70164,#70165,
#70166,#70167,#70168,#70169,#70170,#70171,#70172,#70173,#70174,#70175,#70176,
#70177,#70178,#70179,#70180,#70181,#70182,#70183,#70184,#70185,#70186,#70187,
#70188,#70189,#70190,#70191,#70192,#70193,#70194,#70195,#70196,#70197,#70198,
#70199,#70200,#70201,#70202,#70203,#70204,#70205,#70206,#70207,#70208,#70209,
#70210,#70211,#70212,#70213,#70214,#70215,#70216,#70217,#70218,#70219,#70220,
#70221,#70222,#70223,#70224,#70225,#70226,#70227,#70228,#70229,#70230,#70231,
#70232,#70233,#70234,#70235,#70236,#70237,#70238,#70239,#70240,#70241,#70242,
#70243,#70244,#70245,#70246,#70247,#70248,#70249,#70250,#70251,#70252,#70253,
#70254,#70255,#70256,#70257,#70258,#70259,#70260,#70261,#70262,#70263,#70264,
#70265,#70266,#70267,#70268,#70269,#70270,#70271,#70272,#70273,#70274,#70275,
#70276,#70277,#70278,#70279,#70280,#70281,#70282,#70283,#70284,#70285,#70286,
#70287,#70288,#70289,#70290,#70291,#70292,#70293,#70294,#70295,#70296,#70297,
#70298,#70299,#70300,#70301,#70302,#70303,#70304,#70305,#70306,#70307,#70308,
#70309,#70310,#70311,#70312,#70313,#70314,#70315,#70316,#70317,#70318,#70319,
#70320,#70321,#70322,#70323,#70324,#70325,#70326,#70327,#70328,#70329,#70330,
#70331,#70332,#70333,#70334,#70335,#70336,#70337,#70338,#70339,#70340,#70341,
#70342,#70343,#70344,#70345,#70346,#70347,#70348,#70349,#70350,#70351,#70352,
#70353,#70354,#70355,#70356,#70357,#70358,#70359,#70360,#70361,#70362,#70363,
#70364,#70365,#70366,#70367,#70368,#70369,#70370,#70371,#70372,#70373,#70374,
#70375,#70376,#70377,#70378,#70379,#70380,#70381,#70382,#70383,#70384,#70385,
#70386,#70387,#70388,#70389,#70390,#70391,#70392,#70393,#70394,#70395,#70396,
#70397,#70398,#70399,#70400,#70401,#70402,#70403,#70404,#70405,#70406,#70407,
#70408,#70409,#70410,#70411,#70412,#70413,#70414,#70415,#70416,#70417,#70418,
#70419,#70420,#70421,#70422,#70423,#70424,#70425,#70426,#70427,#70428,#70429,
#70430,#70431,#70432,#70433,#70434,#70435,#70436,#70437,#70438,#70439,#70440,
#70441,#70442,#70443,#70444,#70445,#70446,#70447,#70448,#70449,#70450,#70451,
#70452,#70453,#70454,#70455,#70456,#70457,#70458,#70459,#70460,#70461,#70462,
#70463,#70464,#70465,#70466,#70467,#70468,#70469,#70470,#70471,#70472,#70473,
#70474,#70475,#70476,#70477,#70478,#70479,#70480,#70481,#70482,#70483,#70484,
#70485,#70486,#70487,#70488,#70489,#70490,#70491,#70492,#70493,#70494,#70495,
#70496,#70497,#70498,#70499,#70500,#70501)),.UNSPECIFIED.,.F.,.F.,.F.,(4,
4),(4,1,1,1,1,1,1,1,1,1,1,1,1,1,1,1,1,1,1,1,1,1,1,1,1,1,1,1,1,1,1,1,1,1,
1,1,1,1,1,1,1,1,1,1,1,1,1,1,1,1,1,1,1,1,1,1,1,1,1,1,1,1,1,1,1,1,1,1,1,1,
1,1,1,1,1,1,1,1,1,1,1,1,1,1,1,1,1,1,1,1,1,1,1,1,1,1,1,1,1,1,1,1,1,1,1,1,
1,1,1,1,1,1,1,1,1,1,1,1,1,1,1,1,1,1,1,1,1,1,1,1,1,1,1,1,1,1,1,1,1,1,1,1,
1,1,1,1,1,1,1,1,1,1,1,1,1,1,1,1,1,1,1,1,1,1,1,1,1,1,1,1,1,1,1,1,1,1,1,1,
1,1,1,1,1,1,1,1,1,1,1,1,1,1,1,1,1,1,1,1,1,1,1,1,1,1,1,1,1,1,1,1,1,1,1,1,
1,1,1,1,1,1,1,1,1,1,1,1,1,1,1,1,1,1,1,1,1,1,1,1,1,1,1,1,1,1,1,1,1,1,1,1,
1,1,1,1,1,1,1,1,1,1,1,1,1,1,1,1,1,1,1,1,1,1,1,1,1,1,1,1,1,1,1,1,1,1,1,1,
1,1,1,1,1,1,1,1,1,1,1,1,1,1,1,1,1,1,1,1,1,1,1,1,1,1,1,1,1,1,1,1,1,1,1,1,
1,1,1,1,1,1,1,1,1,1,1,1,1,1,1,1,1,1,1,1,1,1,1,1,1,1,1,1,1,1,1,1,1,1,1,1,
1,1,1,1,1,1,1,1,1,1,1,1,1,1,1,1,1,1,1,1,1,1,1,1,1,1,1,1,1,1,1,1,1,1,1,1,
1,1,1,1,1,1,1,1,1,1,1,1,1,1,1,1,1,1,1,1,1,1,1,1,1,1,1,1,1,1,1,1,1,1,1,1,
1,1,1,1,1,1,1,1,1,1,1,1,1,1,1,1,1,1,1,1,1,1,1,1,1,1,1,1,1,1,1,1,1,1,1,1,
1,1,1,1,1,1,1,1,1,1,1,1,1,1,1,1,1,1,1,1,1,1,1,1,1,1,1,1,1,1,1,1,1,1,1,1,
1,1,1,1,1,1,1,1,1,1,1,1,1,1,1,1,1,1,1,1,1,1,1,1,1,1,1,1,1,1,1,1,1,4),(0.,
0.132097741590587),(11.6150328478189,12.1141250590241,12.6132172702293,
13.1123094814345,13.6114016926397,14.60958611505,15.6077705374604,16.6059549598707,
17.1050471710759,17.6041393822811,18.1032315934863,18.6023238046915,19.6005082271018,
20.099600438307,20.5986926495122,21.5968770719225,22.5950614943329,23.5932459167433,
24.0923381279484,24.5914303391536,25.0905225503588,25.589614761564,26.5877991839743,
27.0868913951795,27.5859836063847,28.5841680287951,29.5823524512054,30.5805368736158,
31.079629084821,31.5787212960261,32.0778135072313,32.5769057184365,33.5750901408469,
34.074182352052,34.5732745632572,35.5714589856676,36.569643408078,37.5678278304883,
38.0669200416935,38.5660122528987,39.0651044641039,39.564196675309,40.5623810977194,
41.0614733089246,41.5605655201297,42.5587499425401,43.5569343649505,44.5551187873608,
45.054210998566,45.5533032097712,46.0523954209764,46.5514876321816,47.5496720545919,
48.0487642657971,48.5478564770023,49.5460408994126,50.544225321823,51.5424097442334,
52.0415019554385,52.5405941666437,53.0396863778489,53.5387785890541,54.5369630114644,
55.0360552226696,55.5351474338748,56.5333318562852,57.5315162786955,58.5297007011059,
59.0287929123111,59.5278851235162,60.0269773347214,60.5260695459266,61.524253968337,
62.0233461795421,62.5224383907473,63.5206228131577,64.518807235568,65.5169916579784,
66.0160838691836,66.5151760803888,67.0142682915939,67.5133605027991,68.5115449252095,
69.0106371364147,69.5097293476198,70.5079137700302,71.5060981924406,72.5042826148509,
73.0033748260561,73.5024670372613,74.0015592484665,74.5006514596716,75.498835882082,
75.9979280932872,76.4970203044924,77.4952047269027,78.4933891493131,79.4915735717234,
79.9906657829286,80.4897579941338,80.988850205339,81.4879424165442,82.4861268389545,
82.9852190501597,83.4843112613649,84.4824956837752,85.4806801061856,86.4788645285959,
86.9779567398011,87.4770489510063,87.9761411622115,88.4752333734167,89.473417795827,
89.9725100070322,90.4716022182374,91.4697866406478,92.4679710630581,93.4661554854685,
93.9652476966737,94.4643399078788,94.963432119084,95.4625243302892,96.4607087526996,
96.9598009639047,97.4588931751099,98.4570775975203,99.4552620199306,100.453446442341,
100.952538653546,101.451630864751,101.950723075957,102.449815287162,103.447999709572,
103.947091920777,104.446184131982,105.444368554393,106.442552976803,107.440737399214,
107.939829610419,108.438921821624,108.938014032829,109.437106244034,110.435290666445,
110.93438287765,111.433475088855,112.431659511265,113.429843933676,114.428028356086,
114.927120567291,115.426212778496,115.925304989702,116.424397200907,117.422581623317,
117.921673834522,118.420766045727,119.418950468138,120.417134890548,121.415319312959,
121.914411524164,122.413503735369,122.912595946574,123.411688157779,124.40987258019,
124.908964791395,125.4080570026,126.40624142501,127.404425847421,128.402610269831,
128.901702481036,129.400794692241,129.899886903447,130.398979114652,131.397163537062,
131.896255748267,132.395347959473,133.393532381883,134.391716804293,135.389901226704,
135.888993437909,136.388085649114,136.887177860319,137.386270071524,138.384454493935,
138.88354670514,139.382638916345,140.380823338755,141.379007761166,142.377192183576,
142.876284394781,143.375376605987,143.874468817192,144.373561028397,145.371745450807,
145.870837662012,146.369929873218,147.368114295628,148.366298718038,149.364483140449,
149.863575351654,150.362667562859,150.861759774064,151.360851985269,152.35903640768,
152.858128618885,153.35722083009,154.3554052525,155.353589674911,156.351774097321,
156.850866308526,157.349958519732,157.849050730937,158.348142942142,159.346327364552,
159.845419575757,160.344511786963,161.342696209373,162.340880631783,163.339065054194,
163.838157265399,164.337249476604,164.836341687809,165.335433899014,166.333618321425,
166.83271053263,167.331802743835,168.329987166246,169.328171588656,170.326356011066,
170.825448222271,171.324540433477,171.823632644682,172.322724855887,173.320909278297,
173.820001489502,174.319093700708,175.317278123118,176.315462545528,177.313646967939,
177.812739179144,178.311831390349,178.810923601554,179.310015812759,180.30820023517,
180.807292446375,181.30638465758,182.304569079991,183.302753502401,184.300937924811,
184.800030136016,185.299122347222,185.798214558427,186.297306769632,187.295491192042,
187.794583403248,188.293675614453,189.291860036863,190.290044459273,191.288228881684,
191.787321092889,192.286413304094,192.785505515299,193.284597726505,194.282782148915,
194.78187436012,195.280966571325,196.279150993736,197.277335416146,198.275519838556,
199.273704260967,200.271888683377,201.270073105787,202.268257528198,202.767349739403,
203.266441950608,204.264626373018,204.763718584224,205.262810795429,205.761903006634,
206.260995217839,207.25917964025,208.25736406266,209.25554848507,209.754640696275,
210.253732907481,211.251917329891,211.751009541096,212.250101752301,212.749193963507,
213.248286174712,214.246470597122,215.244655019532,216.242839441943,216.741931653148,
217.241023864353,218.239208286764,218.738300497969,219.237392709174,219.736484920379,
220.235577131584,221.233761553995,222.231945976405,223.230130398815,223.72922261002,
224.228314821226,225.226499243636,225.725591454841,226.224683666046,226.723775877252,
227.222868088457,228.221052510867,229.219236933277,230.217421355688,230.716513566893,
231.215605778098,232.213790200509,232.712882411714,233.211974622919,233.711066834124,
234.210159045329,235.20834346774,236.20652789015,237.20471231256,237.703804523766,
238.202896734971,239.201081157381,239.700173368586,240.199265579791,240.698357790997,
241.197450002202,242.195634424612,243.193818847023,244.192003269433,244.691095480638,
245.190187691843,246.188372114254,246.687464325459,247.186556536664,247.685648747869,
248.184740959074,249.182925381485,250.181109803895,251.179294226305,251.678386437511,
252.177478648716,253.175663071126,253.674755282331,254.173847493536,254.672939704742,
255.172031915947,256.170216338357,257.168400760768,258.166585183178,258.665677394383,
259.164769605588,260.162954027999,260.662046239204,261.161138450409,261.660230661614,
262.159322872819,263.15750729523,264.15569171764,265.15387614005,265.652968351256,
266.152060562461,267.150244984871,267.649337196076,268.148429407282,268.647521618487,
269.146613829692,270.144798252102,271.142982674513,272.141167096923,272.640259308128,
273.139351519333,274.137535941744,274.636628152949,275.135720364154,275.634812575359,
276.133904786564,277.132089208975,278.130273631385,279.128458053795,279.627550265001,
280.126642476206,281.124826898616,281.623919109821,282.123011321027,282.622103532232,
283.121195743437,284.119380165847,285.117564588258,286.115749010668,286.614841221873,
287.113933433078,288.112117855489,288.611210066694,289.110302277899,289.609394489104,
290.108486700309,291.10667112272,292.10485554513,293.103039967541,293.602132178746,
294.101224389951,295.099408812361,295.598501023566,296.097593234772,296.596685445977,
297.095777657182,298.093962079592,299.092146502003,300.090330924413,300.589423135618,
301.088515346823,302.086699769234,302.585791980439,303.084884191644,303.583976402849,
304.083068614054,305.081253036465,306.079437458875,307.077621881286,307.576714092491,
308.075806303696,309.073990726106,309.573082937311,310.072175148517,310.571267359722,
311.070359570927,312.068543993337,313.066728415748,314.064912838158,314.564005049363,
315.063097260568,316.061281682979,316.560373894184,317.059466105389,317.558558316594,
318.0576505278,319.05583495021,320.05401937262,321.052203795031,321.551296006236,
322.050388217441,323.048572639851,323.547664851057,324.046757062262,324.545849273467,
325.044941484672,326.043125907082,327.041310329493,328.039494751903,328.538586963108,
329.037679174313,330.035863596724,330.534955807929,331.034048019134,331.533140230339,
332.032232441545,333.030416863955,334.028601286365,335.026785708776,335.525877919981,
336.024970131186,337.023154553596,337.522246764802,338.021338976007,338.520431187212,
339.019523398417,340.017707820827,341.015892243238,342.014076665648,342.513168876853,
343.012261088059,344.010445510469,344.509537721674,345.008629932879,345.507722144084,
346.00681435529,347.0049987777,348.00318320011,349.001367622521,349.500459833726,
349.999552044931,350.997736467341,351.496828678547,351.995920889752,352.495013100957,
352.994105312162,353.992289734573,354.990474156983,355.988658579393,356.487750790598,
356.986843001804,357.985027424214,358.484119635419,358.983211846624,359.48230405783,
359.981396269035,360.979580691445,361.977765113855,362.975949536266,363.475041747471,
363.974133958676,364.972318381086,365.471410592292,365.970502803497,366.469595014702,
366.968687225907,367.966871648318,368.965056070728,369.963240493138,370.462332704343,
370.961424915549,371.959609337959,372.458701549164,372.957793760369,373.456885971574,
373.95597818278,374.95416260519,375.9523470276,376.950531450011,377.449623661216,
377.948715872421,378.946900294831,379.445992506037,379.945084717242,380.444176928447,
380.943269139652,381.941453562063,382.939637984473,383.937822406883,384.436914618089,
384.936006829294,385.435099040499,385.934191251704),.UNSPECIFIED.);
#1709=CYLINDRICAL_SURFACE('',#30285,0.7911);
#1710=CYLINDRICAL_SURFACE('',#30287,0.7911);
#1711=CYLINDRICAL_SURFACE('',#30288,0.7911);
#1712=CYLINDRICAL_SURFACE('',#30289,0.7911);
#1713=CYLINDRICAL_SURFACE('',#30290,0.7911);
#1714=CYLINDRICAL_SURFACE('',#30291,0.7911);
#1715=CYLINDRICAL_SURFACE('',#30292,0.7911);
#1716=CYLINDRICAL_SURFACE('',#30293,0.7911);
#1717=CYLINDRICAL_SURFACE('',#30294,0.7911);
#1718=CYLINDRICAL_SURFACE('',#30295,0.7911);
#1719=CYLINDRICAL_SURFACE('',#30296,0.7911);
#1720=CYLINDRICAL_SURFACE('',#30297,0.7911);
#1721=CYLINDRICAL_SURFACE('',#30298,0.7911);
#1722=CYLINDRICAL_SURFACE('',#30299,0.7911);
#1723=CYLINDRICAL_SURFACE('',#30300,0.7911);
#1724=CYLINDRICAL_SURFACE('',#30301,0.7911);
#1725=CYLINDRICAL_SURFACE('',#30302,0.7911);
#1726=CYLINDRICAL_SURFACE('',#30303,0.7911);
#1727=CYLINDRICAL_SURFACE('',#30304,0.7911);
#1728=CYLINDRICAL_SURFACE('',#30305,0.7911);
#1729=CYLINDRICAL_SURFACE('',#30306,0.7911);
#1730=CYLINDRICAL_SURFACE('',#30307,0.7911);
#1731=CYLINDRICAL_SURFACE('',#30308,0.7911);
#1732=CYLINDRICAL_SURFACE('',#30309,0.7911);
#1733=CYLINDRICAL_SURFACE('',#30310,0.7911);
#1734=CYLINDRICAL_SURFACE('',#30311,0.7911);
#1735=CYLINDRICAL_SURFACE('',#30312,0.7911);
#1736=CYLINDRICAL_SURFACE('',#30313,0.7911);
#1737=CYLINDRICAL_SURFACE('',#30314,0.7911);
#1738=CYLINDRICAL_SURFACE('',#30315,0.7911);
#1739=CYLINDRICAL_SURFACE('',#30316,0.7911);
#1740=CYLINDRICAL_SURFACE('',#30317,0.7911);
#1741=CYLINDRICAL_SURFACE('',#30318,0.7911);
#1742=CYLINDRICAL_SURFACE('',#30319,0.7911);
#1743=CYLINDRICAL_SURFACE('',#30320,0.7911);
#1744=CYLINDRICAL_SURFACE('',#30321,0.7911);
#1745=CYLINDRICAL_SURFACE('',#30322,0.7911);
#1746=CYLINDRICAL_SURFACE('',#30323,0.7911);
#1747=CYLINDRICAL_SURFACE('',#30324,0.7911);
#1748=CYLINDRICAL_SURFACE('',#30325,0.7911);
#1749=CYLINDRICAL_SURFACE('',#30326,0.7911);
#1750=CYLINDRICAL_SURFACE('',#30327,0.7911);
#1751=CYLINDRICAL_SURFACE('',#30328,0.7911);
#1752=CYLINDRICAL_SURFACE('',#30329,0.7911);
#1753=CYLINDRICAL_SURFACE('',#30330,0.7911);
#1754=CYLINDRICAL_SURFACE('',#30331,0.7911);
#1755=CYLINDRICAL_SURFACE('',#30332,0.7911);
#1756=CYLINDRICAL_SURFACE('',#30333,0.7911);
#1757=CYLINDRICAL_SURFACE('',#30334,0.7911);
#1758=CYLINDRICAL_SURFACE('',#30335,0.7911);
#1759=CYLINDRICAL_SURFACE('',#30336,0.7911);
#1760=CYLINDRICAL_SURFACE('',#30337,0.7911);
#1761=CYLINDRICAL_SURFACE('',#30338,0.7911);
#1762=CYLINDRICAL_SURFACE('',#30339,0.7911);
#1763=CYLINDRICAL_SURFACE('',#30340,0.7911);
#1764=CYLINDRICAL_SURFACE('',#30341,0.7911);
#1765=CYLINDRICAL_SURFACE('',#30342,0.7911);
#1766=CYLINDRICAL_SURFACE('',#30343,0.7911);
#1767=CYLINDRICAL_SURFACE('',#30344,0.7911);
#1768=CYLINDRICAL_SURFACE('',#30345,0.7911);
#1769=CYLINDRICAL_SURFACE('',#30347,0.6767);
#1770=CYLINDRICAL_SURFACE('',#30349,0.6767);
#1771=CYLINDRICAL_SURFACE('',#30350,0.6767);
#1772=CYLINDRICAL_SURFACE('',#30351,0.6767);
#1773=CYLINDRICAL_SURFACE('',#30352,0.6767);
#1774=CYLINDRICAL_SURFACE('',#30353,0.6767);
#1775=CYLINDRICAL_SURFACE('',#30354,0.6767);
#1776=CYLINDRICAL_SURFACE('',#30355,0.6767);
#1777=CYLINDRICAL_SURFACE('',#30356,0.6767);
#1778=CYLINDRICAL_SURFACE('',#30357,0.6767);
#1779=CYLINDRICAL_SURFACE('',#30358,0.6767);
#1780=CYLINDRICAL_SURFACE('',#30359,0.6767);
#1781=CYLINDRICAL_SURFACE('',#30360,0.6767);
#1782=CYLINDRICAL_SURFACE('',#30361,0.6767);
#1783=CYLINDRICAL_SURFACE('',#30362,0.6767);
#1784=CYLINDRICAL_SURFACE('',#30363,0.6767);
#1785=CYLINDRICAL_SURFACE('',#30364,0.6767);
#1786=CYLINDRICAL_SURFACE('',#30365,0.6767);
#1787=CYLINDRICAL_SURFACE('',#30366,0.6767);
#1788=CYLINDRICAL_SURFACE('',#30367,0.6767);
#1789=CYLINDRICAL_SURFACE('',#30368,0.6767);
#1790=CYLINDRICAL_SURFACE('',#30369,0.6767);
#1791=CYLINDRICAL_SURFACE('',#30370,0.6767);
#1792=CYLINDRICAL_SURFACE('',#30371,0.6767);
#1793=CYLINDRICAL_SURFACE('',#30372,0.6767);
#1794=CYLINDRICAL_SURFACE('',#30373,0.6767);
#1795=CYLINDRICAL_SURFACE('',#30374,0.6767);
#1796=CYLINDRICAL_SURFACE('',#30375,0.6767);
#1797=CYLINDRICAL_SURFACE('',#30376,0.6767);
#1798=CYLINDRICAL_SURFACE('',#30377,0.6767);
#1799=CYLINDRICAL_SURFACE('',#30378,0.6767);
#1800=CYLINDRICAL_SURFACE('',#30379,0.6767);
#1801=CYLINDRICAL_SURFACE('',#30380,0.6767);
#1802=CYLINDRICAL_SURFACE('',#30381,0.6767);
#1803=CYLINDRICAL_SURFACE('',#30382,0.6767);
#1804=CYLINDRICAL_SURFACE('',#30383,0.6767);
#1805=CYLINDRICAL_SURFACE('',#30384,0.6767);
#1806=CYLINDRICAL_SURFACE('',#30385,0.6767);
#1807=CYLINDRICAL_SURFACE('',#30386,0.6767);
#1808=CYLINDRICAL_SURFACE('',#30387,0.6767);
#1809=CYLINDRICAL_SURFACE('',#30388,0.6767);
#1810=CYLINDRICAL_SURFACE('',#30389,0.6767);
#1811=CYLINDRICAL_SURFACE('',#30390,0.6767);
#1812=CYLINDRICAL_SURFACE('',#30391,0.6767);
#1813=CYLINDRICAL_SURFACE('',#30392,0.6767);
#1814=CYLINDRICAL_SURFACE('',#30393,0.6767);
#1815=CYLINDRICAL_SURFACE('',#30394,0.6767);
#1816=CYLINDRICAL_SURFACE('',#30395,0.6767);
#1817=CYLINDRICAL_SURFACE('',#30396,0.6767);
#1818=CYLINDRICAL_SURFACE('',#30397,0.6767);
#1819=CYLINDRICAL_SURFACE('',#30398,0.6767);
#1820=CYLINDRICAL_SURFACE('',#30399,0.6767);
#1821=CYLINDRICAL_SURFACE('',#30400,0.6767);
#1822=CYLINDRICAL_SURFACE('',#30401,0.6767);
#1823=CYLINDRICAL_SURFACE('',#30402,0.6767);
#1824=CYLINDRICAL_SURFACE('',#30403,0.6767);
#1825=CYLINDRICAL_SURFACE('',#30404,0.6767);
#1826=CYLINDRICAL_SURFACE('',#30405,0.6767);
#1827=CYLINDRICAL_SURFACE('',#30406,0.6767);
#1828=CYLINDRICAL_SURFACE('',#30425,0.6767);
#1829=CYLINDRICAL_SURFACE('',#30431,0.7911);
#1976=FACE_BOUND('',#5998,.T.);
#1977=FACE_BOUND('',#5999,.T.);
#1978=FACE_BOUND('',#6039,.T.);
#1979=FACE_BOUND('',#6040,.T.);
#1980=FACE_BOUND('',#6052,.T.);
#1981=FACE_BOUND('',#6062,.T.);
#1982=FACE_BOUND('',#6063,.T.);
#1983=FACE_BOUND('',#6064,.T.);
#2550=CIRCLE('',#30286,0.7911);
#2551=CIRCLE('',#30346,0.7911);
#2552=CIRCLE('',#30348,0.6767);
#2553=CIRCLE('',#30419,0.7911);
#2554=CIRCLE('',#30420,0.7911);
#2555=CIRCLE('',#30422,0.7911);
#2556=CIRCLE('',#30423,0.7911);
#2557=CIRCLE('',#30424,0.6767);
#2558=CIRCLE('',#30427,0.8511);
#2559=CIRCLE('',#30428,0.06);
#2560=CIRCLE('',#30429,0.7911);
#2561=CIRCLE('',#30433,1.14);
#2562=CIRCLE('',#30442,0.7);
#2893=CONICAL_SURFACE('',#30432,1.28782032302755,1.0471975511966);
#2894=CONICAL_SURFACE('',#30443,0.75,0.785398163397451);
#4163=FACE_OUTER_BOUND('',#5845,.T.);
#4164=FACE_OUTER_BOUND('',#5846,.T.);
#4165=FACE_OUTER_BOUND('',#5847,.T.);
#4166=FACE_OUTER_BOUND('',#5848,.T.);
#4167=FACE_OUTER_BOUND('',#5849,.T.);
#4168=FACE_OUTER_BOUND('',#5850,.T.);
#4169=FACE_OUTER_BOUND('',#5851,.T.);
#4170=FACE_OUTER_BOUND('',#5852,.T.);
#4171=FACE_OUTER_BOUND('',#5853,.T.);
#4172=FACE_OUTER_BOUND('',#5854,.T.);
#4173=FACE_OUTER_BOUND('',#5855,.T.);
#4174=FACE_OUTER_BOUND('',#5856,.T.);
#4175=FACE_OUTER_BOUND('',#5857,.T.);
#4176=FACE_OUTER_BOUND('',#5858,.T.);
#4177=FACE_OUTER_BOUND('',#5859,.T.);
#4178=FACE_OUTER_BOUND('',#5860,.T.);
#4179=FACE_OUTER_BOUND('',#5861,.T.);
#4180=FACE_OUTER_BOUND('',#5862,.T.);
#4181=FACE_OUTER_BOUND('',#5863,.T.);
#4182=FACE_OUTER_BOUND('',#5864,.T.);
#4183=FACE_OUTER_BOUND('',#5865,.T.);
#4184=FACE_OUTER_BOUND('',#5866,.T.);
#4185=FACE_OUTER_BOUND('',#5867,.T.);
#4186=FACE_OUTER_BOUND('',#5868,.T.);
#4187=FACE_OUTER_BOUND('',#5869,.T.);
#4188=FACE_OUTER_BOUND('',#5870,.T.);
#4189=FACE_OUTER_BOUND('',#5871,.T.);
#4190=FACE_OUTER_BOUND('',#5872,.T.);
#4191=FACE_OUTER_BOUND('',#5873,.T.);
#4192=FACE_OUTER_BOUND('',#5874,.T.);
#4193=FACE_OUTER_BOUND('',#5875,.T.);
#4194=FACE_OUTER_BOUND('',#5876,.T.);
#4195=FACE_OUTER_BOUND('',#5877,.T.);
#4196=FACE_OUTER_BOUND('',#5878,.T.);
#4197=FACE_OUTER_BOUND('',#5879,.T.);
#4198=FACE_OUTER_BOUND('',#5880,.T.);
#4199=FACE_OUTER_BOUND('',#5881,.T.);
#4200=FACE_OUTER_BOUND('',#5882,.T.);
#4201=FACE_OUTER_BOUND('',#5883,.T.);
#4202=FACE_OUTER_BOUND('',#5884,.T.);
#4203=FACE_OUTER_BOUND('',#5885,.T.);
#4204=FACE_OUTER_BOUND('',#5886,.T.);
#4205=FACE_OUTER_BOUND('',#5887,.T.);
#4206=FACE_OUTER_BOUND('',#5888,.T.);
#4207=FACE_OUTER_BOUND('',#5889,.T.);
#4208=FACE_OUTER_BOUND('',#5890,.T.);
#4209=FACE_OUTER_BOUND('',#5891,.T.);
#4210=FACE_OUTER_BOUND('',#5892,.T.);
#4211=FACE_OUTER_BOUND('',#5893,.T.);
#4212=FACE_OUTER_BOUND('',#5894,.T.);
#4213=FACE_OUTER_BOUND('',#5895,.T.);
#4214=FACE_OUTER_BOUND('',#5896,.T.);
#4215=FACE_OUTER_BOUND('',#5897,.T.);
#4216=FACE_OUTER_BOUND('',#5898,.T.);
#4217=FACE_OUTER_BOUND('',#5899,.T.);
#4218=FACE_OUTER_BOUND('',#5900,.T.);
#4219=FACE_OUTER_BOUND('',#5901,.T.);
#4220=FACE_OUTER_BOUND('',#5902,.T.);
#4221=FACE_OUTER_BOUND('',#5903,.T.);
#4222=FACE_OUTER_BOUND('',#5904,.T.);
#4223=FACE_OUTER_BOUND('',#5905,.T.);
#4224=FACE_OUTER_BOUND('',#5906,.T.);
#4225=FACE_OUTER_BOUND('',#5907,.T.);
#4226=FACE_OUTER_BOUND('',#5908,.T.);
#4227=FACE_OUTER_BOUND('',#5909,.T.);
#4228=FACE_OUTER_BOUND('',#5910,.T.);
#4229=FACE_OUTER_BOUND('',#5911,.T.);
#4230=FACE_OUTER_BOUND('',#5912,.T.);
#4231=FACE_OUTER_BOUND('',#5913,.T.);
#4232=FACE_OUTER_BOUND('',#5914,.T.);
#4233=FACE_OUTER_BOUND('',#5915,.T.);
#4234=FACE_OUTER_BOUND('',#5916,.T.);
#4235=FACE_OUTER_BOUND('',#5917,.T.);
#4236=FACE_OUTER_BOUND('',#5918,.T.);
#4237=FACE_OUTER_BOUND('',#5919,.T.);
#4238=FACE_OUTER_BOUND('',#5920,.T.);
#4239=FACE_OUTER_BOUND('',#5921,.T.);
#4240=FACE_OUTER_BOUND('',#5922,.T.);
#4241=FACE_OUTER_BOUND('',#5923,.T.);
#4242=FACE_OUTER_BOUND('',#5924,.T.);
#4243=FACE_OUTER_BOUND('',#5925,.T.);
#4244=FACE_OUTER_BOUND('',#5926,.T.);
#4245=FACE_OUTER_BOUND('',#5927,.T.);
#4246=FACE_OUTER_BOUND('',#5928,.T.);
#4247=FACE_OUTER_BOUND('',#5929,.T.);
#4248=FACE_OUTER_BOUND('',#5930,.T.);
#4249=FACE_OUTER_BOUND('',#5931,.T.);
#4250=FACE_OUTER_BOUND('',#5932,.T.);
#4251=FACE_OUTER_BOUND('',#5933,.T.);
#4252=FACE_OUTER_BOUND('',#5934,.T.);
#4253=FACE_OUTER_BOUND('',#5935,.T.);
#4254=FACE_OUTER_BOUND('',#5936,.T.);
#4255=FACE_OUTER_BOUND('',#5937,.T.);
#4256=FACE_OUTER_BOUND('',#5938,.T.);
#4257=FACE_OUTER_BOUND('',#5939,.T.);
#4258=FACE_OUTER_BOUND('',#5940,.T.);
#4259=FACE_OUTER_BOUND('',#5941,.T.);
#4260=FACE_OUTER_BOUND('',#5942,.T.);
#4261=FACE_OUTER_BOUND('',#5943,.T.);
#4262=FACE_OUTER_BOUND('',#5944,.T.);
#4263=FACE_OUTER_BOUND('',#5945,.T.);
#4264=FACE_OUTER_BOUND('',#5946,.T.);
#4265=FACE_OUTER_BOUND('',#5947,.T.);
#4266=FACE_OUTER_BOUND('',#5948,.T.);
#4267=FACE_OUTER_BOUND('',#5949,.T.);
#4268=FACE_OUTER_BOUND('',#5950,.T.);
#4269=FACE_OUTER_BOUND('',#5951,.T.);
#4270=FACE_OUTER_BOUND('',#5952,.T.);
#4271=FACE_OUTER_BOUND('',#5953,.T.);
#4272=FACE_OUTER_BOUND('',#5954,.T.);
#4273=FACE_OUTER_BOUND('',#5955,.T.);
#4274=FACE_OUTER_BOUND('',#5956,.T.);
#4275=FACE_OUTER_BOUND('',#5957,.T.);
#4276=FACE_OUTER_BOUND('',#5958,.T.);
#4277=FACE_OUTER_BOUND('',#5959,.T.);
#4278=FACE_OUTER_BOUND('',#5960,.T.);
#4279=FACE_OUTER_BOUND('',#5961,.T.);
#4280=FACE_OUTER_BOUND('',#5962,.T.);
#4281=FACE_OUTER_BOUND('',#5963,.T.);
#4282=FACE_OUTER_BOUND('',#5964,.T.);
#4283=FACE_OUTER_BOUND('',#5965,.T.);
#4284=FACE_OUTER_BOUND('',#5966,.T.);
#4285=FACE_OUTER_BOUND('',#5967,.T.);
#4286=FACE_OUTER_BOUND('',#5968,.T.);
#4287=FACE_OUTER_BOUND('',#5969,.T.);
#4288=FACE_OUTER_BOUND('',#5970,.T.);
#4289=FACE_OUTER_BOUND('',#5971,.T.);
#4290=FACE_OUTER_BOUND('',#5972,.T.);
#4291=FACE_OUTER_BOUND('',#5973,.T.);
#4292=FACE_OUTER_BOUND('',#5974,.T.);
#4293=FACE_OUTER_BOUND('',#5975,.T.);
#4294=FACE_OUTER_BOUND('',#5976,.T.);
#4295=FACE_OUTER_BOUND('',#5977,.T.);
#4296=FACE_OUTER_BOUND('',#5978,.T.);
#4297=FACE_OUTER_BOUND('',#5979,.T.);
#4298=FACE_OUTER_BOUND('',#5980,.T.);
#4299=FACE_OUTER_BOUND('',#5981,.T.);
#4300=FACE_OUTER_BOUND('',#5982,.T.);
#4301=FACE_OUTER_BOUND('',#5983,.T.);
#4302=FACE_OUTER_BOUND('',#5984,.T.);
#4303=FACE_OUTER_BOUND('',#5985,.T.);
#4304=FACE_OUTER_BOUND('',#5986,.T.);
#4305=FACE_OUTER_BOUND('',#5987,.T.);
#4306=FACE_OUTER_BOUND('',#5988,.T.);
#4307=FACE_OUTER_BOUND('',#5989,.T.);
#4308=FACE_OUTER_BOUND('',#5990,.T.);
#4309=FACE_OUTER_BOUND('',#5991,.T.);
#4310=FACE_OUTER_BOUND('',#5992,.T.);
#4311=FACE_OUTER_BOUND('',#5993,.T.);
#4312=FACE_OUTER_BOUND('',#5994,.T.);
#4313=FACE_OUTER_BOUND('',#5995,.T.);
#4314=FACE_OUTER_BOUND('',#5996,.T.);
#4315=FACE_OUTER_BOUND('',#5997,.T.);
#4316=FACE_OUTER_BOUND('',#6000,.T.);
#4317=FACE_OUTER_BOUND('',#6001,.T.);
#4318=FACE_OUTER_BOUND('',#6002,.T.);
#4319=FACE_OUTER_BOUND('',#6003,.T.);
#4320=FACE_OUTER_BOUND('',#6004,.T.);
#4321=FACE_OUTER_BOUND('',#6005,.T.);
#4322=FACE_OUTER_BOUND('',#6006,.T.);
#4323=FACE_OUTER_BOUND('',#6007,.T.);
#4324=FACE_OUTER_BOUND('',#6008,.T.);
#4325=FACE_OUTER_BOUND('',#6009,.T.);
#4326=FACE_OUTER_BOUND('',#6010,.T.);
#4327=FACE_OUTER_BOUND('',#6011,.T.);
#4328=FACE_OUTER_BOUND('',#6012,.T.);
#4329=FACE_OUTER_BOUND('',#6013,.T.);
#4330=FACE_OUTER_BOUND('',#6014,.T.);
#4331=FACE_OUTER_BOUND('',#6015,.T.);
#4332=FACE_OUTER_BOUND('',#6016,.T.);
#4333=FACE_OUTER_BOUND('',#6017,.T.);
#4334=FACE_OUTER_BOUND('',#6018,.T.);
#4335=FACE_OUTER_BOUND('',#6019,.T.);
#4336=FACE_OUTER_BOUND('',#6020,.T.);
#4337=FACE_OUTER_BOUND('',#6021,.T.);
#4338=FACE_OUTER_BOUND('',#6022,.T.);
#4339=FACE_OUTER_BOUND('',#6023,.T.);
#4340=FACE_OUTER_BOUND('',#6024,.T.);
#4341=FACE_OUTER_BOUND('',#6025,.T.);
#4342=FACE_OUTER_BOUND('',#6026,.T.);
#4343=FACE_OUTER_BOUND('',#6027,.T.);
#4344=FACE_OUTER_BOUND('',#6028,.T.);
#4345=FACE_OUTER_BOUND('',#6029,.T.);
#4346=FACE_OUTER_BOUND('',#6030,.T.);
#4347=FACE_OUTER_BOUND('',#6031,.T.);
#4348=FACE_OUTER_BOUND('',#6032,.T.);
#4349=FACE_OUTER_BOUND('',#6033,.T.);
#4350=FACE_OUTER_BOUND('',#6034,.T.);
#4351=FACE_OUTER_BOUND('',#6035,.T.);
#4352=FACE_OUTER_BOUND('',#6036,.T.);
#4353=FACE_OUTER_BOUND('',#6037,.T.);
#4354=FACE_OUTER_BOUND('',#6038,.T.);
#4355=FACE_OUTER_BOUND('',#6041,.T.);
#4356=FACE_OUTER_BOUND('',#6042,.T.);
#4357=FACE_OUTER_BOUND('',#6043,.T.);
#4358=FACE_OUTER_BOUND('',#6044,.T.);
#4359=FACE_OUTER_BOUND('',#6045,.T.);
#4360=FACE_OUTER_BOUND('',#6046,.T.);
#4361=FACE_OUTER_BOUND('',#6047,.T.);
#4362=FACE_OUTER_BOUND('',#6048,.T.);
#4363=FACE_OUTER_BOUND('',#6049,.T.);
#4364=FACE_OUTER_BOUND('',#6050,.T.);
#4365=FACE_OUTER_BOUND('',#6051,.T.);
#4366=FACE_OUTER_BOUND('',#6053,.T.);
#4367=FACE_OUTER_BOUND('',#6054,.T.);
#4368=FACE_OUTER_BOUND('',#6055,.T.);
#4369=FACE_OUTER_BOUND('',#6056,.T.);
#4370=FACE_OUTER_BOUND('',#6057,.T.);
#4371=FACE_OUTER_BOUND('',#6058,.T.);
#4372=FACE_OUTER_BOUND('',#6059,.T.);
#4373=FACE_OUTER_BOUND('',#6060,.T.);
#4374=FACE_OUTER_BOUND('',#6061,.T.);
#4375=FACE_OUTER_BOUND('',#6065,.T.);
#4376=FACE_OUTER_BOUND('',#6066,.T.);
#5845=EDGE_LOOP('',(#24089,#24090,#24091,#24092));
#5846=EDGE_LOOP('',(#24093,#24094,#24095,#24096));
#5847=EDGE_LOOP('',(#24097,#24098,#24099,#24100));
#5848=EDGE_LOOP('',(#24101,#24102,#24103,#24104));
#5849=EDGE_LOOP('',(#24105,#24106,#24107,#24108));
#5850=EDGE_LOOP('',(#24109,#24110,#24111,#24112));
#5851=EDGE_LOOP('',(#24113,#24114,#24115,#24116));
#5852=EDGE_LOOP('',(#24117,#24118,#24119,#24120));
#5853=EDGE_LOOP('',(#24121,#24122,#24123,#24124));
#5854=EDGE_LOOP('',(#24125,#24126,#24127,#24128));
#5855=EDGE_LOOP('',(#24129,#24130,#24131,#24132));
#5856=EDGE_LOOP('',(#24133,#24134,#24135,#24136));
#5857=EDGE_LOOP('',(#24137,#24138,#24139,#24140));
#5858=EDGE_LOOP('',(#24141,#24142,#24143,#24144));
#5859=EDGE_LOOP('',(#24145,#24146,#24147,#24148));
#5860=EDGE_LOOP('',(#24149,#24150,#24151,#24152));
#5861=EDGE_LOOP('',(#24153,#24154,#24155,#24156));
#5862=EDGE_LOOP('',(#24157,#24158,#24159,#24160));
#5863=EDGE_LOOP('',(#24161,#24162,#24163,#24164));
#5864=EDGE_LOOP('',(#24165,#24166,#24167,#24168));
#5865=EDGE_LOOP('',(#24169,#24170,#24171,#24172));
#5866=EDGE_LOOP('',(#24173,#24174,#24175,#24176));
#5867=EDGE_LOOP('',(#24177,#24178,#24179,#24180));
#5868=EDGE_LOOP('',(#24181,#24182,#24183,#24184));
#5869=EDGE_LOOP('',(#24185,#24186,#24187,#24188));
#5870=EDGE_LOOP('',(#24189,#24190,#24191,#24192));
#5871=EDGE_LOOP('',(#24193,#24194,#24195,#24196));
#5872=EDGE_LOOP('',(#24197,#24198,#24199,#24200));
#5873=EDGE_LOOP('',(#24201,#24202,#24203,#24204));
#5874=EDGE_LOOP('',(#24205,#24206,#24207,#24208));
#5875=EDGE_LOOP('',(#24209,#24210,#24211,#24212));
#5876=EDGE_LOOP('',(#24213,#24214,#24215,#24216));
#5877=EDGE_LOOP('',(#24217,#24218,#24219,#24220));
#5878=EDGE_LOOP('',(#24221,#24222,#24223,#24224));
#5879=EDGE_LOOP('',(#24225,#24226,#24227,#24228));
#5880=EDGE_LOOP('',(#24229,#24230,#24231,#24232));
#5881=EDGE_LOOP('',(#24233,#24234,#24235,#24236));
#5882=EDGE_LOOP('',(#24237,#24238,#24239,#24240));
#5883=EDGE_LOOP('',(#24241,#24242,#24243,#24244));
#5884=EDGE_LOOP('',(#24245,#24246,#24247,#24248));
#5885=EDGE_LOOP('',(#24249,#24250,#24251,#24252));
#5886=EDGE_LOOP('',(#24253,#24254,#24255,#24256));
#5887=EDGE_LOOP('',(#24257,#24258,#24259,#24260));
#5888=EDGE_LOOP('',(#24261,#24262,#24263,#24264));
#5889=EDGE_LOOP('',(#24265,#24266,#24267,#24268));
#5890=EDGE_LOOP('',(#24269,#24270,#24271,#24272));
#5891=EDGE_LOOP('',(#24273,#24274,#24275,#24276));
#5892=EDGE_LOOP('',(#24277,#24278,#24279,#24280));
#5893=EDGE_LOOP('',(#24281,#24282,#24283,#24284));
#5894=EDGE_LOOP('',(#24285,#24286,#24287,#24288));
#5895=EDGE_LOOP('',(#24289,#24290,#24291,#24292));
#5896=EDGE_LOOP('',(#24293,#24294,#24295,#24296));
#5897=EDGE_LOOP('',(#24297,#24298,#24299,#24300));
#5898=EDGE_LOOP('',(#24301,#24302,#24303,#24304));
#5899=EDGE_LOOP('',(#24305,#24306,#24307,#24308));
#5900=EDGE_LOOP('',(#24309,#24310,#24311,#24312));
#5901=EDGE_LOOP('',(#24313,#24314,#24315,#24316));
#5902=EDGE_LOOP('',(#24317,#24318,#24319,#24320));
#5903=EDGE_LOOP('',(#24321,#24322,#24323,#24324));
#5904=EDGE_LOOP('',(#24325,#24326,#24327,#24328,#24329));
#5905=EDGE_LOOP('',(#24330,#24331,#24332,#24333));
#5906=EDGE_LOOP('',(#24334,#24335,#24336,#24337));
#5907=EDGE_LOOP('',(#24338,#24339,#24340,#24341));
#5908=EDGE_LOOP('',(#24342,#24343,#24344,#24345));
#5909=EDGE_LOOP('',(#24346,#24347,#24348,#24349));
#5910=EDGE_LOOP('',(#24350,#24351,#24352,#24353));
#5911=EDGE_LOOP('',(#24354,#24355,#24356,#24357));
#5912=EDGE_LOOP('',(#24358,#24359,#24360,#24361));
#5913=EDGE_LOOP('',(#24362,#24363,#24364,#24365));
#5914=EDGE_LOOP('',(#24366,#24367,#24368,#24369));
#5915=EDGE_LOOP('',(#24370,#24371,#24372,#24373));
#5916=EDGE_LOOP('',(#24374,#24375,#24376,#24377));
#5917=EDGE_LOOP('',(#24378,#24379,#24380,#24381));
#5918=EDGE_LOOP('',(#24382,#24383,#24384,#24385));
#5919=EDGE_LOOP('',(#24386,#24387,#24388,#24389));
#5920=EDGE_LOOP('',(#24390,#24391,#24392,#24393));
#5921=EDGE_LOOP('',(#24394,#24395,#24396,#24397));
#5922=EDGE_LOOP('',(#24398,#24399,#24400,#24401));
#5923=EDGE_LOOP('',(#24402,#24403,#24404,#24405));
#5924=EDGE_LOOP('',(#24406,#24407,#24408,#24409));
#5925=EDGE_LOOP('',(#24410,#24411,#24412,#24413));
#5926=EDGE_LOOP('',(#24414,#24415,#24416,#24417));
#5927=EDGE_LOOP('',(#24418,#24419,#24420,#24421));
#5928=EDGE_LOOP('',(#24422,#24423,#24424,#24425));
#5929=EDGE_LOOP('',(#24426,#24427,#24428,#24429));
#5930=EDGE_LOOP('',(#24430,#24431,#24432,#24433));
#5931=EDGE_LOOP('',(#24434,#24435,#24436,#24437));
#5932=EDGE_LOOP('',(#24438,#24439,#24440,#24441));
#5933=EDGE_LOOP('',(#24442,#24443,#24444,#24445));
#5934=EDGE_LOOP('',(#24446,#24447,#24448,#24449));
#5935=EDGE_LOOP('',(#24450,#24451,#24452,#24453));
#5936=EDGE_LOOP('',(#24454,#24455,#24456,#24457));
#5937=EDGE_LOOP('',(#24458,#24459,#24460,#24461));
#5938=EDGE_LOOP('',(#24462,#24463,#24464,#24465));
#5939=EDGE_LOOP('',(#24466,#24467,#24468,#24469));
#5940=EDGE_LOOP('',(#24470,#24471,#24472,#24473));
#5941=EDGE_LOOP('',(#24474,#24475,#24476,#24477));
#5942=EDGE_LOOP('',(#24478,#24479,#24480,#24481));
#5943=EDGE_LOOP('',(#24482,#24483,#24484,#24485));
#5944=EDGE_LOOP('',(#24486,#24487,#24488,#24489));
#5945=EDGE_LOOP('',(#24490,#24491,#24492,#24493));
#5946=EDGE_LOOP('',(#24494,#24495,#24496,#24497));
#5947=EDGE_LOOP('',(#24498,#24499,#24500,#24501));
#5948=EDGE_LOOP('',(#24502,#24503,#24504,#24505));
#5949=EDGE_LOOP('',(#24506,#24507,#24508,#24509));
#5950=EDGE_LOOP('',(#24510,#24511,#24512,#24513));
#5951=EDGE_LOOP('',(#24514,#24515,#24516,#24517));
#5952=EDGE_LOOP('',(#24518,#24519,#24520,#24521));
#5953=EDGE_LOOP('',(#24522,#24523,#24524,#24525));
#5954=EDGE_LOOP('',(#24526,#24527,#24528,#24529));
#5955=EDGE_LOOP('',(#24530,#24531,#24532,#24533));
#5956=EDGE_LOOP('',(#24534,#24535,#24536,#24537));
#5957=EDGE_LOOP('',(#24538,#24539,#24540,#24541));
#5958=EDGE_LOOP('',(#24542,#24543,#24544,#24545));
#5959=EDGE_LOOP('',(#24546,#24547,#24548,#24549));
#5960=EDGE_LOOP('',(#24550,#24551,#24552,#24553));
#5961=EDGE_LOOP('',(#24554,#24555,#24556,#24557));
#5962=EDGE_LOOP('',(#24558,#24559,#24560,#24561));
#5963=EDGE_LOOP('',(#24562,#24563,#24564,#24565));
#5964=EDGE_LOOP('',(#24566,#24567,#24568,#24569));
#5965=EDGE_LOOP('',(#24570,#24571,#24572,#24573));
#5966=EDGE_LOOP('',(#24574,#24575,#24576,#24577));
#5967=EDGE_LOOP('',(#24578,#24579,#24580,#24581));
#5968=EDGE_LOOP('',(#24582,#24583,#24584,#24585));
#5969=EDGE_LOOP('',(#24586,#24587,#24588,#24589));
#5970=EDGE_LOOP('',(#24590,#24591,#24592,#24593));
#5971=EDGE_LOOP('',(#24594,#24595,#24596,#24597));
#5972=EDGE_LOOP('',(#24598,#24599,#24600,#24601));
#5973=EDGE_LOOP('',(#24602,#24603,#24604,#24605));
#5974=EDGE_LOOP('',(#24606,#24607,#24608,#24609));
#5975=EDGE_LOOP('',(#24610,#24611,#24612,#24613));
#5976=EDGE_LOOP('',(#24614,#24615,#24616,#24617));
#5977=EDGE_LOOP('',(#24618,#24619,#24620,#24621));
#5978=EDGE_LOOP('',(#24622,#24623,#24624,#24625));
#5979=EDGE_LOOP('',(#24626,#24627,#24628,#24629));
#5980=EDGE_LOOP('',(#24630,#24631,#24632,#24633));
#5981=EDGE_LOOP('',(#24634,#24635,#24636,#24637));
#5982=EDGE_LOOP('',(#24638,#24639,#24640,#24641));
#5983=EDGE_LOOP('',(#24642,#24643,#24644,#24645));
#5984=EDGE_LOOP('',(#24646,#24647,#24648,#24649));
#5985=EDGE_LOOP('',(#24650,#24651,#24652,#24653));
#5986=EDGE_LOOP('',(#24654,#24655,#24656,#24657));
#5987=EDGE_LOOP('',(#24658,#24659,#24660,#24661));
#5988=EDGE_LOOP('',(#24662,#24663,#24664,#24665));
#5989=EDGE_LOOP('',(#24666,#24667,#24668,#24669));
#5990=EDGE_LOOP('',(#24670,#24671,#24672,#24673));
#5991=EDGE_LOOP('',(#24674,#24675,#24676,#24677));
#5992=EDGE_LOOP('',(#24678,#24679,#24680,#24681));
#5993=EDGE_LOOP('',(#24682,#24683,#24684,#24685));
#5994=EDGE_LOOP('',(#24686,#24687,#24688,#24689));
#5995=EDGE_LOOP('',(#24690,#24691,#24692,#24693));
#5996=EDGE_LOOP('',(#24694,#24695,#24696,#24697));
#5997=EDGE_LOOP('',(#24698,#24699,#24700,#24701,#24702,#24703,#24704,#24705,
#24706,#24707,#24708,#24709,#24710,#24711,#24712,#24713));
#5998=EDGE_LOOP('',(#24714,#24715,#24716,#24717,#24718,#24719,#24720,#24721));
#5999=EDGE_LOOP('',(#24722,#24723,#24724,#24725,#24726,#24727,#24728,#24729,
#24730));
#6000=EDGE_LOOP('',(#24731,#24732,#24733,#24734));
#6001=EDGE_LOOP('',(#24735,#24736,#24737,#24738));
#6002=EDGE_LOOP('',(#24739,#24740,#24741,#24742));
#6003=EDGE_LOOP('',(#24743,#24744,#24745,#24746));
#6004=EDGE_LOOP('',(#24747,#24748,#24749,#24750));
#6005=EDGE_LOOP('',(#24751,#24752,#24753,#24754));
#6006=EDGE_LOOP('',(#24755,#24756,#24757,#24758));
#6007=EDGE_LOOP('',(#24759,#24760,#24761,#24762));
#6008=EDGE_LOOP('',(#24763,#24764,#24765,#24766));
#6009=EDGE_LOOP('',(#24767,#24768,#24769,#24770));
#6010=EDGE_LOOP('',(#24771,#24772,#24773,#24774));
#6011=EDGE_LOOP('',(#24775,#24776,#24777,#24778));
#6012=EDGE_LOOP('',(#24779,#24780,#24781,#24782));
#6013=EDGE_LOOP('',(#24783,#24784,#24785,#24786));
#6014=EDGE_LOOP('',(#24787,#24788,#24789,#24790));
#6015=EDGE_LOOP('',(#24791,#24792,#24793,#24794));
#6016=EDGE_LOOP('',(#24795,#24796,#24797,#24798));
#6017=EDGE_LOOP('',(#24799,#24800,#24801,#24802));
#6018=EDGE_LOOP('',(#24803,#24804,#24805,#24806));
#6019=EDGE_LOOP('',(#24807,#24808,#24809,#24810));
#6020=EDGE_LOOP('',(#24811,#24812,#24813,#24814));
#6021=EDGE_LOOP('',(#24815,#24816,#24817,#24818));
#6022=EDGE_LOOP('',(#24819,#24820,#24821,#24822));
#6023=EDGE_LOOP('',(#24823,#24824,#24825,#24826));
#6024=EDGE_LOOP('',(#24827,#24828,#24829,#24830));
#6025=EDGE_LOOP('',(#24831,#24832,#24833,#24834));
#6026=EDGE_LOOP('',(#24835,#24836,#24837,#24838));
#6027=EDGE_LOOP('',(#24839,#24840,#24841,#24842));
#6028=EDGE_LOOP('',(#24843,#24844,#24845,#24846));
#6029=EDGE_LOOP('',(#24847,#24848,#24849,#24850));
#6030=EDGE_LOOP('',(#24851,#24852,#24853,#24854));
#6031=EDGE_LOOP('',(#24855,#24856,#24857,#24858));
#6032=EDGE_LOOP('',(#24859,#24860,#24861,#24862));
#6033=EDGE_LOOP('',(#24863,#24864,#24865,#24866));
#6034=EDGE_LOOP('',(#24867,#24868,#24869,#24870));
#6035=EDGE_LOOP('',(#24871,#24872,#24873,#24874));
#6036=EDGE_LOOP('',(#24875,#24876,#24877,#24878));
#6037=EDGE_LOOP('',(#24879,#24880,#24881,#24882));
#6038=EDGE_LOOP('',(#24883,#24884,#24885,#24886,#24887,#24888,#24889,#24890,
#24891,#24892,#24893,#24894,#24895,#24896,#24897,#24898));
#6039=EDGE_LOOP('',(#24899,#24900,#24901,#24902,#24903,#24904,#24905,#24906));
#6040=EDGE_LOOP('',(#24907,#24908,#24909,#24910,#24911,#24912,#24913,#24914,
#24915));
#6041=EDGE_LOOP('',(#24916,#24917,#24918,#24919,#24920,#24921,#24922,#24923));
#6042=EDGE_LOOP('',(#24924,#24925,#24926,#24927,#24928,#24929,#24930,#24931,
#24932));
#6043=EDGE_LOOP('',(#24933,#24934,#24935,#24936,#24937,#24938,#24939,#24940));
#6044=EDGE_LOOP('',(#24941,#24942,#24943,#24944,#24945,#24946,#24947,#24948,
#24949));
#6045=EDGE_LOOP('',(#24950,#24951,#24952,#24953,#24954));
#6046=EDGE_LOOP('',(#24955,#24956,#24957,#24958,#24959,#24960,#24961,#24962,
#24963,#24964,#24965,#24966,#24967,#24968,#24969,#24970,#24971,#24972,#24973,
#24974,#24975,#24976,#24977,#24978,#24979,#24980,#24981,#24982,#24983,#24984,
#24985,#24986,#24987,#24988,#24989,#24990,#24991,#24992,#24993,#24994,#24995,
#24996,#24997,#24998,#24999,#25000,#25001,#25002,#25003,#25004,#25005,#25006,
#25007,#25008,#25009,#25010,#25011,#25012,#25013,#25014,#25015,#25016,#25017,
#25018,#25019,#25020,#25021,#25022,#25023,#25024,#25025,#25026,#25027,#25028,
#25029,#25030,#25031,#25032,#25033,#25034,#25035,#25036,#25037,#25038,#25039,
#25040,#25041,#25042,#25043,#25044,#25045,#25046,#25047,#25048,#25049,#25050,
#25051,#25052,#25053,#25054,#25055,#25056,#25057,#25058,#25059,#25060,#25061,
#25062,#25063,#25064,#25065,#25066,#25067,#25068,#25069,#25070,#25071,#25072,
#25073,#25074,#25075,#25076,#25077));
#6047=EDGE_LOOP('',(#25078,#25079,#25080,#25081,#25082));
#6048=EDGE_LOOP('',(#25083,#25084,#25085,#25086));
#6049=EDGE_LOOP('',(#25087,#25088,#25089,#25090,#25091,#25092,#25093,#25094,
#25095,#25096,#25097,#25098,#25099,#25100,#25101,#25102,#25103,#25104,#25105,
#25106,#25107,#25108,#25109,#25110,#25111,#25112,#25113,#25114,#25115,#25116,
#25117,#25118,#25119,#25120,#25121,#25122,#25123,#25124,#25125,#25126,#25127,
#25128,#25129,#25130,#25131,#25132,#25133,#25134,#25135,#25136,#25137,#25138,
#25139,#25140,#25141,#25142,#25143,#25144,#25145,#25146,#25147,#25148,#25149,
#25150,#25151,#25152,#25153,#25154,#25155,#25156,#25157,#25158,#25159,#25160,
#25161,#25162,#25163,#25164,#25165,#25166,#25167,#25168,#25169,#25170,#25171,
#25172,#25173,#25174,#25175,#25176,#25177,#25178,#25179,#25180,#25181,#25182,
#25183,#25184,#25185,#25186,#25187,#25188,#25189,#25190,#25191,#25192,#25193,
#25194,#25195,#25196,#25197,#25198,#25199,#25200,#25201,#25202,#25203,#25204,
#25205,#25206,#25207,#25208));
#6050=EDGE_LOOP('',(#25209,#25210,#25211,#25212,#25213,#25214,#25215));
#6051=EDGE_LOOP('',(#25216,#25217,#25218,#25219,#25220,#25221));
#6052=EDGE_LOOP('',(#25222));
#6053=EDGE_LOOP('',(#25223,#25224,#25225));
#6054=EDGE_LOOP('',(#25226,#25227,#25228,#25229,#25230,#25231,#25232,#25233,
#25234,#25235));
#6055=EDGE_LOOP('',(#25236,#25237,#25238,#25239));
#6056=EDGE_LOOP('',(#25240,#25241,#25242,#25243));
#6057=EDGE_LOOP('',(#25244,#25245,#25246,#25247));
#6058=EDGE_LOOP('',(#25248,#25249,#25250,#25251));
#6059=EDGE_LOOP('',(#25252,#25253,#25254,#25255));
#6060=EDGE_LOOP('',(#25256,#25257,#25258,#25259,#25260));
#6061=EDGE_LOOP('',(#25261));
#6062=EDGE_LOOP('',(#25262,#25263,#25264,#25265,#25266,#25267,#25268,#25269,
#25270,#25271,#25272,#25273,#25274,#25275,#25276,#25277));
#6063=EDGE_LOOP('',(#25278,#25279,#25280,#25281));
#6064=EDGE_LOOP('',(#25282,#25283,#25284,#25285,#25286,#25287,#25288,#25289,
#25290,#25291,#25292,#25293,#25294,#25295,#25296,#25297));
#6065=EDGE_LOOP('',(#25298));
#6066=EDGE_LOOP('',(#25299,#25300,#25301,#25302,#25303,#25304));
#8378=LINE('',#59081,#10866);
#8379=LINE('',#59108,#10867);
#8380=LINE('',#59174,#10868);
#8381=LINE('',#59234,#10869);
#8382=LINE('',#59294,#10870);
#8383=LINE('',#59357,#10871);
#8384=LINE('',#59417,#10872);
#8385=LINE('',#59477,#10873);
#8386=LINE('',#59540,#10874);
#8387=LINE('',#59600,#10875);
#8388=LINE('',#59666,#10876);
#8389=LINE('',#59735,#10877);
#8390=LINE('',#59801,#10878);
#8391=LINE('',#59861,#10879);
#8392=LINE('',#59924,#10880);
#8393=LINE('',#59990,#10881);
#8394=LINE('',#60050,#10882);
#8395=LINE('',#60104,#10883);
#8396=LINE('',#60158,#10884);
#8397=LINE('',#60218,#10885);
#8398=LINE('',#60284,#10886);
#8399=LINE('',#60350,#10887);
#8400=LINE('',#60419,#10888);
#8401=LINE('',#60479,#10889);
#8402=LINE('',#60542,#10890);
#8403=LINE('',#60608,#10891);
#8404=LINE('',#60674,#10892);
#8405=LINE('',#60728,#10893);
#8406=LINE('',#60782,#10894);
#8407=LINE('',#60845,#10895);
#8408=LINE('',#60911,#10896);
#8409=LINE('',#60962,#10897);
#8410=LINE('',#61025,#10898);
#8411=LINE('',#61079,#10899);
#8412=LINE('',#61142,#10900);
#8413=LINE('',#61211,#10901);
#8414=LINE('',#61274,#10902);
#8415=LINE('',#61328,#10903);
#8416=LINE('',#61388,#10904);
#8417=LINE('',#61448,#10905);
#8418=LINE('',#61508,#10906);
#8419=LINE('',#61571,#10907);
#8420=LINE('',#61625,#10908);
#8421=LINE('',#61679,#10909);
#8422=LINE('',#61745,#10910);
#8423=LINE('',#61814,#10911);
#8424=LINE('',#61877,#10912);
#8425=LINE('',#61931,#10913);
#8426=LINE('',#61997,#10914);
#8427=LINE('',#62063,#10915);
#8428=LINE('',#62123,#10916);
#8429=LINE('',#62183,#10917);
#8430=LINE('',#62237,#10918);
#8431=LINE('',#62294,#10919);
#8432=LINE('',#62360,#10920);
#8433=LINE('',#62429,#10921);
#8434=LINE('',#62492,#10922);
#8435=LINE('',#62546,#10923);
#8436=LINE('',#62612,#10924);
#8437=LINE('',#62678,#10925);
#8438=LINE('',#62737,#10926);
#8439=LINE('',#62768,#10927);
#8440=LINE('',#62798,#10928);
#8441=LINE('',#62828,#10929);
#8442=LINE('',#62873,#10930);
#8443=LINE('',#62918,#10931);
#8444=LINE('',#62948,#10932);
#8445=LINE('',#62978,#10933);
#8446=LINE('',#63007,#10934);
#8447=LINE('',#63049,#10935);
#8448=LINE('',#63079,#10936);
#8449=LINE('',#63121,#10937);
#8450=LINE('',#63151,#10938);
#8451=LINE('',#63181,#10939);
#8452=LINE('',#63223,#10940);
#8453=LINE('',#63265,#10941);
#8454=LINE('',#63295,#10942);
#8455=LINE('',#63325,#10943);
#8456=LINE('',#63367,#10944);
#8457=LINE('',#63421,#10945);
#8458=LINE('',#63451,#10946);
#8459=LINE('',#63493,#10947);
#8460=LINE('',#63522,#10948);
#8461=LINE('',#63552,#10949);
#8462=LINE('',#63595,#10950);
#8463=LINE('',#63637,#10951);
#8464=LINE('',#63667,#10952);
#8465=LINE('',#63696,#10953);
#8466=LINE('',#63738,#10954);
#8467=LINE('',#63795,#10955);
#8468=LINE('',#63824,#10956);
#8469=LINE('',#63851,#10957);
#8470=LINE('',#63880,#10958);
#8471=LINE('',#63925,#10959);
#8472=LINE('',#63968,#10960);
#8473=LINE('',#64013,#10961);
#8474=LINE('',#64043,#10962);
#8475=LINE('',#64073,#10963);
#8476=LINE('',#64102,#10964);
#8477=LINE('',#64148,#10965);
#8478=LINE('',#64178,#10966);
#8479=LINE('',#64208,#10967);
#8480=LINE('',#64237,#10968);
#8481=LINE('',#64279,#10969);
#8482=LINE('',#64322,#10970);
#8483=LINE('',#64364,#10971);
#8484=LINE('',#64394,#10972);
#8485=LINE('',#64424,#10973);
#8486=LINE('',#64453,#10974);
#8487=LINE('',#64495,#10975);
#8488=LINE('',#64526,#10976);
#8489=LINE('',#64556,#10977);
#8490=LINE('',#64598,#10978);
#8491=LINE('',#64640,#10979);
#8492=LINE('',#64671,#10980);
#8493=LINE('',#64713,#10981);
#8494=LINE('',#64743,#10982);
#8495=LINE('',#64772,#10983);
#8496=LINE('',#64802,#10984);
#8497=LINE('',#64853,#10985);
#8498=LINE('',#64858,#10986);
#8499=LINE('',#64870,#10987);
#8500=LINE('',#64885,#10988);
#8501=LINE('',#64900,#10989);
#8502=LINE('',#64915,#10990);
#8503=LINE('',#64930,#10991);
#8504=LINE('',#64945,#10992);
#8505=LINE('',#64960,#10993);
#8506=LINE('',#64988,#10994);
#8507=LINE('',#64993,#10995);
#8508=LINE('',#65005,#10996);
#8509=LINE('',#65020,#10997);
#8510=LINE('',#65035,#10998);
#8511=LINE('',#65050,#10999);
#8512=LINE('',#65065,#11000);
#8513=LINE('',#65080,#11001);
#8514=LINE('',#65108,#11002);
#8515=LINE('',#65113,#11003);
#8516=LINE('',#65125,#11004);
#8517=LINE('',#65140,#11005);
#8518=LINE('',#65155,#11006);
#8519=LINE('',#65170,#11007);
#8520=LINE('',#65185,#11008);
#8521=LINE('',#65200,#11009);
#8522=LINE('',#65215,#11010);
#8523=LINE('',#65230,#11011);
#8524=LINE('',#65245,#11012);
#8525=LINE('',#65260,#11013);
#8526=LINE('',#65275,#11014);
#8527=LINE('',#65290,#11015);
#8528=LINE('',#65305,#11016);
#8529=LINE('',#65320,#11017);
#8530=LINE('',#65340,#11018);
#8531=LINE('',#65342,#11019);
#8532=LINE('',#65344,#11020);
#8533=LINE('',#65345,#11021);
#8534=LINE('',#65348,#11022);
#8535=LINE('',#65350,#11023);
#8536=LINE('',#65351,#11024);
#8537=LINE('',#65354,#11025);
#8538=LINE('',#65356,#11026);
#8539=LINE('',#65357,#11027);
#8540=LINE('',#65359,#11028);
#8541=LINE('',#65360,#11029);
#8542=LINE('',#65374,#11030);
#8543=LINE('',#65379,#11031);
#8544=LINE('',#65391,#11032);
#8545=LINE('',#65406,#11033);
#8546=LINE('',#65421,#11034);
#8547=LINE('',#65436,#11035);
#8548=LINE('',#65451,#11036);
#8549=LINE('',#65466,#11037);
#8550=LINE('',#65481,#11038);
#8551=LINE('',#65509,#11039);
#8552=LINE('',#65514,#11040);
#8553=LINE('',#65526,#11041);
#8554=LINE('',#65541,#11042);
#8555=LINE('',#65556,#11043);
#8556=LINE('',#65571,#11044);
#8557=LINE('',#65586,#11045);
#8558=LINE('',#65601,#11046);
#8559=LINE('',#65629,#11047);
#8560=LINE('',#65634,#11048);
#8561=LINE('',#65646,#11049);
#8562=LINE('',#65661,#11050);
#8563=LINE('',#65676,#11051);
#8564=LINE('',#65691,#11052);
#8565=LINE('',#65706,#11053);
#8566=LINE('',#65721,#11054);
#8567=LINE('',#65736,#11055);
#8568=LINE('',#65751,#11056);
#8569=LINE('',#65766,#11057);
#8570=LINE('',#65781,#11058);
#8571=LINE('',#65796,#11059);
#8572=LINE('',#65811,#11060);
#8573=LINE('',#65826,#11061);
#8574=LINE('',#65841,#11062);
#8575=LINE('',#70510,#11063);
#8576=LINE('',#70512,#11064);
#8577=LINE('',#70514,#11065);
#8578=LINE('',#70516,#11066);
#8579=LINE('',#70518,#11067);
#8580=LINE('',#70519,#11068);
#8581=LINE('',#70544,#11069);
#8582=LINE('',#70554,#11070);
#8583=LINE('',#70555,#11071);
#8584=LINE('',#70557,#11072);
#8585=LINE('',#70559,#11073);
#8586=LINE('',#70561,#11074);
#8587=LINE('',#70563,#11075);
#8588=LINE('',#70570,#11076);
#10866=VECTOR('',#36127,0.8);
#10867=VECTOR('',#36132,0.8);
#10868=VECTOR('',#36135,0.8);
#10869=VECTOR('',#36138,0.8);
#10870=VECTOR('',#36141,0.8);
#10871=VECTOR('',#36144,0.8);
#10872=VECTOR('',#36147,0.8);
#10873=VECTOR('',#36150,0.8);
#10874=VECTOR('',#36153,0.8);
#10875=VECTOR('',#36156,0.8);
#10876=VECTOR('',#36159,0.8);
#10877=VECTOR('',#36162,0.8);
#10878=VECTOR('',#36165,0.8);
#10879=VECTOR('',#36168,0.8);
#10880=VECTOR('',#36171,0.8);
#10881=VECTOR('',#36174,0.8);
#10882=VECTOR('',#36177,0.8);
#10883=VECTOR('',#36180,0.8);
#10884=VECTOR('',#36183,0.8);
#10885=VECTOR('',#36186,0.8);
#10886=VECTOR('',#36189,0.8);
#10887=VECTOR('',#36192,0.8);
#10888=VECTOR('',#36195,0.8);
#10889=VECTOR('',#36198,0.8);
#10890=VECTOR('',#36201,0.8);
#10891=VECTOR('',#36204,0.8);
#10892=VECTOR('',#36207,0.8);
#10893=VECTOR('',#36210,0.8);
#10894=VECTOR('',#36213,0.8);
#10895=VECTOR('',#36216,0.8);
#10896=VECTOR('',#36219,0.8);
#10897=VECTOR('',#36222,0.8);
#10898=VECTOR('',#36225,0.8);
#10899=VECTOR('',#36228,0.8);
#10900=VECTOR('',#36231,0.8);
#10901=VECTOR('',#36234,0.8);
#10902=VECTOR('',#36237,0.8);
#10903=VECTOR('',#36240,0.8);
#10904=VECTOR('',#36243,0.8);
#10905=VECTOR('',#36246,0.8);
#10906=VECTOR('',#36249,0.8);
#10907=VECTOR('',#36252,0.8);
#10908=VECTOR('',#36255,0.8);
#10909=VECTOR('',#36258,0.8);
#10910=VECTOR('',#36261,0.8);
#10911=VECTOR('',#36264,0.8);
#10912=VECTOR('',#36267,0.8);
#10913=VECTOR('',#36270,0.8);
#10914=VECTOR('',#36273,0.8);
#10915=VECTOR('',#36276,0.8);
#10916=VECTOR('',#36279,0.8);
#10917=VECTOR('',#36282,0.8);
#10918=VECTOR('',#36285,0.8);
#10919=VECTOR('',#36288,0.8);
#10920=VECTOR('',#36291,0.8);
#10921=VECTOR('',#36294,0.8);
#10922=VECTOR('',#36297,0.8);
#10923=VECTOR('',#36300,0.8);
#10924=VECTOR('',#36303,0.8);
#10925=VECTOR('',#36306,0.8);
#10926=VECTOR('',#36311,0.6767);
#10927=VECTOR('',#36316,0.6767);
#10928=VECTOR('',#36319,0.6767);
#10929=VECTOR('',#36322,0.6767);
#10930=VECTOR('',#36325,0.6767);
#10931=VECTOR('',#36328,0.6767);
#10932=VECTOR('',#36331,0.6767);
#10933=VECTOR('',#36334,0.6767);
#10934=VECTOR('',#36337,0.6767);
#10935=VECTOR('',#36340,0.6767);
#10936=VECTOR('',#36343,0.6767);
#10937=VECTOR('',#36346,0.6767);
#10938=VECTOR('',#36349,0.6767);
#10939=VECTOR('',#36352,0.6767);
#10940=VECTOR('',#36355,0.6767);
#10941=VECTOR('',#36358,0.6767);
#10942=VECTOR('',#36361,0.6767);
#10943=VECTOR('',#36364,0.6767);
#10944=VECTOR('',#36367,0.6767);
#10945=VECTOR('',#36370,0.6767);
#10946=VECTOR('',#36373,0.6767);
#10947=VECTOR('',#36376,0.6767);
#10948=VECTOR('',#36379,0.6767);
#10949=VECTOR('',#36382,0.6767);
#10950=VECTOR('',#36385,0.6767);
#10951=VECTOR('',#36388,0.6767);
#10952=VECTOR('',#36391,0.6767);
#10953=VECTOR('',#36394,0.6767);
#10954=VECTOR('',#36397,0.6767);
#10955=VECTOR('',#36400,0.6767);
#10956=VECTOR('',#36403,0.6767);
#10957=VECTOR('',#36406,0.6767);
#10958=VECTOR('',#36409,0.6767);
#10959=VECTOR('',#36412,0.6767);
#10960=VECTOR('',#36415,0.6767);
#10961=VECTOR('',#36418,0.6767);
#10962=VECTOR('',#36421,0.6767);
#10963=VECTOR('',#36424,0.6767);
#10964=VECTOR('',#36427,0.6767);
#10965=VECTOR('',#36430,0.6767);
#10966=VECTOR('',#36433,0.6767);
#10967=VECTOR('',#36436,0.6767);
#10968=VECTOR('',#36439,0.6767);
#10969=VECTOR('',#36442,0.6767);
#10970=VECTOR('',#36445,0.6767);
#10971=VECTOR('',#36448,0.6767);
#10972=VECTOR('',#36451,0.6767);
#10973=VECTOR('',#36454,0.6767);
#10974=VECTOR('',#36457,0.6767);
#10975=VECTOR('',#36460,0.6767);
#10976=VECTOR('',#36463,0.6767);
#10977=VECTOR('',#36466,0.6767);
#10978=VECTOR('',#36469,0.6767);
#10979=VECTOR('',#36472,0.6767);
#10980=VECTOR('',#36475,0.6767);
#10981=VECTOR('',#36478,0.6767);
#10982=VECTOR('',#36481,0.6767);
#10983=VECTOR('',#36484,0.6767);
#10984=VECTOR('',#36487,0.6767);
#10985=VECTOR('',#36488,1.);
#10986=VECTOR('',#36489,1.);
#10987=VECTOR('',#36490,1.);
#10988=VECTOR('',#36491,1.);
#10989=VECTOR('',#36492,1.);
#10990=VECTOR('',#36493,1.);
#10991=VECTOR('',#36494,1.);
#10992=VECTOR('',#36495,1.);
#10993=VECTOR('',#36496,1.);
#10994=VECTOR('',#36497,1.);
#10995=VECTOR('',#36498,1.);
#10996=VECTOR('',#36499,1.);
#10997=VECTOR('',#36500,1.);
#10998=VECTOR('',#36501,1.);
#10999=VECTOR('',#36502,1.);
#11000=VECTOR('',#36503,1.);
#11001=VECTOR('',#36504,1.);
#11002=VECTOR('',#36505,1.);
#11003=VECTOR('',#36506,1.);
#11004=VECTOR('',#36507,1.);
#11005=VECTOR('',#36508,1.);
#11006=VECTOR('',#36509,1.);
#11007=VECTOR('',#36510,1.);
#11008=VECTOR('',#36511,1.);
#11009=VECTOR('',#36512,1.);
#11010=VECTOR('',#36513,1.);
#11011=VECTOR('',#36514,1.);
#11012=VECTOR('',#36515,1.);
#11013=VECTOR('',#36516,1.);
#11014=VECTOR('',#36517,1.);
#11015=VECTOR('',#36518,1.);
#11016=VECTOR('',#36519,1.);
#11017=VECTOR('',#36520,1.);
#11018=VECTOR('',#36525,1.);
#11019=VECTOR('',#36526,1.);
#11020=VECTOR('',#36527,1.);
#11021=VECTOR('',#36528,1.);
#11022=VECTOR('',#36531,1.);
#11023=VECTOR('',#36532,1.);
#11024=VECTOR('',#36533,1.);
#11025=VECTOR('',#36536,1.);
#11026=VECTOR('',#36537,1.);
#11027=VECTOR('',#36538,1.);
#11028=VECTOR('',#36541,1.);
#11029=VECTOR('',#36542,1.);
#11030=VECTOR('',#36545,1.);
#11031=VECTOR('',#36546,1.);
#11032=VECTOR('',#36547,1.);
#11033=VECTOR('',#36548,1.);
#11034=VECTOR('',#36549,1.);
#11035=VECTOR('',#36550,1.);
#11036=VECTOR('',#36551,1.);
#11037=VECTOR('',#36552,1.);
#11038=VECTOR('',#36553,1.);
#11039=VECTOR('',#36554,1.);
#11040=VECTOR('',#36555,1.);
#11041=VECTOR('',#36556,1.);
#11042=VECTOR('',#36557,1.);
#11043=VECTOR('',#36558,1.);
#11044=VECTOR('',#36559,1.);
#11045=VECTOR('',#36560,1.);
#11046=VECTOR('',#36561,1.);
#11047=VECTOR('',#36562,1.);
#11048=VECTOR('',#36563,1.);
#11049=VECTOR('',#36564,1.);
#11050=VECTOR('',#36565,1.);
#11051=VECTOR('',#36566,1.);
#11052=VECTOR('',#36567,1.);
#11053=VECTOR('',#36568,1.);
#11054=VECTOR('',#36569,1.);
#11055=VECTOR('',#36570,1.);
#11056=VECTOR('',#36571,1.);
#11057=VECTOR('',#36572,1.);
#11058=VECTOR('',#36573,1.);
#11059=VECTOR('',#36574,1.);
#11060=VECTOR('',#36575,1.);
#11061=VECTOR('',#36576,1.);
#11062=VECTOR('',#36577,1.);
#11063=VECTOR('',#36614,1.);
#11064=VECTOR('',#36615,1.);
#11065=VECTOR('',#36616,1.);
#11066=VECTOR('',#36617,1.);
#11067=VECTOR('',#36618,1.);
#11068=VECTOR('',#36619,1.);
#11069=VECTOR('',#36624,1.28782032302755);
#11070=VECTOR('',#36629,1.);
#11071=VECTOR('',#36630,1.);
#11072=VECTOR('',#36633,1.);
#11073=VECTOR('',#36636,1.);
#11074=VECTOR('',#36639,1.);
#11075=VECTOR('',#36642,1.);
#11076=VECTOR('',#36653,0.75);
#13213=VERTEX_POINT('',#59079);
#13214=VERTEX_POINT('',#59080);
#13215=VERTEX_POINT('',#59082);
#13216=VERTEX_POINT('',#59093);
#13217=VERTEX_POINT('',#59106);
#13218=VERTEX_POINT('',#59107);
#13219=VERTEX_POINT('',#59172);
#13220=VERTEX_POINT('',#59173);
#13221=VERTEX_POINT('',#59232);
#13222=VERTEX_POINT('',#59233);
#13223=VERTEX_POINT('',#59292);
#13224=VERTEX_POINT('',#59293);
#13225=VERTEX_POINT('',#59355);
#13226=VERTEX_POINT('',#59356);
#13227=VERTEX_POINT('',#59415);
#13228=VERTEX_POINT('',#59416);
#13229=VERTEX_POINT('',#59475);
#13230=VERTEX_POINT('',#59476);
#13231=VERTEX_POINT('',#59538);
#13232=VERTEX_POINT('',#59539);
#13233=VERTEX_POINT('',#59598);
#13234=VERTEX_POINT('',#59599);
#13235=VERTEX_POINT('',#59664);
#13236=VERTEX_POINT('',#59665);
#13237=VERTEX_POINT('',#59733);
#13238=VERTEX_POINT('',#59734);
#13239=VERTEX_POINT('',#59799);
#13240=VERTEX_POINT('',#59800);
#13241=VERTEX_POINT('',#59859);
#13242=VERTEX_POINT('',#59860);
#13243=VERTEX_POINT('',#59922);
#13244=VERTEX_POINT('',#59923);
#13245=VERTEX_POINT('',#59988);
#13246=VERTEX_POINT('',#59989);
#13247=VERTEX_POINT('',#60048);
#13248=VERTEX_POINT('',#60049);
#13249=VERTEX_POINT('',#60102);
#13250=VERTEX_POINT('',#60103);
#13251=VERTEX_POINT('',#60156);
#13252=VERTEX_POINT('',#60157);
#13253=VERTEX_POINT('',#60216);
#13254=VERTEX_POINT('',#60217);
#13255=VERTEX_POINT('',#60282);
#13256=VERTEX_POINT('',#60283);
#13257=VERTEX_POINT('',#60348);
#13258=VERTEX_POINT('',#60349);
#13259=VERTEX_POINT('',#60417);
#13260=VERTEX_POINT('',#60418);
#13261=VERTEX_POINT('',#60477);
#13262=VERTEX_POINT('',#60478);
#13263=VERTEX_POINT('',#60540);
#13264=VERTEX_POINT('',#60541);
#13265=VERTEX_POINT('',#60606);
#13266=VERTEX_POINT('',#60607);
#13267=VERTEX_POINT('',#60672);
#13268=VERTEX_POINT('',#60673);
#13269=VERTEX_POINT('',#60726);
#13270=VERTEX_POINT('',#60727);
#13271=VERTEX_POINT('',#60780);
#13272=VERTEX_POINT('',#60781);
#13273=VERTEX_POINT('',#60843);
#13274=VERTEX_POINT('',#60844);
#13275=VERTEX_POINT('',#60909);
#13276=VERTEX_POINT('',#60910);
#13277=VERTEX_POINT('',#60960);
#13278=VERTEX_POINT('',#60961);
#13279=VERTEX_POINT('',#61023);
#13280=VERTEX_POINT('',#61024);
#13281=VERTEX_POINT('',#61077);
#13282=VERTEX_POINT('',#61078);
#13283=VERTEX_POINT('',#61140);
#13284=VERTEX_POINT('',#61141);
#13285=VERTEX_POINT('',#61209);
#13286=VERTEX_POINT('',#61210);
#13287=VERTEX_POINT('',#61272);
#13288=VERTEX_POINT('',#61273);
#13289=VERTEX_POINT('',#61326);
#13290=VERTEX_POINT('',#61327);
#13291=VERTEX_POINT('',#61386);
#13292=VERTEX_POINT('',#61387);
#13293=VERTEX_POINT('',#61446);
#13294=VERTEX_POINT('',#61447);
#13295=VERTEX_POINT('',#61506);
#13296=VERTEX_POINT('',#61507);
#13297=VERTEX_POINT('',#61569);
#13298=VERTEX_POINT('',#61570);
#13299=VERTEX_POINT('',#61623);
#13300=VERTEX_POINT('',#61624);
#13301=VERTEX_POINT('',#61677);
#13302=VERTEX_POINT('',#61678);
#13303=VERTEX_POINT('',#61743);
#13304=VERTEX_POINT('',#61744);
#13305=VERTEX_POINT('',#61812);
#13306=VERTEX_POINT('',#61813);
#13307=VERTEX_POINT('',#61875);
#13308=VERTEX_POINT('',#61876);
#13309=VERTEX_POINT('',#61929);
#13310=VERTEX_POINT('',#61930);
#13311=VERTEX_POINT('',#61995);
#13312=VERTEX_POINT('',#61996);
#13313=VERTEX_POINT('',#62061);
#13314=VERTEX_POINT('',#62062);
#13315=VERTEX_POINT('',#62121);
#13316=VERTEX_POINT('',#62122);
#13317=VERTEX_POINT('',#62181);
#13318=VERTEX_POINT('',#62182);
#13319=VERTEX_POINT('',#62235);
#13320=VERTEX_POINT('',#62236);
#13321=VERTEX_POINT('',#62292);
#13322=VERTEX_POINT('',#62293);
#13323=VERTEX_POINT('',#62358);
#13324=VERTEX_POINT('',#62359);
#13325=VERTEX_POINT('',#62427);
#13326=VERTEX_POINT('',#62428);
#13327=VERTEX_POINT('',#62490);
#13328=VERTEX_POINT('',#62491);
#13329=VERTEX_POINT('',#62544);
#13330=VERTEX_POINT('',#62545);
#13331=VERTEX_POINT('',#62610);
#13332=VERTEX_POINT('',#62611);
#13333=VERTEX_POINT('',#62676);
#13334=VERTEX_POINT('',#62677);
#13335=VERTEX_POINT('',#62679);
#13336=VERTEX_POINT('',#62735);
#13337=VERTEX_POINT('',#62736);
#13338=VERTEX_POINT('',#62738);
#13339=VERTEX_POINT('',#62755);
#13340=VERTEX_POINT('',#62766);
#13341=VERTEX_POINT('',#62767);
#13342=VERTEX_POINT('',#62796);
#13343=VERTEX_POINT('',#62797);
#13344=VERTEX_POINT('',#62826);
#13345=VERTEX_POINT('',#62827);
#13346=VERTEX_POINT('',#62871);
#13347=VERTEX_POINT('',#62872);
#13348=VERTEX_POINT('',#62916);
#13349=VERTEX_POINT('',#62917);
#13350=VERTEX_POINT('',#62946);
#13351=VERTEX_POINT('',#62947);
#13352=VERTEX_POINT('',#62976);
#13353=VERTEX_POINT('',#62977);
#13354=VERTEX_POINT('',#63005);
#13355=VERTEX_POINT('',#63006);
#13356=VERTEX_POINT('',#63047);
#13357=VERTEX_POINT('',#63048);
#13358=VERTEX_POINT('',#63077);
#13359=VERTEX_POINT('',#63078);
#13360=VERTEX_POINT('',#63119);
#13361=VERTEX_POINT('',#63120);
#13362=VERTEX_POINT('',#63149);
#13363=VERTEX_POINT('',#63150);
#13364=VERTEX_POINT('',#63179);
#13365=VERTEX_POINT('',#63180);
#13366=VERTEX_POINT('',#63221);
#13367=VERTEX_POINT('',#63222);
#13368=VERTEX_POINT('',#63263);
#13369=VERTEX_POINT('',#63264);
#13370=VERTEX_POINT('',#63293);
#13371=VERTEX_POINT('',#63294);
#13372=VERTEX_POINT('',#63323);
#13373=VERTEX_POINT('',#63324);
#13374=VERTEX_POINT('',#63365);
#13375=VERTEX_POINT('',#63366);
#13376=VERTEX_POINT('',#63419);
#13377=VERTEX_POINT('',#63420);
#13378=VERTEX_POINT('',#63449);
#13379=VERTEX_POINT('',#63450);
#13380=VERTEX_POINT('',#63491);
#13381=VERTEX_POINT('',#63492);
#13382=VERTEX_POINT('',#63520);
#13383=VERTEX_POINT('',#63521);
#13384=VERTEX_POINT('',#63550);
#13385=VERTEX_POINT('',#63551);
#13386=VERTEX_POINT('',#63593);
#13387=VERTEX_POINT('',#63594);
#13388=VERTEX_POINT('',#63635);
#13389=VERTEX_POINT('',#63636);
#13390=VERTEX_POINT('',#63665);
#13391=VERTEX_POINT('',#63666);
#13392=VERTEX_POINT('',#63694);
#13393=VERTEX_POINT('',#63695);
#13394=VERTEX_POINT('',#63736);
#13395=VERTEX_POINT('',#63737);
#13396=VERTEX_POINT('',#63793);
#13397=VERTEX_POINT('',#63794);
#13398=VERTEX_POINT('',#63822);
#13399=VERTEX_POINT('',#63823);
#13400=VERTEX_POINT('',#63849);
#13401=VERTEX_POINT('',#63850);
#13402=VERTEX_POINT('',#63878);
#13403=VERTEX_POINT('',#63879);
#13404=VERTEX_POINT('',#63923);
#13405=VERTEX_POINT('',#63924);
#13406=VERTEX_POINT('',#63966);
#13407=VERTEX_POINT('',#63967);
#13408=VERTEX_POINT('',#64011);
#13409=VERTEX_POINT('',#64012);
#13410=VERTEX_POINT('',#64041);
#13411=VERTEX_POINT('',#64042);
#13412=VERTEX_POINT('',#64071);
#13413=VERTEX_POINT('',#64072);
#13414=VERTEX_POINT('',#64100);
#13415=VERTEX_POINT('',#64101);
#13416=VERTEX_POINT('',#64146);
#13417=VERTEX_POINT('',#64147);
#13418=VERTEX_POINT('',#64176);
#13419=VERTEX_POINT('',#64177);
#13420=VERTEX_POINT('',#64206);
#13421=VERTEX_POINT('',#64207);
#13422=VERTEX_POINT('',#64235);
#13423=VERTEX_POINT('',#64236);
#13424=VERTEX_POINT('',#64277);
#13425=VERTEX_POINT('',#64278);
#13426=VERTEX_POINT('',#64320);
#13427=VERTEX_POINT('',#64321);
#13428=VERTEX_POINT('',#64362);
#13429=VERTEX_POINT('',#64363);
#13430=VERTEX_POINT('',#64392);
#13431=VERTEX_POINT('',#64393);
#13432=VERTEX_POINT('',#64422);
#13433=VERTEX_POINT('',#64423);
#13434=VERTEX_POINT('',#64451);
#13435=VERTEX_POINT('',#64452);
#13436=VERTEX_POINT('',#64493);
#13437=VERTEX_POINT('',#64494);
#13438=VERTEX_POINT('',#64524);
#13439=VERTEX_POINT('',#64525);
#13440=VERTEX_POINT('',#64554);
#13441=VERTEX_POINT('',#64555);
#13442=VERTEX_POINT('',#64596);
#13443=VERTEX_POINT('',#64597);
#13444=VERTEX_POINT('',#64638);
#13445=VERTEX_POINT('',#64639);
#13446=VERTEX_POINT('',#64669);
#13447=VERTEX_POINT('',#64670);
#13448=VERTEX_POINT('',#64711);
#13449=VERTEX_POINT('',#64712);
#13450=VERTEX_POINT('',#64741);
#13451=VERTEX_POINT('',#64742);
#13452=VERTEX_POINT('',#64770);
#13453=VERTEX_POINT('',#64771);
#13454=VERTEX_POINT('',#64800);
#13455=VERTEX_POINT('',#64801);
#13456=VERTEX_POINT('',#64847);
#13457=VERTEX_POINT('',#64848);
#13458=VERTEX_POINT('',#64852);
#13459=VERTEX_POINT('',#64854);
#13460=VERTEX_POINT('',#64865);
#13461=VERTEX_POINT('',#64869);
#13462=VERTEX_POINT('',#64880);
#13463=VERTEX_POINT('',#64884);
#13464=VERTEX_POINT('',#64895);
#13465=VERTEX_POINT('',#64899);
#13466=VERTEX_POINT('',#64910);
#13467=VERTEX_POINT('',#64914);
#13468=VERTEX_POINT('',#64925);
#13469=VERTEX_POINT('',#64929);
#13470=VERTEX_POINT('',#64940);
#13471=VERTEX_POINT('',#64944);
#13472=VERTEX_POINT('',#64955);
#13473=VERTEX_POINT('',#64959);
#13474=VERTEX_POINT('',#64982);
#13475=VERTEX_POINT('',#64983);
#13476=VERTEX_POINT('',#64987);
#13477=VERTEX_POINT('',#64989);
#13478=VERTEX_POINT('',#65000);
#13479=VERTEX_POINT('',#65004);
#13480=VERTEX_POINT('',#65015);
#13481=VERTEX_POINT('',#65019);
#13482=VERTEX_POINT('',#65030);
#13483=VERTEX_POINT('',#65034);
#13484=VERTEX_POINT('',#65045);
#13485=VERTEX_POINT('',#65049);
#13486=VERTEX_POINT('',#65060);
#13487=VERTEX_POINT('',#65064);
#13488=VERTEX_POINT('',#65075);
#13489=VERTEX_POINT('',#65079);
#13490=VERTEX_POINT('',#65102);
#13491=VERTEX_POINT('',#65103);
#13492=VERTEX_POINT('',#65107);
#13493=VERTEX_POINT('',#65109);
#13494=VERTEX_POINT('',#65120);
#13495=VERTEX_POINT('',#65124);
#13496=VERTEX_POINT('',#65135);
#13497=VERTEX_POINT('',#65139);
#13498=VERTEX_POINT('',#65150);
#13499=VERTEX_POINT('',#65154);
#13500=VERTEX_POINT('',#65165);
#13501=VERTEX_POINT('',#65169);
#13502=VERTEX_POINT('',#65180);
#13503=VERTEX_POINT('',#65184);
#13504=VERTEX_POINT('',#65195);
#13505=VERTEX_POINT('',#65199);
#13506=VERTEX_POINT('',#65210);
#13507=VERTEX_POINT('',#65214);
#13508=VERTEX_POINT('',#65225);
#13509=VERTEX_POINT('',#65229);
#13510=VERTEX_POINT('',#65240);
#13511=VERTEX_POINT('',#65244);
#13512=VERTEX_POINT('',#65255);
#13513=VERTEX_POINT('',#65259);
#13514=VERTEX_POINT('',#65270);
#13515=VERTEX_POINT('',#65274);
#13516=VERTEX_POINT('',#65285);
#13517=VERTEX_POINT('',#65289);
#13518=VERTEX_POINT('',#65300);
#13519=VERTEX_POINT('',#65304);
#13520=VERTEX_POINT('',#65315);
#13521=VERTEX_POINT('',#65319);
#13522=VERTEX_POINT('',#65338);
#13523=VERTEX_POINT('',#65339);
#13524=VERTEX_POINT('',#65341);
#13525=VERTEX_POINT('',#65343);
#13526=VERTEX_POINT('',#65347);
#13527=VERTEX_POINT('',#65349);
#13528=VERTEX_POINT('',#65353);
#13529=VERTEX_POINT('',#65355);
#13530=VERTEX_POINT('',#65368);
#13531=VERTEX_POINT('',#65369);
#13532=VERTEX_POINT('',#65373);
#13533=VERTEX_POINT('',#65375);
#13534=VERTEX_POINT('',#65386);
#13535=VERTEX_POINT('',#65390);
#13536=VERTEX_POINT('',#65401);
#13537=VERTEX_POINT('',#65405);
#13538=VERTEX_POINT('',#65416);
#13539=VERTEX_POINT('',#65420);
#13540=VERTEX_POINT('',#65431);
#13541=VERTEX_POINT('',#65435);
#13542=VERTEX_POINT('',#65446);
#13543=VERTEX_POINT('',#65450);
#13544=VERTEX_POINT('',#65461);
#13545=VERTEX_POINT('',#65465);
#13546=VERTEX_POINT('',#65476);
#13547=VERTEX_POINT('',#65480);
#13548=VERTEX_POINT('',#65503);
#13549=VERTEX_POINT('',#65504);
#13550=VERTEX_POINT('',#65508);
#13551=VERTEX_POINT('',#65510);
#13552=VERTEX_POINT('',#65521);
#13553=VERTEX_POINT('',#65525);
#13554=VERTEX_POINT('',#65536);
#13555=VERTEX_POINT('',#65540);
#13556=VERTEX_POINT('',#65551);
#13557=VERTEX_POINT('',#65555);
#13558=VERTEX_POINT('',#65566);
#13559=VERTEX_POINT('',#65570);
#13560=VERTEX_POINT('',#65581);
#13561=VERTEX_POINT('',#65585);
#13562=VERTEX_POINT('',#65596);
#13563=VERTEX_POINT('',#65600);
#13564=VERTEX_POINT('',#65623);
#13565=VERTEX_POINT('',#65624);
#13566=VERTEX_POINT('',#65628);
#13567=VERTEX_POINT('',#65630);
#13568=VERTEX_POINT('',#65641);
#13569=VERTEX_POINT('',#65645);
#13570=VERTEX_POINT('',#65656);
#13571=VERTEX_POINT('',#65660);
#13572=VERTEX_POINT('',#65671);
#13573=VERTEX_POINT('',#65675);
#13574=VERTEX_POINT('',#65686);
#13575=VERTEX_POINT('',#65690);
#13576=VERTEX_POINT('',#65701);
#13577=VERTEX_POINT('',#65705);
#13578=VERTEX_POINT('',#65716);
#13579=VERTEX_POINT('',#65720);
#13580=VERTEX_POINT('',#65731);
#13581=VERTEX_POINT('',#65735);
#13582=VERTEX_POINT('',#65746);
#13583=VERTEX_POINT('',#65750);
#13584=VERTEX_POINT('',#65761);
#13585=VERTEX_POINT('',#65765);
#13586=VERTEX_POINT('',#65776);
#13587=VERTEX_POINT('',#65780);
#13588=VERTEX_POINT('',#65791);
#13589=VERTEX_POINT('',#65795);
#13590=VERTEX_POINT('',#65806);
#13591=VERTEX_POINT('',#65810);
#13592=VERTEX_POINT('',#65821);
#13593=VERTEX_POINT('',#65825);
#13594=VERTEX_POINT('',#65836);
#13595=VERTEX_POINT('',#65840);
#13596=VERTEX_POINT('',#65936);
#13597=VERTEX_POINT('',#65938);
#13598=VERTEX_POINT('',#68172);
#13599=VERTEX_POINT('',#68258);
#13600=VERTEX_POINT('',#68261);
#13601=VERTEX_POINT('',#70503);
#13602=VERTEX_POINT('',#70508);
#13603=VERTEX_POINT('',#70509);
#13604=VERTEX_POINT('',#70511);
#13605=VERTEX_POINT('',#70513);
#13606=VERTEX_POINT('',#70515);
#13607=VERTEX_POINT('',#70517);
#13608=VERTEX_POINT('',#70522);
#13609=VERTEX_POINT('',#70523);
#13610=VERTEX_POINT('',#70527);
#13611=VERTEX_POINT('',#70531);
#13612=VERTEX_POINT('',#70535);
#13613=VERTEX_POINT('',#70539);
#13614=VERTEX_POINT('',#70543);
#13615=VERTEX_POINT('',#70546);
#13616=VERTEX_POINT('',#70567);
#16928=EDGE_CURVE('',#13213,#13214,#8378,.T.);
#16929=EDGE_CURVE('',#13213,#13215,#971,.T.);
#16930=EDGE_CURVE('',#13215,#13216,#2550,.T.);
#16931=EDGE_CURVE('',#13216,#13214,#972,.T.);
#16932=EDGE_CURVE('',#13217,#13218,#8379,.T.);
#16933=EDGE_CURVE('',#13217,#13213,#973,.T.);
#16934=EDGE_CURVE('',#13214,#13218,#974,.T.);
#16935=EDGE_CURVE('',#13219,#13220,#8380,.T.);
#16936=EDGE_CURVE('',#13219,#13217,#975,.T.);
#16937=EDGE_CURVE('',#13218,#13220,#976,.T.);
#16938=EDGE_CURVE('',#13221,#13222,#8381,.T.);
#16939=EDGE_CURVE('',#13221,#13219,#977,.T.);
#16940=EDGE_CURVE('',#13220,#13222,#978,.T.);
#16941=EDGE_CURVE('',#13223,#13224,#8382,.T.);
#16942=EDGE_CURVE('',#13223,#13221,#979,.T.);
#16943=EDGE_CURVE('',#13222,#13224,#980,.T.);
#16944=EDGE_CURVE('',#13225,#13226,#8383,.T.);
#16945=EDGE_CURVE('',#13225,#13223,#981,.T.);
#16946=EDGE_CURVE('',#13224,#13226,#982,.T.);
#16947=EDGE_CURVE('',#13227,#13228,#8384,.T.);
#16948=EDGE_CURVE('',#13227,#13225,#983,.T.);
#16949=EDGE_CURVE('',#13226,#13228,#984,.T.);
#16950=EDGE_CURVE('',#13229,#13230,#8385,.T.);
#16951=EDGE_CURVE('',#13229,#13227,#985,.T.);
#16952=EDGE_CURVE('',#13228,#13230,#986,.T.);
#16953=EDGE_CURVE('',#13231,#13232,#8386,.T.);
#16954=EDGE_CURVE('',#13231,#13229,#987,.T.);
#16955=EDGE_CURVE('',#13230,#13232,#988,.T.);
#16956=EDGE_CURVE('',#13233,#13234,#8387,.T.);
#16957=EDGE_CURVE('',#13233,#13231,#989,.T.);
#16958=EDGE_CURVE('',#13232,#13234,#990,.T.);
#16959=EDGE_CURVE('',#13235,#13236,#8388,.T.);
#16960=EDGE_CURVE('',#13235,#13233,#991,.T.);
#16961=EDGE_CURVE('',#13234,#13236,#992,.T.);
#16962=EDGE_CURVE('',#13237,#13238,#8389,.T.);
#16963=EDGE_CURVE('',#13237,#13235,#993,.T.);
#16964=EDGE_CURVE('',#13236,#13238,#994,.T.);
#16965=EDGE_CURVE('',#13239,#13240,#8390,.T.);
#16966=EDGE_CURVE('',#13239,#13237,#995,.T.);
#16967=EDGE_CURVE('',#13238,#13240,#996,.T.);
#16968=EDGE_CURVE('',#13241,#13242,#8391,.T.);
#16969=EDGE_CURVE('',#13241,#13239,#997,.T.);
#16970=EDGE_CURVE('',#13240,#13242,#998,.T.);
#16971=EDGE_CURVE('',#13243,#13244,#8392,.T.);
#16972=EDGE_CURVE('',#13243,#13241,#999,.T.);
#16973=EDGE_CURVE('',#13242,#13244,#1000,.T.);
#16974=EDGE_CURVE('',#13245,#13246,#8393,.T.);
#16975=EDGE_CURVE('',#13245,#13243,#1001,.T.);
#16976=EDGE_CURVE('',#13244,#13246,#1002,.T.);
#16977=EDGE_CURVE('',#13247,#13248,#8394,.T.);
#16978=EDGE_CURVE('',#13247,#13245,#1003,.T.);
#16979=EDGE_CURVE('',#13246,#13248,#1004,.T.);
#16980=EDGE_CURVE('',#13249,#13250,#8395,.T.);
#16981=EDGE_CURVE('',#13249,#13247,#1005,.T.);
#16982=EDGE_CURVE('',#13248,#13250,#1006,.T.);
#16983=EDGE_CURVE('',#13251,#13252,#8396,.T.);
#16984=EDGE_CURVE('',#13251,#13249,#1007,.T.);
#16985=EDGE_CURVE('',#13250,#13252,#1008,.T.);
#16986=EDGE_CURVE('',#13253,#13254,#8397,.T.);
#16987=EDGE_CURVE('',#13253,#13251,#1009,.T.);
#16988=EDGE_CURVE('',#13252,#13254,#1010,.T.);
#16989=EDGE_CURVE('',#13255,#13256,#8398,.T.);
#16990=EDGE_CURVE('',#13255,#13253,#1011,.T.);
#16991=EDGE_CURVE('',#13254,#13256,#1012,.T.);
#16992=EDGE_CURVE('',#13257,#13258,#8399,.T.);
#16993=EDGE_CURVE('',#13257,#13255,#1013,.T.);
#16994=EDGE_CURVE('',#13256,#13258,#1014,.T.);
#16995=EDGE_CURVE('',#13259,#13260,#8400,.T.);
#16996=EDGE_CURVE('',#13259,#13257,#1015,.T.);
#16997=EDGE_CURVE('',#13258,#13260,#1016,.T.);
#16998=EDGE_CURVE('',#13261,#13262,#8401,.T.);
#16999=EDGE_CURVE('',#13261,#13259,#1017,.T.);
#17000=EDGE_CURVE('',#13260,#13262,#1018,.T.);
#17001=EDGE_CURVE('',#13263,#13264,#8402,.T.);
#17002=EDGE_CURVE('',#13263,#13261,#1019,.T.);
#17003=EDGE_CURVE('',#13262,#13264,#1020,.T.);
#17004=EDGE_CURVE('',#13265,#13266,#8403,.T.);
#17005=EDGE_CURVE('',#13265,#13263,#1021,.T.);
#17006=EDGE_CURVE('',#13264,#13266,#1022,.T.);
#17007=EDGE_CURVE('',#13267,#13268,#8404,.T.);
#17008=EDGE_CURVE('',#13267,#13265,#1023,.T.);
#17009=EDGE_CURVE('',#13266,#13268,#1024,.T.);
#17010=EDGE_CURVE('',#13269,#13270,#8405,.T.);
#17011=EDGE_CURVE('',#13269,#13267,#1025,.T.);
#17012=EDGE_CURVE('',#13268,#13270,#1026,.T.);
#17013=EDGE_CURVE('',#13271,#13272,#8406,.T.);
#17014=EDGE_CURVE('',#13271,#13269,#1027,.T.);
#17015=EDGE_CURVE('',#13270,#13272,#1028,.T.);
#17016=EDGE_CURVE('',#13273,#13274,#8407,.T.);
#17017=EDGE_CURVE('',#13273,#13271,#1029,.T.);
#17018=EDGE_CURVE('',#13272,#13274,#1030,.T.);
#17019=EDGE_CURVE('',#13275,#13276,#8408,.T.);
#17020=EDGE_CURVE('',#13275,#13273,#1031,.T.);
#17021=EDGE_CURVE('',#13274,#13276,#1032,.T.);
#17022=EDGE_CURVE('',#13277,#13278,#8409,.T.);
#17023=EDGE_CURVE('',#13277,#13275,#1033,.T.);
#17024=EDGE_CURVE('',#13276,#13278,#1034,.T.);
#17025=EDGE_CURVE('',#13279,#13280,#8410,.T.);
#17026=EDGE_CURVE('',#13279,#13277,#1035,.T.);
#17027=EDGE_CURVE('',#13278,#13280,#1036,.T.);
#17028=EDGE_CURVE('',#13281,#13282,#8411,.T.);
#17029=EDGE_CURVE('',#13281,#13279,#1037,.T.);
#17030=EDGE_CURVE('',#13280,#13282,#1038,.T.);
#17031=EDGE_CURVE('',#13283,#13284,#8412,.T.);
#17032=EDGE_CURVE('',#13283,#13281,#1039,.T.);
#17033=EDGE_CURVE('',#13282,#13284,#1040,.T.);
#17034=EDGE_CURVE('',#13285,#13286,#8413,.T.);
#17035=EDGE_CURVE('',#13285,#13283,#1041,.T.);
#17036=EDGE_CURVE('',#13284,#13286,#1042,.T.);
#17037=EDGE_CURVE('',#13287,#13288,#8414,.T.);
#17038=EDGE_CURVE('',#13287,#13285,#1043,.T.);
#17039=EDGE_CURVE('',#13286,#13288,#1044,.T.);
#17040=EDGE_CURVE('',#13289,#13290,#8415,.T.);
#17041=EDGE_CURVE('',#13289,#13287,#1045,.T.);
#17042=EDGE_CURVE('',#13288,#13290,#1046,.T.);
#17043=EDGE_CURVE('',#13291,#13292,#8416,.T.);
#17044=EDGE_CURVE('',#13291,#13289,#1047,.T.);
#17045=EDGE_CURVE('',#13290,#13292,#1048,.T.);
#17046=EDGE_CURVE('',#13293,#13294,#8417,.T.);
#17047=EDGE_CURVE('',#13293,#13291,#1049,.T.);
#17048=EDGE_CURVE('',#13292,#13294,#1050,.T.);
#17049=EDGE_CURVE('',#13295,#13296,#8418,.T.);
#17050=EDGE_CURVE('',#13295,#13293,#1051,.T.);
#17051=EDGE_CURVE('',#13294,#13296,#1052,.T.);
#17052=EDGE_CURVE('',#13297,#13298,#8419,.T.);
#17053=EDGE_CURVE('',#13297,#13295,#1053,.T.);
#17054=EDGE_CURVE('',#13296,#13298,#1054,.T.);
#17055=EDGE_CURVE('',#13299,#13300,#8420,.T.);
#17056=EDGE_CURVE('',#13299,#13297,#1055,.T.);
#17057=EDGE_CURVE('',#13298,#13300,#1056,.T.);
#17058=EDGE_CURVE('',#13301,#13302,#8421,.T.);
#17059=EDGE_CURVE('',#13301,#13299,#1057,.T.);
#17060=EDGE_CURVE('',#13300,#13302,#1058,.T.);
#17061=EDGE_CURVE('',#13303,#13304,#8422,.T.);
#17062=EDGE_CURVE('',#13303,#13301,#1059,.T.);
#17063=EDGE_CURVE('',#13302,#13304,#1060,.T.);
#17064=EDGE_CURVE('',#13305,#13306,#8423,.T.);
#17065=EDGE_CURVE('',#13305,#13303,#1061,.T.);
#17066=EDGE_CURVE('',#13304,#13306,#1062,.T.);
#17067=EDGE_CURVE('',#13307,#13308,#8424,.T.);
#17068=EDGE_CURVE('',#13307,#13305,#1063,.T.);
#17069=EDGE_CURVE('',#13306,#13308,#1064,.T.);
#17070=EDGE_CURVE('',#13309,#13310,#8425,.T.);
#17071=EDGE_CURVE('',#13309,#13307,#1065,.T.);
#17072=EDGE_CURVE('',#13308,#13310,#1066,.T.);
#17073=EDGE_CURVE('',#13311,#13312,#8426,.T.);
#17074=EDGE_CURVE('',#13311,#13309,#1067,.T.);
#17075=EDGE_CURVE('',#13310,#13312,#1068,.T.);
#17076=EDGE_CURVE('',#13313,#13314,#8427,.T.);
#17077=EDGE_CURVE('',#13313,#13311,#1069,.T.);
#17078=EDGE_CURVE('',#13312,#13314,#1070,.T.);
#17079=EDGE_CURVE('',#13315,#13316,#8428,.T.);
#17080=EDGE_CURVE('',#13315,#13313,#1071,.T.);
#17081=EDGE_CURVE('',#13314,#13316,#1072,.T.);
#17082=EDGE_CURVE('',#13317,#13318,#8429,.T.);
#17083=EDGE_CURVE('',#13317,#13315,#1073,.T.);
#17084=EDGE_CURVE('',#13316,#13318,#1074,.T.);
#17085=EDGE_CURVE('',#13319,#13320,#8430,.T.);
#17086=EDGE_CURVE('',#13319,#13317,#1075,.T.);
#17087=EDGE_CURVE('',#13318,#13320,#1076,.T.);
#17088=EDGE_CURVE('',#13321,#13322,#8431,.T.);
#17089=EDGE_CURVE('',#13321,#13319,#1077,.T.);
#17090=EDGE_CURVE('',#13320,#13322,#1078,.T.);
#17091=EDGE_CURVE('',#13323,#13324,#8432,.T.);
#17092=EDGE_CURVE('',#13323,#13321,#1079,.T.);
#17093=EDGE_CURVE('',#13322,#13324,#1080,.T.);
#17094=EDGE_CURVE('',#13325,#13326,#8433,.T.);
#17095=EDGE_CURVE('',#13325,#13323,#1081,.T.);
#17096=EDGE_CURVE('',#13324,#13326,#1082,.T.);
#17097=EDGE_CURVE('',#13327,#13328,#8434,.T.);
#17098=EDGE_CURVE('',#13327,#13325,#1083,.T.);
#17099=EDGE_CURVE('',#13326,#13328,#1084,.T.);
#17100=EDGE_CURVE('',#13329,#13330,#8435,.T.);
#17101=EDGE_CURVE('',#13329,#13327,#1085,.T.);
#17102=EDGE_CURVE('',#13328,#13330,#1086,.T.);
#17103=EDGE_CURVE('',#13331,#13332,#8436,.T.);
#17104=EDGE_CURVE('',#13331,#13329,#1087,.T.);
#17105=EDGE_CURVE('',#13330,#13332,#1088,.T.);
#17106=EDGE_CURVE('',#13333,#13334,#8437,.T.);
#17107=EDGE_CURVE('',#13335,#13333,#2551,.T.);
#17108=EDGE_CURVE('',#13335,#13331,#1089,.T.);
#17109=EDGE_CURVE('',#13332,#13334,#1090,.T.);
#17110=EDGE_CURVE('',#13336,#13337,#8438,.T.);
#17111=EDGE_CURVE('',#13336,#13338,#1091,.T.);
#17112=EDGE_CURVE('',#13339,#13338,#2552,.T.);
#17113=EDGE_CURVE('',#13337,#13339,#1092,.T.);
#17114=EDGE_CURVE('',#13340,#13341,#8439,.T.);
#17115=EDGE_CURVE('',#13340,#13336,#1093,.T.);
#17116=EDGE_CURVE('',#13341,#13337,#1094,.T.);
#17117=EDGE_CURVE('',#13342,#13343,#8440,.T.);
#17118=EDGE_CURVE('',#13342,#13340,#1095,.T.);
#17119=EDGE_CURVE('',#13343,#13341,#1096,.T.);
#17120=EDGE_CURVE('',#13344,#13345,#8441,.T.);
#17121=EDGE_CURVE('',#13344,#13342,#1097,.T.);
#17122=EDGE_CURVE('',#13345,#13343,#1098,.T.);
#17123=EDGE_CURVE('',#13346,#13347,#8442,.T.);
#17124=EDGE_CURVE('',#13346,#13344,#1099,.T.);
#17125=EDGE_CURVE('',#13347,#13345,#1100,.T.);
#17126=EDGE_CURVE('',#13348,#13349,#8443,.T.);
#17127=EDGE_CURVE('',#13348,#13346,#1101,.T.);
#17128=EDGE_CURVE('',#13349,#13347,#1102,.T.);
#17129=EDGE_CURVE('',#13350,#13351,#8444,.T.);
#17130=EDGE_CURVE('',#13350,#13348,#1103,.T.);
#17131=EDGE_CURVE('',#13351,#13349,#1104,.T.);
#17132=EDGE_CURVE('',#13352,#13353,#8445,.T.);
#17133=EDGE_CURVE('',#13352,#13350,#1105,.T.);
#17134=EDGE_CURVE('',#13353,#13351,#1106,.T.);
#17135=EDGE_CURVE('',#13354,#13355,#8446,.T.);
#17136=EDGE_CURVE('',#13354,#13352,#1107,.T.);
#17137=EDGE_CURVE('',#13355,#13353,#1108,.T.);
#17138=EDGE_CURVE('',#13356,#13357,#8447,.T.);
#17139=EDGE_CURVE('',#13356,#13354,#1109,.T.);
#17140=EDGE_CURVE('',#13357,#13355,#1110,.T.);
#17141=EDGE_CURVE('',#13358,#13359,#8448,.T.);
#17142=EDGE_CURVE('',#13358,#13356,#1111,.T.);
#17143=EDGE_CURVE('',#13359,#13357,#1112,.T.);
#17144=EDGE_CURVE('',#13360,#13361,#8449,.T.);
#17145=EDGE_CURVE('',#13360,#13358,#1113,.T.);
#17146=EDGE_CURVE('',#13361,#13359,#1114,.T.);
#17147=EDGE_CURVE('',#13362,#13363,#8450,.T.);
#17148=EDGE_CURVE('',#13362,#13360,#1115,.T.);
#17149=EDGE_CURVE('',#13363,#13361,#1116,.T.);
#17150=EDGE_CURVE('',#13364,#13365,#8451,.T.);
#17151=EDGE_CURVE('',#13364,#13362,#1117,.T.);
#17152=EDGE_CURVE('',#13365,#13363,#1118,.T.);
#17153=EDGE_CURVE('',#13366,#13367,#8452,.T.);
#17154=EDGE_CURVE('',#13366,#13364,#1119,.T.);
#17155=EDGE_CURVE('',#13367,#13365,#1120,.T.);
#17156=EDGE_CURVE('',#13368,#13369,#8453,.T.);
#17157=EDGE_CURVE('',#13368,#13366,#1121,.T.);
#17158=EDGE_CURVE('',#13369,#13367,#1122,.T.);
#17159=EDGE_CURVE('',#13370,#13371,#8454,.T.);
#17160=EDGE_CURVE('',#13370,#13368,#1123,.T.);
#17161=EDGE_CURVE('',#13371,#13369,#1124,.T.);
#17162=EDGE_CURVE('',#13372,#13373,#8455,.T.);
#17163=EDGE_CURVE('',#13372,#13370,#1125,.T.);
#17164=EDGE_CURVE('',#13373,#13371,#1126,.T.);
#17165=EDGE_CURVE('',#13374,#13375,#8456,.T.);
#17166=EDGE_CURVE('',#13374,#13372,#1127,.T.);
#17167=EDGE_CURVE('',#13375,#13373,#1128,.T.);
#17168=EDGE_CURVE('',#13376,#13377,#8457,.T.);
#17169=EDGE_CURVE('',#13376,#13374,#1129,.T.);
#17170=EDGE_CURVE('',#13377,#13375,#1130,.T.);
#17171=EDGE_CURVE('',#13378,#13379,#8458,.T.);
#17172=EDGE_CURVE('',#13378,#13376,#1131,.T.);
#17173=EDGE_CURVE('',#13379,#13377,#1132,.T.);
#17174=EDGE_CURVE('',#13380,#13381,#8459,.T.);
#17175=EDGE_CURVE('',#13380,#13378,#1133,.T.);
#17176=EDGE_CURVE('',#13381,#13379,#1134,.T.);
#17177=EDGE_CURVE('',#13382,#13383,#8460,.T.);
#17178=EDGE_CURVE('',#13382,#13380,#1135,.T.);
#17179=EDGE_CURVE('',#13383,#13381,#1136,.T.);
#17180=EDGE_CURVE('',#13384,#13385,#8461,.T.);
#17181=EDGE_CURVE('',#13384,#13382,#1137,.T.);
#17182=EDGE_CURVE('',#13385,#13383,#1138,.T.);
#17183=EDGE_CURVE('',#13386,#13387,#8462,.T.);
#17184=EDGE_CURVE('',#13386,#13384,#1139,.T.);
#17185=EDGE_CURVE('',#13387,#13385,#1140,.T.);
#17186=EDGE_CURVE('',#13388,#13389,#8463,.T.);
#17187=EDGE_CURVE('',#13388,#13386,#1141,.T.);
#17188=EDGE_CURVE('',#13389,#13387,#1142,.T.);
#17189=EDGE_CURVE('',#13390,#13391,#8464,.T.);
#17190=EDGE_CURVE('',#13390,#13388,#1143,.T.);
#17191=EDGE_CURVE('',#13391,#13389,#1144,.T.);
#17192=EDGE_CURVE('',#13392,#13393,#8465,.T.);
#17193=EDGE_CURVE('',#13392,#13390,#1145,.T.);
#17194=EDGE_CURVE('',#13393,#13391,#1146,.T.);
#17195=EDGE_CURVE('',#13394,#13395,#8466,.T.);
#17196=EDGE_CURVE('',#13394,#13392,#1147,.T.);
#17197=EDGE_CURVE('',#13395,#13393,#1148,.T.);
#17198=EDGE_CURVE('',#13396,#13397,#8467,.T.);
#17199=EDGE_CURVE('',#13396,#13394,#1149,.T.);
#17200=EDGE_CURVE('',#13397,#13395,#1150,.T.);
#17201=EDGE_CURVE('',#13398,#13399,#8468,.T.);
#17202=EDGE_CURVE('',#13398,#13396,#1151,.T.);
#17203=EDGE_CURVE('',#13399,#13397,#1152,.T.);
#17204=EDGE_CURVE('',#13400,#13401,#8469,.T.);
#17205=EDGE_CURVE('',#13400,#13398,#1153,.T.);
#17206=EDGE_CURVE('',#13401,#13399,#1154,.T.);
#17207=EDGE_CURVE('',#13402,#13403,#8470,.T.);
#17208=EDGE_CURVE('',#13402,#13400,#1155,.T.);
#17209=EDGE_CURVE('',#13403,#13401,#1156,.T.);
#17210=EDGE_CURVE('',#13404,#13405,#8471,.T.);
#17211=EDGE_CURVE('',#13404,#13402,#1157,.T.);
#17212=EDGE_CURVE('',#13405,#13403,#1158,.T.);
#17213=EDGE_CURVE('',#13406,#13407,#8472,.T.);
#17214=EDGE_CURVE('',#13406,#13404,#1159,.T.);
#17215=EDGE_CURVE('',#13407,#13405,#1160,.T.);
#17216=EDGE_CURVE('',#13408,#13409,#8473,.T.);
#17217=EDGE_CURVE('',#13408,#13406,#1161,.T.);
#17218=EDGE_CURVE('',#13409,#13407,#1162,.T.);
#17219=EDGE_CURVE('',#13410,#13411,#8474,.T.);
#17220=EDGE_CURVE('',#13410,#13408,#1163,.T.);
#17221=EDGE_CURVE('',#13411,#13409,#1164,.T.);
#17222=EDGE_CURVE('',#13412,#13413,#8475,.T.);
#17223=EDGE_CURVE('',#13412,#13410,#1165,.T.);
#17224=EDGE_CURVE('',#13413,#13411,#1166,.T.);
#17225=EDGE_CURVE('',#13414,#13415,#8476,.T.);
#17226=EDGE_CURVE('',#13414,#13412,#1167,.T.);
#17227=EDGE_CURVE('',#13415,#13413,#1168,.T.);
#17228=EDGE_CURVE('',#13416,#13417,#8477,.T.);
#17229=EDGE_CURVE('',#13416,#13414,#1169,.T.);
#17230=EDGE_CURVE('',#13417,#13415,#1170,.T.);
#17231=EDGE_CURVE('',#13418,#13419,#8478,.T.);
#17232=EDGE_CURVE('',#13418,#13416,#1171,.T.);
#17233=EDGE_CURVE('',#13419,#13417,#1172,.T.);
#17234=EDGE_CURVE('',#13420,#13421,#8479,.T.);
#17235=EDGE_CURVE('',#13420,#13418,#1173,.T.);
#17236=EDGE_CURVE('',#13421,#13419,#1174,.T.);
#17237=EDGE_CURVE('',#13422,#13423,#8480,.T.);
#17238=EDGE_CURVE('',#13422,#13420,#1175,.T.);
#17239=EDGE_CURVE('',#13423,#13421,#1176,.T.);
#17240=EDGE_CURVE('',#13424,#13425,#8481,.T.);
#17241=EDGE_CURVE('',#13424,#13422,#1177,.T.);
#17242=EDGE_CURVE('',#13425,#13423,#1178,.T.);
#17243=EDGE_CURVE('',#13426,#13427,#8482,.T.);
#17244=EDGE_CURVE('',#13426,#13424,#1179,.T.);
#17245=EDGE_CURVE('',#13427,#13425,#1180,.T.);
#17246=EDGE_CURVE('',#13428,#13429,#8483,.T.);
#17247=EDGE_CURVE('',#13428,#13426,#1181,.T.);
#17248=EDGE_CURVE('',#13429,#13427,#1182,.T.);
#17249=EDGE_CURVE('',#13430,#13431,#8484,.T.);
#17250=EDGE_CURVE('',#13430,#13428,#1183,.T.);
#17251=EDGE_CURVE('',#13431,#13429,#1184,.T.);
#17252=EDGE_CURVE('',#13432,#13433,#8485,.T.);
#17253=EDGE_CURVE('',#13432,#13430,#1185,.T.);
#17254=EDGE_CURVE('',#13433,#13431,#1186,.T.);
#17255=EDGE_CURVE('',#13434,#13435,#8486,.T.);
#17256=EDGE_CURVE('',#13434,#13432,#1187,.T.);
#17257=EDGE_CURVE('',#13435,#13433,#1188,.T.);
#17258=EDGE_CURVE('',#13436,#13437,#8487,.T.);
#17259=EDGE_CURVE('',#13436,#13434,#1189,.T.);
#17260=EDGE_CURVE('',#13437,#13435,#1190,.T.);
#17261=EDGE_CURVE('',#13438,#13439,#8488,.T.);
#17262=EDGE_CURVE('',#13438,#13436,#1191,.T.);
#17263=EDGE_CURVE('',#13439,#13437,#1192,.T.);
#17264=EDGE_CURVE('',#13440,#13441,#8489,.T.);
#17265=EDGE_CURVE('',#13440,#13438,#1193,.T.);
#17266=EDGE_CURVE('',#13441,#13439,#1194,.T.);
#17267=EDGE_CURVE('',#13442,#13443,#8490,.T.);
#17268=EDGE_CURVE('',#13442,#13440,#1195,.T.);
#17269=EDGE_CURVE('',#13443,#13441,#1196,.T.);
#17270=EDGE_CURVE('',#13444,#13445,#8491,.T.);
#17271=EDGE_CURVE('',#13444,#13442,#1197,.T.);
#17272=EDGE_CURVE('',#13445,#13443,#1198,.T.);
#17273=EDGE_CURVE('',#13446,#13447,#8492,.T.);
#17274=EDGE_CURVE('',#13446,#13444,#1199,.T.);
#17275=EDGE_CURVE('',#13447,#13445,#1200,.T.);
#17276=EDGE_CURVE('',#13448,#13449,#8493,.T.);
#17277=EDGE_CURVE('',#13448,#13446,#1201,.T.);
#17278=EDGE_CURVE('',#13449,#13447,#1202,.T.);
#17279=EDGE_CURVE('',#13450,#13451,#8494,.T.);
#17280=EDGE_CURVE('',#13450,#13448,#1203,.T.);
#17281=EDGE_CURVE('',#13451,#13449,#1204,.T.);
#17282=EDGE_CURVE('',#13452,#13453,#8495,.T.);
#17283=EDGE_CURVE('',#13452,#13450,#1205,.T.);
#17284=EDGE_CURVE('',#13453,#13451,#1206,.T.);
#17285=EDGE_CURVE('',#13454,#13455,#8496,.T.);
#17286=EDGE_CURVE('',#13454,#13452,#1207,.T.);
#17287=EDGE_CURVE('',#13455,#13453,#1208,.T.);
#17288=EDGE_CURVE('',#13456,#13457,#1209,.T.);
#17289=EDGE_CURVE('',#13456,#13458,#8497,.T.);
#17290=EDGE_CURVE('',#13458,#13459,#1210,.T.);
#17291=EDGE_CURVE('',#13457,#13459,#8498,.T.);
#17292=EDGE_CURVE('',#13460,#13456,#1211,.T.);
#17293=EDGE_CURVE('',#13460,#13461,#8499,.T.);
#17294=EDGE_CURVE('',#13461,#13458,#1212,.T.);
#17295=EDGE_CURVE('',#13462,#13460,#1213,.T.);
#17296=EDGE_CURVE('',#13462,#13463,#8500,.T.);
#17297=EDGE_CURVE('',#13463,#13461,#1214,.T.);
#17298=EDGE_CURVE('',#13464,#13462,#1215,.T.);
#17299=EDGE_CURVE('',#13464,#13465,#8501,.T.);
#17300=EDGE_CURVE('',#13465,#13463,#1216,.T.);
#17301=EDGE_CURVE('',#13466,#13464,#1217,.T.);
#17302=EDGE_CURVE('',#13466,#13467,#8502,.T.);
#17303=EDGE_CURVE('',#13467,#13465,#1218,.T.);
#17304=EDGE_CURVE('',#13468,#13466,#1219,.T.);
#17305=EDGE_CURVE('',#13468,#13469,#8503,.T.);
#17306=EDGE_CURVE('',#13469,#13467,#1220,.T.);
#17307=EDGE_CURVE('',#13470,#13468,#1221,.T.);
#17308=EDGE_CURVE('',#13470,#13471,#8504,.T.);
#17309=EDGE_CURVE('',#13471,#13469,#1222,.T.);
#17310=EDGE_CURVE('',#13472,#13470,#1223,.T.);
#17311=EDGE_CURVE('',#13472,#13473,#8505,.T.);
#17312=EDGE_CURVE('',#13473,#13471,#1224,.T.);
#17313=EDGE_CURVE('',#13457,#13472,#1225,.T.);
#17314=EDGE_CURVE('',#13459,#13473,#1226,.T.);
#17315=EDGE_CURVE('',#13474,#13475,#1227,.T.);
#17316=EDGE_CURVE('',#13474,#13476,#8506,.T.);
#17317=EDGE_CURVE('',#13476,#13477,#1228,.T.);
#17318=EDGE_CURVE('',#13475,#13477,#8507,.T.);
#17319=EDGE_CURVE('',#13478,#13474,#1229,.T.);
#17320=EDGE_CURVE('',#13478,#13479,#8508,.T.);
#17321=EDGE_CURVE('',#13479,#13476,#1230,.T.);
#17322=EDGE_CURVE('',#13480,#13478,#1231,.T.);
#17323=EDGE_CURVE('',#13480,#13481,#8509,.T.);
#17324=EDGE_CURVE('',#13481,#13479,#1232,.T.);
#17325=EDGE_CURVE('',#13482,#13480,#1233,.T.);
#17326=EDGE_CURVE('',#13482,#13483,#8510,.T.);
#17327=EDGE_CURVE('',#13483,#13481,#1234,.T.);
#17328=EDGE_CURVE('',#13484,#13482,#1235,.T.);
#17329=EDGE_CURVE('',#13484,#13485,#8511,.T.);
#17330=EDGE_CURVE('',#13485,#13483,#1236,.T.);
#17331=EDGE_CURVE('',#13486,#13484,#1237,.T.);
#17332=EDGE_CURVE('',#13486,#13487,#8512,.T.);
#17333=EDGE_CURVE('',#13487,#13485,#1238,.T.);
#17334=EDGE_CURVE('',#13488,#13486,#1239,.T.);
#17335=EDGE_CURVE('',#13488,#13489,#8513,.T.);
#17336=EDGE_CURVE('',#13489,#13487,#1240,.T.);
#17337=EDGE_CURVE('',#13475,#13488,#1241,.T.);
#17338=EDGE_CURVE('',#13477,#13489,#1242,.T.);
#17339=EDGE_CURVE('',#13490,#13491,#1243,.T.);
#17340=EDGE_CURVE('',#13490,#13492,#8514,.T.);
#17341=EDGE_CURVE('',#13492,#13493,#1244,.T.);
#17342=EDGE_CURVE('',#13491,#13493,#8515,.T.);
#17343=EDGE_CURVE('',#13494,#13490,#1245,.T.);
#17344=EDGE_CURVE('',#13494,#13495,#8516,.T.);
#17345=EDGE_CURVE('',#13495,#13492,#1246,.T.);
#17346=EDGE_CURVE('',#13496,#13494,#1247,.T.);
#17347=EDGE_CURVE('',#13496,#13497,#8517,.T.);
#17348=EDGE_CURVE('',#13497,#13495,#1248,.T.);
#17349=EDGE_CURVE('',#13498,#13496,#1249,.T.);
#17350=EDGE_CURVE('',#13498,#13499,#8518,.T.);
#17351=EDGE_CURVE('',#13499,#13497,#1250,.T.);
#17352=EDGE_CURVE('',#13500,#13498,#1251,.T.);
#17353=EDGE_CURVE('',#13500,#13501,#8519,.T.);
#17354=EDGE_CURVE('',#13501,#13499,#1252,.T.);
#17355=EDGE_CURVE('',#13502,#13500,#1253,.T.);
#17356=EDGE_CURVE('',#13502,#13503,#8520,.T.);
#17357=EDGE_CURVE('',#13503,#13501,#1254,.T.);
#17358=EDGE_CURVE('',#13504,#13502,#1255,.T.);
#17359=EDGE_CURVE('',#13504,#13505,#8521,.T.);
#17360=EDGE_CURVE('',#13505,#13503,#1256,.T.);
#17361=EDGE_CURVE('',#13506,#13504,#1257,.T.);
#17362=EDGE_CURVE('',#13506,#13507,#8522,.T.);
#17363=EDGE_CURVE('',#13507,#13505,#1258,.T.);
#17364=EDGE_CURVE('',#13508,#13506,#1259,.T.);
#17365=EDGE_CURVE('',#13508,#13509,#8523,.T.);
#17366=EDGE_CURVE('',#13509,#13507,#1260,.T.);
#17367=EDGE_CURVE('',#13510,#13508,#1261,.T.);
#17368=EDGE_CURVE('',#13510,#13511,#8524,.T.);
#17369=EDGE_CURVE('',#13511,#13509,#1262,.T.);
#17370=EDGE_CURVE('',#13512,#13510,#1263,.T.);
#17371=EDGE_CURVE('',#13512,#13513,#8525,.T.);
#17372=EDGE_CURVE('',#13513,#13511,#1264,.T.);
#17373=EDGE_CURVE('',#13514,#13512,#1265,.T.);
#17374=EDGE_CURVE('',#13514,#13515,#8526,.T.);
#17375=EDGE_CURVE('',#13515,#13513,#1266,.T.);
#17376=EDGE_CURVE('',#13516,#13514,#1267,.T.);
#17377=EDGE_CURVE('',#13516,#13517,#8527,.T.);
#17378=EDGE_CURVE('',#13517,#13515,#1268,.T.);
#17379=EDGE_CURVE('',#13518,#13516,#1269,.T.);
#17380=EDGE_CURVE('',#13518,#13519,#8528,.T.);
#17381=EDGE_CURVE('',#13519,#13517,#1270,.T.);
#17382=EDGE_CURVE('',#13520,#13518,#1271,.T.);
#17383=EDGE_CURVE('',#13520,#13521,#8529,.T.);
#17384=EDGE_CURVE('',#13521,#13519,#1272,.T.);
#17385=EDGE_CURVE('',#13491,#13520,#1273,.T.);
#17386=EDGE_CURVE('',#13493,#13521,#1274,.T.);
#17387=EDGE_CURVE('',#13522,#13523,#8530,.T.);
#17388=EDGE_CURVE('',#13522,#13524,#8531,.T.);
#17389=EDGE_CURVE('',#13524,#13525,#8532,.T.);
#17390=EDGE_CURVE('',#13523,#13525,#8533,.T.);
#17391=EDGE_CURVE('',#13526,#13522,#8534,.T.);
#17392=EDGE_CURVE('',#13526,#13527,#8535,.T.);
#17393=EDGE_CURVE('',#13527,#13524,#8536,.T.);
#17394=EDGE_CURVE('',#13528,#13526,#8537,.T.);
#17395=EDGE_CURVE('',#13528,#13529,#8538,.T.);
#17396=EDGE_CURVE('',#13529,#13527,#8539,.T.);
#17397=EDGE_CURVE('',#13523,#13528,#8540,.T.);
#17398=EDGE_CURVE('',#13525,#13529,#8541,.T.);
#17399=EDGE_CURVE('',#13530,#13531,#1275,.T.);
#17400=EDGE_CURVE('',#13530,#13532,#8542,.T.);
#17401=EDGE_CURVE('',#13532,#13533,#1276,.T.);
#17402=EDGE_CURVE('',#13531,#13533,#8543,.T.);
#17403=EDGE_CURVE('',#13534,#13530,#1277,.T.);
#17404=EDGE_CURVE('',#13534,#13535,#8544,.T.);
#17405=EDGE_CURVE('',#13535,#13532,#1278,.T.);
#17406=EDGE_CURVE('',#13536,#13534,#1279,.T.);
#17407=EDGE_CURVE('',#13536,#13537,#8545,.T.);
#17408=EDGE_CURVE('',#13537,#13535,#1280,.T.);
#17409=EDGE_CURVE('',#13538,#13536,#1281,.T.);
#17410=EDGE_CURVE('',#13538,#13539,#8546,.T.);
#17411=EDGE_CURVE('',#13539,#13537,#1282,.T.);
#17412=EDGE_CURVE('',#13540,#13538,#1283,.T.);
#17413=EDGE_CURVE('',#13540,#13541,#8547,.T.);
#17414=EDGE_CURVE('',#13541,#13539,#1284,.T.);
#17415=EDGE_CURVE('',#13542,#13540,#1285,.T.);
#17416=EDGE_CURVE('',#13542,#13543,#8548,.T.);
#17417=EDGE_CURVE('',#13543,#13541,#1286,.T.);
#17418=EDGE_CURVE('',#13544,#13542,#1287,.T.);
#17419=EDGE_CURVE('',#13544,#13545,#8549,.T.);
#17420=EDGE_CURVE('',#13545,#13543,#1288,.T.);
#17421=EDGE_CURVE('',#13546,#13544,#1289,.T.);
#17422=EDGE_CURVE('',#13546,#13547,#8550,.T.);
#17423=EDGE_CURVE('',#13547,#13545,#1290,.T.);
#17424=EDGE_CURVE('',#13531,#13546,#1291,.T.);
#17425=EDGE_CURVE('',#13533,#13547,#1292,.T.);
#17426=EDGE_CURVE('',#13548,#13549,#1293,.T.);
#17427=EDGE_CURVE('',#13548,#13550,#8551,.T.);
#17428=EDGE_CURVE('',#13550,#13551,#1294,.T.);
#17429=EDGE_CURVE('',#13549,#13551,#8552,.T.);
#17430=EDGE_CURVE('',#13552,#13548,#1295,.T.);
#17431=EDGE_CURVE('',#13552,#13553,#8553,.T.);
#17432=EDGE_CURVE('',#13553,#13550,#1296,.T.);
#17433=EDGE_CURVE('',#13554,#13552,#1297,.T.);
#17434=EDGE_CURVE('',#13554,#13555,#8554,.T.);
#17435=EDGE_CURVE('',#13555,#13553,#1298,.T.);
#17436=EDGE_CURVE('',#13556,#13554,#1299,.T.);
#17437=EDGE_CURVE('',#13556,#13557,#8555,.T.);
#17438=EDGE_CURVE('',#13557,#13555,#1300,.T.);
#17439=EDGE_CURVE('',#13558,#13556,#1301,.T.);
#17440=EDGE_CURVE('',#13558,#13559,#8556,.T.);
#17441=EDGE_CURVE('',#13559,#13557,#1302,.T.);
#17442=EDGE_CURVE('',#13560,#13558,#1303,.T.);
#17443=EDGE_CURVE('',#13560,#13561,#8557,.T.);
#17444=EDGE_CURVE('',#13561,#13559,#1304,.T.);
#17445=EDGE_CURVE('',#13562,#13560,#1305,.T.);
#17446=EDGE_CURVE('',#13562,#13563,#8558,.T.);
#17447=EDGE_CURVE('',#13563,#13561,#1306,.T.);
#17448=EDGE_CURVE('',#13549,#13562,#1307,.T.);
#17449=EDGE_CURVE('',#13551,#13563,#1308,.T.);
#17450=EDGE_CURVE('',#13564,#13565,#1309,.T.);
#17451=EDGE_CURVE('',#13564,#13566,#8559,.T.);
#17452=EDGE_CURVE('',#13566,#13567,#1310,.T.);
#17453=EDGE_CURVE('',#13565,#13567,#8560,.T.);
#17454=EDGE_CURVE('',#13568,#13564,#1311,.T.);
#17455=EDGE_CURVE('',#13568,#13569,#8561,.T.);
#17456=EDGE_CURVE('',#13569,#13566,#1312,.T.);
#17457=EDGE_CURVE('',#13570,#13568,#1313,.T.);
#17458=EDGE_CURVE('',#13570,#13571,#8562,.T.);
#17459=EDGE_CURVE('',#13571,#13569,#1314,.T.);
#17460=EDGE_CURVE('',#13572,#13570,#1315,.T.);
#17461=EDGE_CURVE('',#13572,#13573,#8563,.T.);
#17462=EDGE_CURVE('',#13573,#13571,#1316,.T.);
#17463=EDGE_CURVE('',#13574,#13572,#1317,.T.);
#17464=EDGE_CURVE('',#13574,#13575,#8564,.T.);
#17465=EDGE_CURVE('',#13575,#13573,#1318,.T.);
#17466=EDGE_CURVE('',#13576,#13574,#1319,.T.);
#17467=EDGE_CURVE('',#13576,#13577,#8565,.T.);
#17468=EDGE_CURVE('',#13577,#13575,#1320,.T.);
#17469=EDGE_CURVE('',#13578,#13576,#1321,.T.);
#17470=EDGE_CURVE('',#13578,#13579,#8566,.T.);
#17471=EDGE_CURVE('',#13579,#13577,#1322,.T.);
#17472=EDGE_CURVE('',#13580,#13578,#1323,.T.);
#17473=EDGE_CURVE('',#13580,#13581,#8567,.T.);
#17474=EDGE_CURVE('',#13581,#13579,#1324,.T.);
#17475=EDGE_CURVE('',#13582,#13580,#1325,.T.);
#17476=EDGE_CURVE('',#13582,#13583,#8568,.T.);
#17477=EDGE_CURVE('',#13583,#13581,#1326,.T.);
#17478=EDGE_CURVE('',#13584,#13582,#1327,.T.);
#17479=EDGE_CURVE('',#13584,#13585,#8569,.T.);
#17480=EDGE_CURVE('',#13585,#13583,#1328,.T.);
#17481=EDGE_CURVE('',#13586,#13584,#1329,.T.);
#17482=EDGE_CURVE('',#13586,#13587,#8570,.T.);
#17483=EDGE_CURVE('',#13587,#13585,#1330,.T.);
#17484=EDGE_CURVE('',#13588,#13586,#1331,.T.);
#17485=EDGE_CURVE('',#13588,#13589,#8571,.T.);
#17486=EDGE_CURVE('',#13589,#13587,#1332,.T.);
#17487=EDGE_CURVE('',#13590,#13588,#1333,.T.);
#17488=EDGE_CURVE('',#13590,#13591,#8572,.T.);
#17489=EDGE_CURVE('',#13591,#13589,#1334,.T.);
#17490=EDGE_CURVE('',#13592,#13590,#1335,.T.);
#17491=EDGE_CURVE('',#13592,#13593,#8573,.T.);
#17492=EDGE_CURVE('',#13593,#13591,#1336,.T.);
#17493=EDGE_CURVE('',#13594,#13592,#1337,.T.);
#17494=EDGE_CURVE('',#13594,#13595,#8574,.T.);
#17495=EDGE_CURVE('',#13595,#13593,#1338,.T.);
#17496=EDGE_CURVE('',#13565,#13594,#1339,.T.);
#17497=EDGE_CURVE('',#13567,#13595,#1340,.T.);
#17498=EDGE_CURVE('',#13338,#13335,#1341,.T.);
#17499=EDGE_CURVE('',#13596,#13335,#2553,.T.);
#17500=EDGE_CURVE('',#13597,#13596,#2554,.T.);
#17501=EDGE_CURVE('',#13597,#13339,#1342,.T.);
#17502=EDGE_CURVE('',#13334,#13597,#1343,.T.);
#17503=EDGE_CURVE('',#13598,#13216,#1344,.T.);
#17504=EDGE_CURVE('',#13598,#13455,#1345,.T.);
#17505=EDGE_CURVE('',#13216,#13599,#2555,.T.);
#17506=EDGE_CURVE('',#13599,#13215,#2556,.T.);
#17507=EDGE_CURVE('',#13215,#13600,#1346,.T.);
#17508=EDGE_CURVE('',#13600,#13598,#2557,.T.);
#17509=EDGE_CURVE('',#13600,#13454,#1347,.T.);
#17510=EDGE_CURVE('',#13601,#13601,#2558,.T.);
#17511=EDGE_CURVE('',#13601,#13596,#2559,.T.);
#17512=EDGE_CURVE('',#13333,#13597,#2560,.T.);
#17513=EDGE_CURVE('',#13602,#13603,#8575,.T.);
#17514=EDGE_CURVE('',#13604,#13602,#8576,.T.);
#17515=EDGE_CURVE('',#13605,#13604,#8577,.T.);
#17516=EDGE_CURVE('',#13606,#13605,#8578,.T.);
#17517=EDGE_CURVE('',#13607,#13606,#8579,.T.);
#17518=EDGE_CURVE('',#13603,#13607,#8580,.T.);
#17519=EDGE_CURVE('',#13608,#13609,#355,.T.);
#17520=EDGE_CURVE('',#13610,#13608,#356,.T.);
#17521=EDGE_CURVE('',#13611,#13610,#357,.T.);
#17522=EDGE_CURVE('',#13612,#13611,#358,.T.);
#17523=EDGE_CURVE('',#13613,#13612,#359,.T.);
#17524=EDGE_CURVE('',#13613,#13614,#8581,.T.);
#17525=EDGE_CURVE('',#13614,#13614,#2561,.T.);
#17526=EDGE_CURVE('',#13615,#13613,#360,.T.);
#17527=EDGE_CURVE('',#13609,#13615,#361,.T.);
#17528=EDGE_CURVE('',#13607,#13611,#8582,.T.);
#17529=EDGE_CURVE('',#13606,#13612,#8583,.T.);
#17530=EDGE_CURVE('',#13603,#13610,#8584,.T.);
#17531=EDGE_CURVE('',#13602,#13608,#8585,.T.);
#17532=EDGE_CURVE('',#13604,#13609,#8586,.T.);
#17533=EDGE_CURVE('',#13605,#13615,#8587,.T.);
#17534=EDGE_CURVE('',#13616,#13616,#2562,.T.);
#17535=EDGE_CURVE('',#13599,#13616,#8588,.T.);
#24089=ORIENTED_EDGE('',*,*,#16928,.F.);
#24090=ORIENTED_EDGE('',*,*,#16929,.T.);
#24091=ORIENTED_EDGE('',*,*,#16930,.T.);
#24092=ORIENTED_EDGE('',*,*,#16931,.T.);
#24093=ORIENTED_EDGE('',*,*,#16932,.F.);
#24094=ORIENTED_EDGE('',*,*,#16933,.T.);
#24095=ORIENTED_EDGE('',*,*,#16928,.T.);
#24096=ORIENTED_EDGE('',*,*,#16934,.T.);
#24097=ORIENTED_EDGE('',*,*,#16935,.F.);
#24098=ORIENTED_EDGE('',*,*,#16936,.T.);
#24099=ORIENTED_EDGE('',*,*,#16932,.T.);
#24100=ORIENTED_EDGE('',*,*,#16937,.T.);
#24101=ORIENTED_EDGE('',*,*,#16938,.F.);
#24102=ORIENTED_EDGE('',*,*,#16939,.T.);
#24103=ORIENTED_EDGE('',*,*,#16935,.T.);
#24104=ORIENTED_EDGE('',*,*,#16940,.T.);
#24105=ORIENTED_EDGE('',*,*,#16941,.F.);
#24106=ORIENTED_EDGE('',*,*,#16942,.T.);
#24107=ORIENTED_EDGE('',*,*,#16938,.T.);
#24108=ORIENTED_EDGE('',*,*,#16943,.T.);
#24109=ORIENTED_EDGE('',*,*,#16944,.F.);
#24110=ORIENTED_EDGE('',*,*,#16945,.T.);
#24111=ORIENTED_EDGE('',*,*,#16941,.T.);
#24112=ORIENTED_EDGE('',*,*,#16946,.T.);
#24113=ORIENTED_EDGE('',*,*,#16947,.F.);
#24114=ORIENTED_EDGE('',*,*,#16948,.T.);
#24115=ORIENTED_EDGE('',*,*,#16944,.T.);
#24116=ORIENTED_EDGE('',*,*,#16949,.T.);
#24117=ORIENTED_EDGE('',*,*,#16950,.F.);
#24118=ORIENTED_EDGE('',*,*,#16951,.T.);
#24119=ORIENTED_EDGE('',*,*,#16947,.T.);
#24120=ORIENTED_EDGE('',*,*,#16952,.T.);
#24121=ORIENTED_EDGE('',*,*,#16953,.F.);
#24122=ORIENTED_EDGE('',*,*,#16954,.T.);
#24123=ORIENTED_EDGE('',*,*,#16950,.T.);
#24124=ORIENTED_EDGE('',*,*,#16955,.T.);
#24125=ORIENTED_EDGE('',*,*,#16956,.F.);
#24126=ORIENTED_EDGE('',*,*,#16957,.T.);
#24127=ORIENTED_EDGE('',*,*,#16953,.T.);
#24128=ORIENTED_EDGE('',*,*,#16958,.T.);
#24129=ORIENTED_EDGE('',*,*,#16959,.F.);
#24130=ORIENTED_EDGE('',*,*,#16960,.T.);
#24131=ORIENTED_EDGE('',*,*,#16956,.T.);
#24132=ORIENTED_EDGE('',*,*,#16961,.T.);
#24133=ORIENTED_EDGE('',*,*,#16962,.F.);
#24134=ORIENTED_EDGE('',*,*,#16963,.T.);
#24135=ORIENTED_EDGE('',*,*,#16959,.T.);
#24136=ORIENTED_EDGE('',*,*,#16964,.T.);
#24137=ORIENTED_EDGE('',*,*,#16965,.F.);
#24138=ORIENTED_EDGE('',*,*,#16966,.T.);
#24139=ORIENTED_EDGE('',*,*,#16962,.T.);
#24140=ORIENTED_EDGE('',*,*,#16967,.T.);
#24141=ORIENTED_EDGE('',*,*,#16968,.F.);
#24142=ORIENTED_EDGE('',*,*,#16969,.T.);
#24143=ORIENTED_EDGE('',*,*,#16965,.T.);
#24144=ORIENTED_EDGE('',*,*,#16970,.T.);
#24145=ORIENTED_EDGE('',*,*,#16971,.F.);
#24146=ORIENTED_EDGE('',*,*,#16972,.T.);
#24147=ORIENTED_EDGE('',*,*,#16968,.T.);
#24148=ORIENTED_EDGE('',*,*,#16973,.T.);
#24149=ORIENTED_EDGE('',*,*,#16974,.F.);
#24150=ORIENTED_EDGE('',*,*,#16975,.T.);
#24151=ORIENTED_EDGE('',*,*,#16971,.T.);
#24152=ORIENTED_EDGE('',*,*,#16976,.T.);
#24153=ORIENTED_EDGE('',*,*,#16977,.F.);
#24154=ORIENTED_EDGE('',*,*,#16978,.T.);
#24155=ORIENTED_EDGE('',*,*,#16974,.T.);
#24156=ORIENTED_EDGE('',*,*,#16979,.T.);
#24157=ORIENTED_EDGE('',*,*,#16980,.F.);
#24158=ORIENTED_EDGE('',*,*,#16981,.T.);
#24159=ORIENTED_EDGE('',*,*,#16977,.T.);
#24160=ORIENTED_EDGE('',*,*,#16982,.T.);
#24161=ORIENTED_EDGE('',*,*,#16983,.F.);
#24162=ORIENTED_EDGE('',*,*,#16984,.T.);
#24163=ORIENTED_EDGE('',*,*,#16980,.T.);
#24164=ORIENTED_EDGE('',*,*,#16985,.T.);
#24165=ORIENTED_EDGE('',*,*,#16986,.F.);
#24166=ORIENTED_EDGE('',*,*,#16987,.T.);
#24167=ORIENTED_EDGE('',*,*,#16983,.T.);
#24168=ORIENTED_EDGE('',*,*,#16988,.T.);
#24169=ORIENTED_EDGE('',*,*,#16989,.F.);
#24170=ORIENTED_EDGE('',*,*,#16990,.T.);
#24171=ORIENTED_EDGE('',*,*,#16986,.T.);
#24172=ORIENTED_EDGE('',*,*,#16991,.T.);
#24173=ORIENTED_EDGE('',*,*,#16992,.F.);
#24174=ORIENTED_EDGE('',*,*,#16993,.T.);
#24175=ORIENTED_EDGE('',*,*,#16989,.T.);
#24176=ORIENTED_EDGE('',*,*,#16994,.T.);
#24177=ORIENTED_EDGE('',*,*,#16995,.F.);
#24178=ORIENTED_EDGE('',*,*,#16996,.T.);
#24179=ORIENTED_EDGE('',*,*,#16992,.T.);
#24180=ORIENTED_EDGE('',*,*,#16997,.T.);
#24181=ORIENTED_EDGE('',*,*,#16998,.F.);
#24182=ORIENTED_EDGE('',*,*,#16999,.T.);
#24183=ORIENTED_EDGE('',*,*,#16995,.T.);
#24184=ORIENTED_EDGE('',*,*,#17000,.T.);
#24185=ORIENTED_EDGE('',*,*,#17001,.F.);
#24186=ORIENTED_EDGE('',*,*,#17002,.T.);
#24187=ORIENTED_EDGE('',*,*,#16998,.T.);
#24188=ORIENTED_EDGE('',*,*,#17003,.T.);
#24189=ORIENTED_EDGE('',*,*,#17004,.F.);
#24190=ORIENTED_EDGE('',*,*,#17005,.T.);
#24191=ORIENTED_EDGE('',*,*,#17001,.T.);
#24192=ORIENTED_EDGE('',*,*,#17006,.T.);
#24193=ORIENTED_EDGE('',*,*,#17007,.F.);
#24194=ORIENTED_EDGE('',*,*,#17008,.T.);
#24195=ORIENTED_EDGE('',*,*,#17004,.T.);
#24196=ORIENTED_EDGE('',*,*,#17009,.T.);
#24197=ORIENTED_EDGE('',*,*,#17010,.F.);
#24198=ORIENTED_EDGE('',*,*,#17011,.T.);
#24199=ORIENTED_EDGE('',*,*,#17007,.T.);
#24200=ORIENTED_EDGE('',*,*,#17012,.T.);
#24201=ORIENTED_EDGE('',*,*,#17013,.F.);
#24202=ORIENTED_EDGE('',*,*,#17014,.T.);
#24203=ORIENTED_EDGE('',*,*,#17010,.T.);
#24204=ORIENTED_EDGE('',*,*,#17015,.T.);
#24205=ORIENTED_EDGE('',*,*,#17016,.F.);
#24206=ORIENTED_EDGE('',*,*,#17017,.T.);
#24207=ORIENTED_EDGE('',*,*,#17013,.T.);
#24208=ORIENTED_EDGE('',*,*,#17018,.T.);
#24209=ORIENTED_EDGE('',*,*,#17019,.F.);
#24210=ORIENTED_EDGE('',*,*,#17020,.T.);
#24211=ORIENTED_EDGE('',*,*,#17016,.T.);
#24212=ORIENTED_EDGE('',*,*,#17021,.T.);
#24213=ORIENTED_EDGE('',*,*,#17022,.F.);
#24214=ORIENTED_EDGE('',*,*,#17023,.T.);
#24215=ORIENTED_EDGE('',*,*,#17019,.T.);
#24216=ORIENTED_EDGE('',*,*,#17024,.T.);
#24217=ORIENTED_EDGE('',*,*,#17025,.F.);
#24218=ORIENTED_EDGE('',*,*,#17026,.T.);
#24219=ORIENTED_EDGE('',*,*,#17022,.T.);
#24220=ORIENTED_EDGE('',*,*,#17027,.T.);
#24221=ORIENTED_EDGE('',*,*,#17028,.F.);
#24222=ORIENTED_EDGE('',*,*,#17029,.T.);
#24223=ORIENTED_EDGE('',*,*,#17025,.T.);
#24224=ORIENTED_EDGE('',*,*,#17030,.T.);
#24225=ORIENTED_EDGE('',*,*,#17031,.F.);
#24226=ORIENTED_EDGE('',*,*,#17032,.T.);
#24227=ORIENTED_EDGE('',*,*,#17028,.T.);
#24228=ORIENTED_EDGE('',*,*,#17033,.T.);
#24229=ORIENTED_EDGE('',*,*,#17034,.F.);
#24230=ORIENTED_EDGE('',*,*,#17035,.T.);
#24231=ORIENTED_EDGE('',*,*,#17031,.T.);
#24232=ORIENTED_EDGE('',*,*,#17036,.T.);
#24233=ORIENTED_EDGE('',*,*,#17037,.F.);
#24234=ORIENTED_EDGE('',*,*,#17038,.T.);
#24235=ORIENTED_EDGE('',*,*,#17034,.T.);
#24236=ORIENTED_EDGE('',*,*,#17039,.T.);
#24237=ORIENTED_EDGE('',*,*,#17040,.F.);
#24238=ORIENTED_EDGE('',*,*,#17041,.T.);
#24239=ORIENTED_EDGE('',*,*,#17037,.T.);
#24240=ORIENTED_EDGE('',*,*,#17042,.T.);
#24241=ORIENTED_EDGE('',*,*,#17043,.F.);
#24242=ORIENTED_EDGE('',*,*,#17044,.T.);
#24243=ORIENTED_EDGE('',*,*,#17040,.T.);
#24244=ORIENTED_EDGE('',*,*,#17045,.T.);
#24245=ORIENTED_EDGE('',*,*,#17046,.F.);
#24246=ORIENTED_EDGE('',*,*,#17047,.T.);
#24247=ORIENTED_EDGE('',*,*,#17043,.T.);
#24248=ORIENTED_EDGE('',*,*,#17048,.T.);
#24249=ORIENTED_EDGE('',*,*,#17049,.F.);
#24250=ORIENTED_EDGE('',*,*,#17050,.T.);
#24251=ORIENTED_EDGE('',*,*,#17046,.T.);
#24252=ORIENTED_EDGE('',*,*,#17051,.T.);
#24253=ORIENTED_EDGE('',*,*,#17052,.F.);
#24254=ORIENTED_EDGE('',*,*,#17053,.T.);
#24255=ORIENTED_EDGE('',*,*,#17049,.T.);
#24256=ORIENTED_EDGE('',*,*,#17054,.T.);
#24257=ORIENTED_EDGE('',*,*,#17055,.F.);
#24258=ORIENTED_EDGE('',*,*,#17056,.T.);
#24259=ORIENTED_EDGE('',*,*,#17052,.T.);
#24260=ORIENTED_EDGE('',*,*,#17057,.T.);
#24261=ORIENTED_EDGE('',*,*,#17058,.F.);
#24262=ORIENTED_EDGE('',*,*,#17059,.T.);
#24263=ORIENTED_EDGE('',*,*,#17055,.T.);
#24264=ORIENTED_EDGE('',*,*,#17060,.T.);
#24265=ORIENTED_EDGE('',*,*,#17061,.F.);
#24266=ORIENTED_EDGE('',*,*,#17062,.T.);
#24267=ORIENTED_EDGE('',*,*,#17058,.T.);
#24268=ORIENTED_EDGE('',*,*,#17063,.T.);
#24269=ORIENTED_EDGE('',*,*,#17064,.F.);
#24270=ORIENTED_EDGE('',*,*,#17065,.T.);
#24271=ORIENTED_EDGE('',*,*,#17061,.T.);
#24272=ORIENTED_EDGE('',*,*,#17066,.T.);
#24273=ORIENTED_EDGE('',*,*,#17067,.F.);
#24274=ORIENTED_EDGE('',*,*,#17068,.T.);
#24275=ORIENTED_EDGE('',*,*,#17064,.T.);
#24276=ORIENTED_EDGE('',*,*,#17069,.T.);
#24277=ORIENTED_EDGE('',*,*,#17070,.F.);
#24278=ORIENTED_EDGE('',*,*,#17071,.T.);
#24279=ORIENTED_EDGE('',*,*,#17067,.T.);
#24280=ORIENTED_EDGE('',*,*,#17072,.T.);
#24281=ORIENTED_EDGE('',*,*,#17073,.F.);
#24282=ORIENTED_EDGE('',*,*,#17074,.T.);
#24283=ORIENTED_EDGE('',*,*,#17070,.T.);
#24284=ORIENTED_EDGE('',*,*,#17075,.T.);
#24285=ORIENTED_EDGE('',*,*,#17076,.F.);
#24286=ORIENTED_EDGE('',*,*,#17077,.T.);
#24287=ORIENTED_EDGE('',*,*,#17073,.T.);
#24288=ORIENTED_EDGE('',*,*,#17078,.T.);
#24289=ORIENTED_EDGE('',*,*,#17079,.F.);
#24290=ORIENTED_EDGE('',*,*,#17080,.T.);
#24291=ORIENTED_EDGE('',*,*,#17076,.T.);
#24292=ORIENTED_EDGE('',*,*,#17081,.T.);
#24293=ORIENTED_EDGE('',*,*,#17082,.F.);
#24294=ORIENTED_EDGE('',*,*,#17083,.T.);
#24295=ORIENTED_EDGE('',*,*,#17079,.T.);
#24296=ORIENTED_EDGE('',*,*,#17084,.T.);
#24297=ORIENTED_EDGE('',*,*,#17085,.F.);
#24298=ORIENTED_EDGE('',*,*,#17086,.T.);
#24299=ORIENTED_EDGE('',*,*,#17082,.T.);
#24300=ORIENTED_EDGE('',*,*,#17087,.T.);
#24301=ORIENTED_EDGE('',*,*,#17088,.F.);
#24302=ORIENTED_EDGE('',*,*,#17089,.T.);
#24303=ORIENTED_EDGE('',*,*,#17085,.T.);
#24304=ORIENTED_EDGE('',*,*,#17090,.T.);
#24305=ORIENTED_EDGE('',*,*,#17091,.F.);
#24306=ORIENTED_EDGE('',*,*,#17092,.T.);
#24307=ORIENTED_EDGE('',*,*,#17088,.T.);
#24308=ORIENTED_EDGE('',*,*,#17093,.T.);
#24309=ORIENTED_EDGE('',*,*,#17094,.F.);
#24310=ORIENTED_EDGE('',*,*,#17095,.T.);
#24311=ORIENTED_EDGE('',*,*,#17091,.T.);
#24312=ORIENTED_EDGE('',*,*,#17096,.T.);
#24313=ORIENTED_EDGE('',*,*,#17097,.F.);
#24314=ORIENTED_EDGE('',*,*,#17098,.T.);
#24315=ORIENTED_EDGE('',*,*,#17094,.T.);
#24316=ORIENTED_EDGE('',*,*,#17099,.T.);
#24317=ORIENTED_EDGE('',*,*,#17100,.F.);
#24318=ORIENTED_EDGE('',*,*,#17101,.T.);
#24319=ORIENTED_EDGE('',*,*,#17097,.T.);
#24320=ORIENTED_EDGE('',*,*,#17102,.T.);
#24321=ORIENTED_EDGE('',*,*,#17103,.F.);
#24322=ORIENTED_EDGE('',*,*,#17104,.T.);
#24323=ORIENTED_EDGE('',*,*,#17100,.T.);
#24324=ORIENTED_EDGE('',*,*,#17105,.T.);
#24325=ORIENTED_EDGE('',*,*,#17106,.F.);
#24326=ORIENTED_EDGE('',*,*,#17107,.F.);
#24327=ORIENTED_EDGE('',*,*,#17108,.T.);
#24328=ORIENTED_EDGE('',*,*,#17103,.T.);
#24329=ORIENTED_EDGE('',*,*,#17109,.T.);
#24330=ORIENTED_EDGE('',*,*,#17110,.F.);
#24331=ORIENTED_EDGE('',*,*,#17111,.T.);
#24332=ORIENTED_EDGE('',*,*,#17112,.F.);
#24333=ORIENTED_EDGE('',*,*,#17113,.F.);
#24334=ORIENTED_EDGE('',*,*,#17114,.F.);
#24335=ORIENTED_EDGE('',*,*,#17115,.T.);
#24336=ORIENTED_EDGE('',*,*,#17110,.T.);
#24337=ORIENTED_EDGE('',*,*,#17116,.F.);
#24338=ORIENTED_EDGE('',*,*,#17117,.F.);
#24339=ORIENTED_EDGE('',*,*,#17118,.T.);
#24340=ORIENTED_EDGE('',*,*,#17114,.T.);
#24341=ORIENTED_EDGE('',*,*,#17119,.F.);
#24342=ORIENTED_EDGE('',*,*,#17120,.F.);
#24343=ORIENTED_EDGE('',*,*,#17121,.T.);
#24344=ORIENTED_EDGE('',*,*,#17117,.T.);
#24345=ORIENTED_EDGE('',*,*,#17122,.F.);
#24346=ORIENTED_EDGE('',*,*,#17123,.F.);
#24347=ORIENTED_EDGE('',*,*,#17124,.T.);
#24348=ORIENTED_EDGE('',*,*,#17120,.T.);
#24349=ORIENTED_EDGE('',*,*,#17125,.F.);
#24350=ORIENTED_EDGE('',*,*,#17126,.F.);
#24351=ORIENTED_EDGE('',*,*,#17127,.T.);
#24352=ORIENTED_EDGE('',*,*,#17123,.T.);
#24353=ORIENTED_EDGE('',*,*,#17128,.F.);
#24354=ORIENTED_EDGE('',*,*,#17129,.F.);
#24355=ORIENTED_EDGE('',*,*,#17130,.T.);
#24356=ORIENTED_EDGE('',*,*,#17126,.T.);
#24357=ORIENTED_EDGE('',*,*,#17131,.F.);
#24358=ORIENTED_EDGE('',*,*,#17132,.F.);
#24359=ORIENTED_EDGE('',*,*,#17133,.T.);
#24360=ORIENTED_EDGE('',*,*,#17129,.T.);
#24361=ORIENTED_EDGE('',*,*,#17134,.F.);
#24362=ORIENTED_EDGE('',*,*,#17135,.F.);
#24363=ORIENTED_EDGE('',*,*,#17136,.T.);
#24364=ORIENTED_EDGE('',*,*,#17132,.T.);
#24365=ORIENTED_EDGE('',*,*,#17137,.F.);
#24366=ORIENTED_EDGE('',*,*,#17138,.F.);
#24367=ORIENTED_EDGE('',*,*,#17139,.T.);
#24368=ORIENTED_EDGE('',*,*,#17135,.T.);
#24369=ORIENTED_EDGE('',*,*,#17140,.F.);
#24370=ORIENTED_EDGE('',*,*,#17141,.F.);
#24371=ORIENTED_EDGE('',*,*,#17142,.T.);
#24372=ORIENTED_EDGE('',*,*,#17138,.T.);
#24373=ORIENTED_EDGE('',*,*,#17143,.F.);
#24374=ORIENTED_EDGE('',*,*,#17144,.F.);
#24375=ORIENTED_EDGE('',*,*,#17145,.T.);
#24376=ORIENTED_EDGE('',*,*,#17141,.T.);
#24377=ORIENTED_EDGE('',*,*,#17146,.F.);
#24378=ORIENTED_EDGE('',*,*,#17147,.F.);
#24379=ORIENTED_EDGE('',*,*,#17148,.T.);
#24380=ORIENTED_EDGE('',*,*,#17144,.T.);
#24381=ORIENTED_EDGE('',*,*,#17149,.F.);
#24382=ORIENTED_EDGE('',*,*,#17150,.F.);
#24383=ORIENTED_EDGE('',*,*,#17151,.T.);
#24384=ORIENTED_EDGE('',*,*,#17147,.T.);
#24385=ORIENTED_EDGE('',*,*,#17152,.F.);
#24386=ORIENTED_EDGE('',*,*,#17153,.F.);
#24387=ORIENTED_EDGE('',*,*,#17154,.T.);
#24388=ORIENTED_EDGE('',*,*,#17150,.T.);
#24389=ORIENTED_EDGE('',*,*,#17155,.F.);
#24390=ORIENTED_EDGE('',*,*,#17156,.F.);
#24391=ORIENTED_EDGE('',*,*,#17157,.T.);
#24392=ORIENTED_EDGE('',*,*,#17153,.T.);
#24393=ORIENTED_EDGE('',*,*,#17158,.F.);
#24394=ORIENTED_EDGE('',*,*,#17159,.F.);
#24395=ORIENTED_EDGE('',*,*,#17160,.T.);
#24396=ORIENTED_EDGE('',*,*,#17156,.T.);
#24397=ORIENTED_EDGE('',*,*,#17161,.F.);
#24398=ORIENTED_EDGE('',*,*,#17162,.F.);
#24399=ORIENTED_EDGE('',*,*,#17163,.T.);
#24400=ORIENTED_EDGE('',*,*,#17159,.T.);
#24401=ORIENTED_EDGE('',*,*,#17164,.F.);
#24402=ORIENTED_EDGE('',*,*,#17165,.F.);
#24403=ORIENTED_EDGE('',*,*,#17166,.T.);
#24404=ORIENTED_EDGE('',*,*,#17162,.T.);
#24405=ORIENTED_EDGE('',*,*,#17167,.F.);
#24406=ORIENTED_EDGE('',*,*,#17168,.F.);
#24407=ORIENTED_EDGE('',*,*,#17169,.T.);
#24408=ORIENTED_EDGE('',*,*,#17165,.T.);
#24409=ORIENTED_EDGE('',*,*,#17170,.F.);
#24410=ORIENTED_EDGE('',*,*,#17171,.F.);
#24411=ORIENTED_EDGE('',*,*,#17172,.T.);
#24412=ORIENTED_EDGE('',*,*,#17168,.T.);
#24413=ORIENTED_EDGE('',*,*,#17173,.F.);
#24414=ORIENTED_EDGE('',*,*,#17174,.F.);
#24415=ORIENTED_EDGE('',*,*,#17175,.T.);
#24416=ORIENTED_EDGE('',*,*,#17171,.T.);
#24417=ORIENTED_EDGE('',*,*,#17176,.F.);
#24418=ORIENTED_EDGE('',*,*,#17177,.F.);
#24419=ORIENTED_EDGE('',*,*,#17178,.T.);
#24420=ORIENTED_EDGE('',*,*,#17174,.T.);
#24421=ORIENTED_EDGE('',*,*,#17179,.F.);
#24422=ORIENTED_EDGE('',*,*,#17180,.F.);
#24423=ORIENTED_EDGE('',*,*,#17181,.T.);
#24424=ORIENTED_EDGE('',*,*,#17177,.T.);
#24425=ORIENTED_EDGE('',*,*,#17182,.F.);
#24426=ORIENTED_EDGE('',*,*,#17183,.F.);
#24427=ORIENTED_EDGE('',*,*,#17184,.T.);
#24428=ORIENTED_EDGE('',*,*,#17180,.T.);
#24429=ORIENTED_EDGE('',*,*,#17185,.F.);
#24430=ORIENTED_EDGE('',*,*,#17186,.F.);
#24431=ORIENTED_EDGE('',*,*,#17187,.T.);
#24432=ORIENTED_EDGE('',*,*,#17183,.T.);
#24433=ORIENTED_EDGE('',*,*,#17188,.F.);
#24434=ORIENTED_EDGE('',*,*,#17189,.F.);
#24435=ORIENTED_EDGE('',*,*,#17190,.T.);
#24436=ORIENTED_EDGE('',*,*,#17186,.T.);
#24437=ORIENTED_EDGE('',*,*,#17191,.F.);
#24438=ORIENTED_EDGE('',*,*,#17192,.F.);
#24439=ORIENTED_EDGE('',*,*,#17193,.T.);
#24440=ORIENTED_EDGE('',*,*,#17189,.T.);
#24441=ORIENTED_EDGE('',*,*,#17194,.F.);
#24442=ORIENTED_EDGE('',*,*,#17195,.F.);
#24443=ORIENTED_EDGE('',*,*,#17196,.T.);
#24444=ORIENTED_EDGE('',*,*,#17192,.T.);
#24445=ORIENTED_EDGE('',*,*,#17197,.F.);
#24446=ORIENTED_EDGE('',*,*,#17198,.F.);
#24447=ORIENTED_EDGE('',*,*,#17199,.T.);
#24448=ORIENTED_EDGE('',*,*,#17195,.T.);
#24449=ORIENTED_EDGE('',*,*,#17200,.F.);
#24450=ORIENTED_EDGE('',*,*,#17201,.F.);
#24451=ORIENTED_EDGE('',*,*,#17202,.T.);
#24452=ORIENTED_EDGE('',*,*,#17198,.T.);
#24453=ORIENTED_EDGE('',*,*,#17203,.F.);
#24454=ORIENTED_EDGE('',*,*,#17204,.F.);
#24455=ORIENTED_EDGE('',*,*,#17205,.T.);
#24456=ORIENTED_EDGE('',*,*,#17201,.T.);
#24457=ORIENTED_EDGE('',*,*,#17206,.F.);
#24458=ORIENTED_EDGE('',*,*,#17207,.F.);
#24459=ORIENTED_EDGE('',*,*,#17208,.T.);
#24460=ORIENTED_EDGE('',*,*,#17204,.T.);
#24461=ORIENTED_EDGE('',*,*,#17209,.F.);
#24462=ORIENTED_EDGE('',*,*,#17210,.F.);
#24463=ORIENTED_EDGE('',*,*,#17211,.T.);
#24464=ORIENTED_EDGE('',*,*,#17207,.T.);
#24465=ORIENTED_EDGE('',*,*,#17212,.F.);
#24466=ORIENTED_EDGE('',*,*,#17213,.F.);
#24467=ORIENTED_EDGE('',*,*,#17214,.T.);
#24468=ORIENTED_EDGE('',*,*,#17210,.T.);
#24469=ORIENTED_EDGE('',*,*,#17215,.F.);
#24470=ORIENTED_EDGE('',*,*,#17216,.F.);
#24471=ORIENTED_EDGE('',*,*,#17217,.T.);
#24472=ORIENTED_EDGE('',*,*,#17213,.T.);
#24473=ORIENTED_EDGE('',*,*,#17218,.F.);
#24474=ORIENTED_EDGE('',*,*,#17219,.F.);
#24475=ORIENTED_EDGE('',*,*,#17220,.T.);
#24476=ORIENTED_EDGE('',*,*,#17216,.T.);
#24477=ORIENTED_EDGE('',*,*,#17221,.F.);
#24478=ORIENTED_EDGE('',*,*,#17222,.F.);
#24479=ORIENTED_EDGE('',*,*,#17223,.T.);
#24480=ORIENTED_EDGE('',*,*,#17219,.T.);
#24481=ORIENTED_EDGE('',*,*,#17224,.F.);
#24482=ORIENTED_EDGE('',*,*,#17225,.F.);
#24483=ORIENTED_EDGE('',*,*,#17226,.T.);
#24484=ORIENTED_EDGE('',*,*,#17222,.T.);
#24485=ORIENTED_EDGE('',*,*,#17227,.F.);
#24486=ORIENTED_EDGE('',*,*,#17228,.F.);
#24487=ORIENTED_EDGE('',*,*,#17229,.T.);
#24488=ORIENTED_EDGE('',*,*,#17225,.T.);
#24489=ORIENTED_EDGE('',*,*,#17230,.F.);
#24490=ORIENTED_EDGE('',*,*,#17231,.F.);
#24491=ORIENTED_EDGE('',*,*,#17232,.T.);
#24492=ORIENTED_EDGE('',*,*,#17228,.T.);
#24493=ORIENTED_EDGE('',*,*,#17233,.F.);
#24494=ORIENTED_EDGE('',*,*,#17234,.F.);
#24495=ORIENTED_EDGE('',*,*,#17235,.T.);
#24496=ORIENTED_EDGE('',*,*,#17231,.T.);
#24497=ORIENTED_EDGE('',*,*,#17236,.F.);
#24498=ORIENTED_EDGE('',*,*,#17237,.F.);
#24499=ORIENTED_EDGE('',*,*,#17238,.T.);
#24500=ORIENTED_EDGE('',*,*,#17234,.T.);
#24501=ORIENTED_EDGE('',*,*,#17239,.F.);
#24502=ORIENTED_EDGE('',*,*,#17240,.F.);
#24503=ORIENTED_EDGE('',*,*,#17241,.T.);
#24504=ORIENTED_EDGE('',*,*,#17237,.T.);
#24505=ORIENTED_EDGE('',*,*,#17242,.F.);
#24506=ORIENTED_EDGE('',*,*,#17243,.F.);
#24507=ORIENTED_EDGE('',*,*,#17244,.T.);
#24508=ORIENTED_EDGE('',*,*,#17240,.T.);
#24509=ORIENTED_EDGE('',*,*,#17245,.F.);
#24510=ORIENTED_EDGE('',*,*,#17246,.F.);
#24511=ORIENTED_EDGE('',*,*,#17247,.T.);
#24512=ORIENTED_EDGE('',*,*,#17243,.T.);
#24513=ORIENTED_EDGE('',*,*,#17248,.F.);
#24514=ORIENTED_EDGE('',*,*,#17249,.F.);
#24515=ORIENTED_EDGE('',*,*,#17250,.T.);
#24516=ORIENTED_EDGE('',*,*,#17246,.T.);
#24517=ORIENTED_EDGE('',*,*,#17251,.F.);
#24518=ORIENTED_EDGE('',*,*,#17252,.F.);
#24519=ORIENTED_EDGE('',*,*,#17253,.T.);
#24520=ORIENTED_EDGE('',*,*,#17249,.T.);
#24521=ORIENTED_EDGE('',*,*,#17254,.F.);
#24522=ORIENTED_EDGE('',*,*,#17255,.F.);
#24523=ORIENTED_EDGE('',*,*,#17256,.T.);
#24524=ORIENTED_EDGE('',*,*,#17252,.T.);
#24525=ORIENTED_EDGE('',*,*,#17257,.F.);
#24526=ORIENTED_EDGE('',*,*,#17258,.F.);
#24527=ORIENTED_EDGE('',*,*,#17259,.T.);
#24528=ORIENTED_EDGE('',*,*,#17255,.T.);
#24529=ORIENTED_EDGE('',*,*,#17260,.F.);
#24530=ORIENTED_EDGE('',*,*,#17261,.F.);
#24531=ORIENTED_EDGE('',*,*,#17262,.T.);
#24532=ORIENTED_EDGE('',*,*,#17258,.T.);
#24533=ORIENTED_EDGE('',*,*,#17263,.F.);
#24534=ORIENTED_EDGE('',*,*,#17264,.F.);
#24535=ORIENTED_EDGE('',*,*,#17265,.T.);
#24536=ORIENTED_EDGE('',*,*,#17261,.T.);
#24537=ORIENTED_EDGE('',*,*,#17266,.F.);
#24538=ORIENTED_EDGE('',*,*,#17267,.F.);
#24539=ORIENTED_EDGE('',*,*,#17268,.T.);
#24540=ORIENTED_EDGE('',*,*,#17264,.T.);
#24541=ORIENTED_EDGE('',*,*,#17269,.F.);
#24542=ORIENTED_EDGE('',*,*,#17270,.F.);
#24543=ORIENTED_EDGE('',*,*,#17271,.T.);
#24544=ORIENTED_EDGE('',*,*,#17267,.T.);
#24545=ORIENTED_EDGE('',*,*,#17272,.F.);
#24546=ORIENTED_EDGE('',*,*,#17273,.F.);
#24547=ORIENTED_EDGE('',*,*,#17274,.T.);
#24548=ORIENTED_EDGE('',*,*,#17270,.T.);
#24549=ORIENTED_EDGE('',*,*,#17275,.F.);
#24550=ORIENTED_EDGE('',*,*,#17276,.F.);
#24551=ORIENTED_EDGE('',*,*,#17277,.T.);
#24552=ORIENTED_EDGE('',*,*,#17273,.T.);
#24553=ORIENTED_EDGE('',*,*,#17278,.F.);
#24554=ORIENTED_EDGE('',*,*,#17279,.F.);
#24555=ORIENTED_EDGE('',*,*,#17280,.T.);
#24556=ORIENTED_EDGE('',*,*,#17276,.T.);
#24557=ORIENTED_EDGE('',*,*,#17281,.F.);
#24558=ORIENTED_EDGE('',*,*,#17282,.F.);
#24559=ORIENTED_EDGE('',*,*,#17283,.T.);
#24560=ORIENTED_EDGE('',*,*,#17279,.T.);
#24561=ORIENTED_EDGE('',*,*,#17284,.F.);
#24562=ORIENTED_EDGE('',*,*,#17285,.F.);
#24563=ORIENTED_EDGE('',*,*,#17286,.T.);
#24564=ORIENTED_EDGE('',*,*,#17282,.T.);
#24565=ORIENTED_EDGE('',*,*,#17287,.F.);
#24566=ORIENTED_EDGE('',*,*,#17288,.F.);
#24567=ORIENTED_EDGE('',*,*,#17289,.T.);
#24568=ORIENTED_EDGE('',*,*,#17290,.T.);
#24569=ORIENTED_EDGE('',*,*,#17291,.F.);
#24570=ORIENTED_EDGE('',*,*,#17292,.F.);
#24571=ORIENTED_EDGE('',*,*,#17293,.T.);
#24572=ORIENTED_EDGE('',*,*,#17294,.T.);
#24573=ORIENTED_EDGE('',*,*,#17289,.F.);
#24574=ORIENTED_EDGE('',*,*,#17295,.F.);
#24575=ORIENTED_EDGE('',*,*,#17296,.T.);
#24576=ORIENTED_EDGE('',*,*,#17297,.T.);
#24577=ORIENTED_EDGE('',*,*,#17293,.F.);
#24578=ORIENTED_EDGE('',*,*,#17298,.F.);
#24579=ORIENTED_EDGE('',*,*,#17299,.T.);
#24580=ORIENTED_EDGE('',*,*,#17300,.T.);
#24581=ORIENTED_EDGE('',*,*,#17296,.F.);
#24582=ORIENTED_EDGE('',*,*,#17301,.F.);
#24583=ORIENTED_EDGE('',*,*,#17302,.T.);
#24584=ORIENTED_EDGE('',*,*,#17303,.T.);
#24585=ORIENTED_EDGE('',*,*,#17299,.F.);
#24586=ORIENTED_EDGE('',*,*,#17304,.F.);
#24587=ORIENTED_EDGE('',*,*,#17305,.T.);
#24588=ORIENTED_EDGE('',*,*,#17306,.T.);
#24589=ORIENTED_EDGE('',*,*,#17302,.F.);
#24590=ORIENTED_EDGE('',*,*,#17307,.F.);
#24591=ORIENTED_EDGE('',*,*,#17308,.T.);
#24592=ORIENTED_EDGE('',*,*,#17309,.T.);
#24593=ORIENTED_EDGE('',*,*,#17305,.F.);
#24594=ORIENTED_EDGE('',*,*,#17310,.F.);
#24595=ORIENTED_EDGE('',*,*,#17311,.T.);
#24596=ORIENTED_EDGE('',*,*,#17312,.T.);
#24597=ORIENTED_EDGE('',*,*,#17308,.F.);
#24598=ORIENTED_EDGE('',*,*,#17313,.F.);
#24599=ORIENTED_EDGE('',*,*,#17291,.T.);
#24600=ORIENTED_EDGE('',*,*,#17314,.T.);
#24601=ORIENTED_EDGE('',*,*,#17311,.F.);
#24602=ORIENTED_EDGE('',*,*,#17315,.F.);
#24603=ORIENTED_EDGE('',*,*,#17316,.T.);
#24604=ORIENTED_EDGE('',*,*,#17317,.T.);
#24605=ORIENTED_EDGE('',*,*,#17318,.F.);
#24606=ORIENTED_EDGE('',*,*,#17319,.F.);
#24607=ORIENTED_EDGE('',*,*,#17320,.T.);
#24608=ORIENTED_EDGE('',*,*,#17321,.T.);
#24609=ORIENTED_EDGE('',*,*,#17316,.F.);
#24610=ORIENTED_EDGE('',*,*,#17322,.F.);
#24611=ORIENTED_EDGE('',*,*,#17323,.T.);
#24612=ORIENTED_EDGE('',*,*,#17324,.T.);
#24613=ORIENTED_EDGE('',*,*,#17320,.F.);
#24614=ORIENTED_EDGE('',*,*,#17325,.F.);
#24615=ORIENTED_EDGE('',*,*,#17326,.T.);
#24616=ORIENTED_EDGE('',*,*,#17327,.T.);
#24617=ORIENTED_EDGE('',*,*,#17323,.F.);
#24618=ORIENTED_EDGE('',*,*,#17328,.F.);
#24619=ORIENTED_EDGE('',*,*,#17329,.T.);
#24620=ORIENTED_EDGE('',*,*,#17330,.T.);
#24621=ORIENTED_EDGE('',*,*,#17326,.F.);
#24622=ORIENTED_EDGE('',*,*,#17331,.F.);
#24623=ORIENTED_EDGE('',*,*,#17332,.T.);
#24624=ORIENTED_EDGE('',*,*,#17333,.T.);
#24625=ORIENTED_EDGE('',*,*,#17329,.F.);
#24626=ORIENTED_EDGE('',*,*,#17334,.F.);
#24627=ORIENTED_EDGE('',*,*,#17335,.T.);
#24628=ORIENTED_EDGE('',*,*,#17336,.T.);
#24629=ORIENTED_EDGE('',*,*,#17332,.F.);
#24630=ORIENTED_EDGE('',*,*,#17337,.F.);
#24631=ORIENTED_EDGE('',*,*,#17318,.T.);
#24632=ORIENTED_EDGE('',*,*,#17338,.T.);
#24633=ORIENTED_EDGE('',*,*,#17335,.F.);
#24634=ORIENTED_EDGE('',*,*,#17339,.F.);
#24635=ORIENTED_EDGE('',*,*,#17340,.T.);
#24636=ORIENTED_EDGE('',*,*,#17341,.T.);
#24637=ORIENTED_EDGE('',*,*,#17342,.F.);
#24638=ORIENTED_EDGE('',*,*,#17343,.F.);
#24639=ORIENTED_EDGE('',*,*,#17344,.T.);
#24640=ORIENTED_EDGE('',*,*,#17345,.T.);
#24641=ORIENTED_EDGE('',*,*,#17340,.F.);
#24642=ORIENTED_EDGE('',*,*,#17346,.F.);
#24643=ORIENTED_EDGE('',*,*,#17347,.T.);
#24644=ORIENTED_EDGE('',*,*,#17348,.T.);
#24645=ORIENTED_EDGE('',*,*,#17344,.F.);
#24646=ORIENTED_EDGE('',*,*,#17349,.F.);
#24647=ORIENTED_EDGE('',*,*,#17350,.T.);
#24648=ORIENTED_EDGE('',*,*,#17351,.T.);
#24649=ORIENTED_EDGE('',*,*,#17347,.F.);
#24650=ORIENTED_EDGE('',*,*,#17352,.F.);
#24651=ORIENTED_EDGE('',*,*,#17353,.T.);
#24652=ORIENTED_EDGE('',*,*,#17354,.T.);
#24653=ORIENTED_EDGE('',*,*,#17350,.F.);
#24654=ORIENTED_EDGE('',*,*,#17355,.F.);
#24655=ORIENTED_EDGE('',*,*,#17356,.T.);
#24656=ORIENTED_EDGE('',*,*,#17357,.T.);
#24657=ORIENTED_EDGE('',*,*,#17353,.F.);
#24658=ORIENTED_EDGE('',*,*,#17358,.F.);
#24659=ORIENTED_EDGE('',*,*,#17359,.T.);
#24660=ORIENTED_EDGE('',*,*,#17360,.T.);
#24661=ORIENTED_EDGE('',*,*,#17356,.F.);
#24662=ORIENTED_EDGE('',*,*,#17361,.F.);
#24663=ORIENTED_EDGE('',*,*,#17362,.T.);
#24664=ORIENTED_EDGE('',*,*,#17363,.T.);
#24665=ORIENTED_EDGE('',*,*,#17359,.F.);
#24666=ORIENTED_EDGE('',*,*,#17364,.F.);
#24667=ORIENTED_EDGE('',*,*,#17365,.T.);
#24668=ORIENTED_EDGE('',*,*,#17366,.T.);
#24669=ORIENTED_EDGE('',*,*,#17362,.F.);
#24670=ORIENTED_EDGE('',*,*,#17367,.F.);
#24671=ORIENTED_EDGE('',*,*,#17368,.T.);
#24672=ORIENTED_EDGE('',*,*,#17369,.T.);
#24673=ORIENTED_EDGE('',*,*,#17365,.F.);
#24674=ORIENTED_EDGE('',*,*,#17370,.F.);
#24675=ORIENTED_EDGE('',*,*,#17371,.T.);
#24676=ORIENTED_EDGE('',*,*,#17372,.T.);
#24677=ORIENTED_EDGE('',*,*,#17368,.F.);
#24678=ORIENTED_EDGE('',*,*,#17373,.F.);
#24679=ORIENTED_EDGE('',*,*,#17374,.T.);
#24680=ORIENTED_EDGE('',*,*,#17375,.T.);
#24681=ORIENTED_EDGE('',*,*,#17371,.F.);
#24682=ORIENTED_EDGE('',*,*,#17376,.F.);
#24683=ORIENTED_EDGE('',*,*,#17377,.T.);
#24684=ORIENTED_EDGE('',*,*,#17378,.T.);
#24685=ORIENTED_EDGE('',*,*,#17374,.F.);
#24686=ORIENTED_EDGE('',*,*,#17379,.F.);
#24687=ORIENTED_EDGE('',*,*,#17380,.T.);
#24688=ORIENTED_EDGE('',*,*,#17381,.T.);
#24689=ORIENTED_EDGE('',*,*,#17377,.F.);
#24690=ORIENTED_EDGE('',*,*,#17382,.F.);
#24691=ORIENTED_EDGE('',*,*,#17383,.T.);
#24692=ORIENTED_EDGE('',*,*,#17384,.T.);
#24693=ORIENTED_EDGE('',*,*,#17380,.F.);
#24694=ORIENTED_EDGE('',*,*,#17385,.F.);
#24695=ORIENTED_EDGE('',*,*,#17342,.T.);
#24696=ORIENTED_EDGE('',*,*,#17386,.T.);
#24697=ORIENTED_EDGE('',*,*,#17383,.F.);
#24698=ORIENTED_EDGE('',*,*,#17386,.F.);
#24699=ORIENTED_EDGE('',*,*,#17341,.F.);
#24700=ORIENTED_EDGE('',*,*,#17345,.F.);
#24701=ORIENTED_EDGE('',*,*,#17348,.F.);
#24702=ORIENTED_EDGE('',*,*,#17351,.F.);
#24703=ORIENTED_EDGE('',*,*,#17354,.F.);
#24704=ORIENTED_EDGE('',*,*,#17357,.F.);
#24705=ORIENTED_EDGE('',*,*,#17360,.F.);
#24706=ORIENTED_EDGE('',*,*,#17363,.F.);
#24707=ORIENTED_EDGE('',*,*,#17366,.F.);
#24708=ORIENTED_EDGE('',*,*,#17369,.F.);
#24709=ORIENTED_EDGE('',*,*,#17372,.F.);
#24710=ORIENTED_EDGE('',*,*,#17375,.F.);
#24711=ORIENTED_EDGE('',*,*,#17378,.F.);
#24712=ORIENTED_EDGE('',*,*,#17381,.F.);
#24713=ORIENTED_EDGE('',*,*,#17384,.F.);
#24714=ORIENTED_EDGE('',*,*,#17338,.F.);
#24715=ORIENTED_EDGE('',*,*,#17317,.F.);
#24716=ORIENTED_EDGE('',*,*,#17321,.F.);
#24717=ORIENTED_EDGE('',*,*,#17324,.F.);
#24718=ORIENTED_EDGE('',*,*,#17327,.F.);
#24719=ORIENTED_EDGE('',*,*,#17330,.F.);
#24720=ORIENTED_EDGE('',*,*,#17333,.F.);
#24721=ORIENTED_EDGE('',*,*,#17336,.F.);
#24722=ORIENTED_EDGE('',*,*,#17314,.F.);
#24723=ORIENTED_EDGE('',*,*,#17290,.F.);
#24724=ORIENTED_EDGE('',*,*,#17294,.F.);
#24725=ORIENTED_EDGE('',*,*,#17297,.F.);
#24726=ORIENTED_EDGE('',*,*,#17300,.F.);
#24727=ORIENTED_EDGE('',*,*,#17303,.F.);
#24728=ORIENTED_EDGE('',*,*,#17306,.F.);
#24729=ORIENTED_EDGE('',*,*,#17309,.F.);
#24730=ORIENTED_EDGE('',*,*,#17312,.F.);
#24731=ORIENTED_EDGE('',*,*,#17387,.F.);
#24732=ORIENTED_EDGE('',*,*,#17388,.T.);
#24733=ORIENTED_EDGE('',*,*,#17389,.T.);
#24734=ORIENTED_EDGE('',*,*,#17390,.F.);
#24735=ORIENTED_EDGE('',*,*,#17391,.F.);
#24736=ORIENTED_EDGE('',*,*,#17392,.T.);
#24737=ORIENTED_EDGE('',*,*,#17393,.T.);
#24738=ORIENTED_EDGE('',*,*,#17388,.F.);
#24739=ORIENTED_EDGE('',*,*,#17394,.F.);
#24740=ORIENTED_EDGE('',*,*,#17395,.T.);
#24741=ORIENTED_EDGE('',*,*,#17396,.T.);
#24742=ORIENTED_EDGE('',*,*,#17392,.F.);
#24743=ORIENTED_EDGE('',*,*,#17397,.F.);
#24744=ORIENTED_EDGE('',*,*,#17390,.T.);
#24745=ORIENTED_EDGE('',*,*,#17398,.T.);
#24746=ORIENTED_EDGE('',*,*,#17395,.F.);
#24747=ORIENTED_EDGE('',*,*,#17398,.F.);
#24748=ORIENTED_EDGE('',*,*,#17389,.F.);
#24749=ORIENTED_EDGE('',*,*,#17393,.F.);
#24750=ORIENTED_EDGE('',*,*,#17396,.F.);
#24751=ORIENTED_EDGE('',*,*,#17399,.F.);
#24752=ORIENTED_EDGE('',*,*,#17400,.T.);
#24753=ORIENTED_EDGE('',*,*,#17401,.T.);
#24754=ORIENTED_EDGE('',*,*,#17402,.F.);
#24755=ORIENTED_EDGE('',*,*,#17403,.F.);
#24756=ORIENTED_EDGE('',*,*,#17404,.T.);
#24757=ORIENTED_EDGE('',*,*,#17405,.T.);
#24758=ORIENTED_EDGE('',*,*,#17400,.F.);
#24759=ORIENTED_EDGE('',*,*,#17406,.F.);
#24760=ORIENTED_EDGE('',*,*,#17407,.T.);
#24761=ORIENTED_EDGE('',*,*,#17408,.T.);
#24762=ORIENTED_EDGE('',*,*,#17404,.F.);
#24763=ORIENTED_EDGE('',*,*,#17409,.F.);
#24764=ORIENTED_EDGE('',*,*,#17410,.T.);
#24765=ORIENTED_EDGE('',*,*,#17411,.T.);
#24766=ORIENTED_EDGE('',*,*,#17407,.F.);
#24767=ORIENTED_EDGE('',*,*,#17412,.F.);
#24768=ORIENTED_EDGE('',*,*,#17413,.T.);
#24769=ORIENTED_EDGE('',*,*,#17414,.T.);
#24770=ORIENTED_EDGE('',*,*,#17410,.F.);
#24771=ORIENTED_EDGE('',*,*,#17415,.F.);
#24772=ORIENTED_EDGE('',*,*,#17416,.T.);
#24773=ORIENTED_EDGE('',*,*,#17417,.T.);
#24774=ORIENTED_EDGE('',*,*,#17413,.F.);
#24775=ORIENTED_EDGE('',*,*,#17418,.F.);
#24776=ORIENTED_EDGE('',*,*,#17419,.T.);
#24777=ORIENTED_EDGE('',*,*,#17420,.T.);
#24778=ORIENTED_EDGE('',*,*,#17416,.F.);
#24779=ORIENTED_EDGE('',*,*,#17421,.F.);
#24780=ORIENTED_EDGE('',*,*,#17422,.T.);
#24781=ORIENTED_EDGE('',*,*,#17423,.T.);
#24782=ORIENTED_EDGE('',*,*,#17419,.F.);
#24783=ORIENTED_EDGE('',*,*,#17424,.F.);
#24784=ORIENTED_EDGE('',*,*,#17402,.T.);
#24785=ORIENTED_EDGE('',*,*,#17425,.T.);
#24786=ORIENTED_EDGE('',*,*,#17422,.F.);
#24787=ORIENTED_EDGE('',*,*,#17426,.F.);
#24788=ORIENTED_EDGE('',*,*,#17427,.T.);
#24789=ORIENTED_EDGE('',*,*,#17428,.T.);
#24790=ORIENTED_EDGE('',*,*,#17429,.F.);
#24791=ORIENTED_EDGE('',*,*,#17430,.F.);
#24792=ORIENTED_EDGE('',*,*,#17431,.T.);
#24793=ORIENTED_EDGE('',*,*,#17432,.T.);
#24794=ORIENTED_EDGE('',*,*,#17427,.F.);
#24795=ORIENTED_EDGE('',*,*,#17433,.F.);
#24796=ORIENTED_EDGE('',*,*,#17434,.T.);
#24797=ORIENTED_EDGE('',*,*,#17435,.T.);
#24798=ORIENTED_EDGE('',*,*,#17431,.F.);
#24799=ORIENTED_EDGE('',*,*,#17436,.F.);
#24800=ORIENTED_EDGE('',*,*,#17437,.T.);
#24801=ORIENTED_EDGE('',*,*,#17438,.T.);
#24802=ORIENTED_EDGE('',*,*,#17434,.F.);
#24803=ORIENTED_EDGE('',*,*,#17439,.F.);
#24804=ORIENTED_EDGE('',*,*,#17440,.T.);
#24805=ORIENTED_EDGE('',*,*,#17441,.T.);
#24806=ORIENTED_EDGE('',*,*,#17437,.F.);
#24807=ORIENTED_EDGE('',*,*,#17442,.F.);
#24808=ORIENTED_EDGE('',*,*,#17443,.T.);
#24809=ORIENTED_EDGE('',*,*,#17444,.T.);
#24810=ORIENTED_EDGE('',*,*,#17440,.F.);
#24811=ORIENTED_EDGE('',*,*,#17445,.F.);
#24812=ORIENTED_EDGE('',*,*,#17446,.T.);
#24813=ORIENTED_EDGE('',*,*,#17447,.T.);
#24814=ORIENTED_EDGE('',*,*,#17443,.F.);
#24815=ORIENTED_EDGE('',*,*,#17448,.F.);
#24816=ORIENTED_EDGE('',*,*,#17429,.T.);
#24817=ORIENTED_EDGE('',*,*,#17449,.T.);
#24818=ORIENTED_EDGE('',*,*,#17446,.F.);
#24819=ORIENTED_EDGE('',*,*,#17450,.F.);
#24820=ORIENTED_EDGE('',*,*,#17451,.T.);
#24821=ORIENTED_EDGE('',*,*,#17452,.T.);
#24822=ORIENTED_EDGE('',*,*,#17453,.F.);
#24823=ORIENTED_EDGE('',*,*,#17454,.F.);
#24824=ORIENTED_EDGE('',*,*,#17455,.T.);
#24825=ORIENTED_EDGE('',*,*,#17456,.T.);
#24826=ORIENTED_EDGE('',*,*,#17451,.F.);
#24827=ORIENTED_EDGE('',*,*,#17457,.F.);
#24828=ORIENTED_EDGE('',*,*,#17458,.T.);
#24829=ORIENTED_EDGE('',*,*,#17459,.T.);
#24830=ORIENTED_EDGE('',*,*,#17455,.F.);
#24831=ORIENTED_EDGE('',*,*,#17460,.F.);
#24832=ORIENTED_EDGE('',*,*,#17461,.T.);
#24833=ORIENTED_EDGE('',*,*,#17462,.T.);
#24834=ORIENTED_EDGE('',*,*,#17458,.F.);
#24835=ORIENTED_EDGE('',*,*,#17463,.F.);
#24836=ORIENTED_EDGE('',*,*,#17464,.T.);
#24837=ORIENTED_EDGE('',*,*,#17465,.T.);
#24838=ORIENTED_EDGE('',*,*,#17461,.F.);
#24839=ORIENTED_EDGE('',*,*,#17466,.F.);
#24840=ORIENTED_EDGE('',*,*,#17467,.T.);
#24841=ORIENTED_EDGE('',*,*,#17468,.T.);
#24842=ORIENTED_EDGE('',*,*,#17464,.F.);
#24843=ORIENTED_EDGE('',*,*,#17469,.F.);
#24844=ORIENTED_EDGE('',*,*,#17470,.T.);
#24845=ORIENTED_EDGE('',*,*,#17471,.T.);
#24846=ORIENTED_EDGE('',*,*,#17467,.F.);
#24847=ORIENTED_EDGE('',*,*,#17472,.F.);
#24848=ORIENTED_EDGE('',*,*,#17473,.T.);
#24849=ORIENTED_EDGE('',*,*,#17474,.T.);
#24850=ORIENTED_EDGE('',*,*,#17470,.F.);
#24851=ORIENTED_EDGE('',*,*,#17475,.F.);
#24852=ORIENTED_EDGE('',*,*,#17476,.T.);
#24853=ORIENTED_EDGE('',*,*,#17477,.T.);
#24854=ORIENTED_EDGE('',*,*,#17473,.F.);
#24855=ORIENTED_EDGE('',*,*,#17478,.F.);
#24856=ORIENTED_EDGE('',*,*,#17479,.T.);
#24857=ORIENTED_EDGE('',*,*,#17480,.T.);
#24858=ORIENTED_EDGE('',*,*,#17476,.F.);
#24859=ORIENTED_EDGE('',*,*,#17481,.F.);
#24860=ORIENTED_EDGE('',*,*,#17482,.T.);
#24861=ORIENTED_EDGE('',*,*,#17483,.T.);
#24862=ORIENTED_EDGE('',*,*,#17479,.F.);
#24863=ORIENTED_EDGE('',*,*,#17484,.F.);
#24864=ORIENTED_EDGE('',*,*,#17485,.T.);
#24865=ORIENTED_EDGE('',*,*,#17486,.T.);
#24866=ORIENTED_EDGE('',*,*,#17482,.F.);
#24867=ORIENTED_EDGE('',*,*,#17487,.F.);
#24868=ORIENTED_EDGE('',*,*,#17488,.T.);
#24869=ORIENTED_EDGE('',*,*,#17489,.T.);
#24870=ORIENTED_EDGE('',*,*,#17485,.F.);
#24871=ORIENTED_EDGE('',*,*,#17490,.F.);
#24872=ORIENTED_EDGE('',*,*,#17491,.T.);
#24873=ORIENTED_EDGE('',*,*,#17492,.T.);
#24874=ORIENTED_EDGE('',*,*,#17488,.F.);
#24875=ORIENTED_EDGE('',*,*,#17493,.F.);
#24876=ORIENTED_EDGE('',*,*,#17494,.T.);
#24877=ORIENTED_EDGE('',*,*,#17495,.T.);
#24878=ORIENTED_EDGE('',*,*,#17491,.F.);
#24879=ORIENTED_EDGE('',*,*,#17496,.F.);
#24880=ORIENTED_EDGE('',*,*,#17453,.T.);
#24881=ORIENTED_EDGE('',*,*,#17497,.T.);
#24882=ORIENTED_EDGE('',*,*,#17494,.F.);
#24883=ORIENTED_EDGE('',*,*,#17497,.F.);
#24884=ORIENTED_EDGE('',*,*,#17452,.F.);
#24885=ORIENTED_EDGE('',*,*,#17456,.F.);
#24886=ORIENTED_EDGE('',*,*,#17459,.F.);
#24887=ORIENTED_EDGE('',*,*,#17462,.F.);
#24888=ORIENTED_EDGE('',*,*,#17465,.F.);
#24889=ORIENTED_EDGE('',*,*,#17468,.F.);
#24890=ORIENTED_EDGE('',*,*,#17471,.F.);
#24891=ORIENTED_EDGE('',*,*,#17474,.F.);
#24892=ORIENTED_EDGE('',*,*,#17477,.F.);
#24893=ORIENTED_EDGE('',*,*,#17480,.F.);
#24894=ORIENTED_EDGE('',*,*,#17483,.F.);
#24895=ORIENTED_EDGE('',*,*,#17486,.F.);
#24896=ORIENTED_EDGE('',*,*,#17489,.F.);
#24897=ORIENTED_EDGE('',*,*,#17492,.F.);
#24898=ORIENTED_EDGE('',*,*,#17495,.F.);
#24899=ORIENTED_EDGE('',*,*,#17449,.F.);
#24900=ORIENTED_EDGE('',*,*,#17428,.F.);
#24901=ORIENTED_EDGE('',*,*,#17432,.F.);
#24902=ORIENTED_EDGE('',*,*,#17435,.F.);
#24903=ORIENTED_EDGE('',*,*,#17438,.F.);
#24904=ORIENTED_EDGE('',*,*,#17441,.F.);
#24905=ORIENTED_EDGE('',*,*,#17444,.F.);
#24906=ORIENTED_EDGE('',*,*,#17447,.F.);
#24907=ORIENTED_EDGE('',*,*,#17425,.F.);
#24908=ORIENTED_EDGE('',*,*,#17401,.F.);
#24909=ORIENTED_EDGE('',*,*,#17405,.F.);
#24910=ORIENTED_EDGE('',*,*,#17408,.F.);
#24911=ORIENTED_EDGE('',*,*,#17411,.F.);
#24912=ORIENTED_EDGE('',*,*,#17414,.F.);
#24913=ORIENTED_EDGE('',*,*,#17417,.F.);
#24914=ORIENTED_EDGE('',*,*,#17420,.F.);
#24915=ORIENTED_EDGE('',*,*,#17423,.F.);
#24916=ORIENTED_EDGE('',*,*,#17426,.T.);
#24917=ORIENTED_EDGE('',*,*,#17448,.T.);
#24918=ORIENTED_EDGE('',*,*,#17445,.T.);
#24919=ORIENTED_EDGE('',*,*,#17442,.T.);
#24920=ORIENTED_EDGE('',*,*,#17439,.T.);
#24921=ORIENTED_EDGE('',*,*,#17436,.T.);
#24922=ORIENTED_EDGE('',*,*,#17433,.T.);
#24923=ORIENTED_EDGE('',*,*,#17430,.T.);
#24924=ORIENTED_EDGE('',*,*,#17399,.T.);
#24925=ORIENTED_EDGE('',*,*,#17424,.T.);
#24926=ORIENTED_EDGE('',*,*,#17421,.T.);
#24927=ORIENTED_EDGE('',*,*,#17418,.T.);
#24928=ORIENTED_EDGE('',*,*,#17415,.T.);
#24929=ORIENTED_EDGE('',*,*,#17412,.T.);
#24930=ORIENTED_EDGE('',*,*,#17409,.T.);
#24931=ORIENTED_EDGE('',*,*,#17406,.T.);
#24932=ORIENTED_EDGE('',*,*,#17403,.T.);
#24933=ORIENTED_EDGE('',*,*,#17315,.T.);
#24934=ORIENTED_EDGE('',*,*,#17337,.T.);
#24935=ORIENTED_EDGE('',*,*,#17334,.T.);
#24936=ORIENTED_EDGE('',*,*,#17331,.T.);
#24937=ORIENTED_EDGE('',*,*,#17328,.T.);
#24938=ORIENTED_EDGE('',*,*,#17325,.T.);
#24939=ORIENTED_EDGE('',*,*,#17322,.T.);
#24940=ORIENTED_EDGE('',*,*,#17319,.T.);
#24941=ORIENTED_EDGE('',*,*,#17288,.T.);
#24942=ORIENTED_EDGE('',*,*,#17313,.T.);
#24943=ORIENTED_EDGE('',*,*,#17310,.T.);
#24944=ORIENTED_EDGE('',*,*,#17307,.T.);
#24945=ORIENTED_EDGE('',*,*,#17304,.T.);
#24946=ORIENTED_EDGE('',*,*,#17301,.T.);
#24947=ORIENTED_EDGE('',*,*,#17298,.T.);
#24948=ORIENTED_EDGE('',*,*,#17295,.T.);
#24949=ORIENTED_EDGE('',*,*,#17292,.T.);
#24950=ORIENTED_EDGE('',*,*,#17112,.T.);
#24951=ORIENTED_EDGE('',*,*,#17498,.T.);
#24952=ORIENTED_EDGE('',*,*,#17499,.F.);
#24953=ORIENTED_EDGE('',*,*,#17500,.F.);
#24954=ORIENTED_EDGE('',*,*,#17501,.T.);
#24955=ORIENTED_EDGE('',*,*,#17501,.F.);
#24956=ORIENTED_EDGE('',*,*,#17502,.F.);
#24957=ORIENTED_EDGE('',*,*,#17109,.F.);
#24958=ORIENTED_EDGE('',*,*,#17105,.F.);
#24959=ORIENTED_EDGE('',*,*,#17102,.F.);
#24960=ORIENTED_EDGE('',*,*,#17099,.F.);
#24961=ORIENTED_EDGE('',*,*,#17096,.F.);
#24962=ORIENTED_EDGE('',*,*,#17093,.F.);
#24963=ORIENTED_EDGE('',*,*,#17090,.F.);
#24964=ORIENTED_EDGE('',*,*,#17087,.F.);
#24965=ORIENTED_EDGE('',*,*,#17084,.F.);
#24966=ORIENTED_EDGE('',*,*,#17081,.F.);
#24967=ORIENTED_EDGE('',*,*,#17078,.F.);
#24968=ORIENTED_EDGE('',*,*,#17075,.F.);
#24969=ORIENTED_EDGE('',*,*,#17072,.F.);
#24970=ORIENTED_EDGE('',*,*,#17069,.F.);
#24971=ORIENTED_EDGE('',*,*,#17066,.F.);
#24972=ORIENTED_EDGE('',*,*,#17063,.F.);
#24973=ORIENTED_EDGE('',*,*,#17060,.F.);
#24974=ORIENTED_EDGE('',*,*,#17057,.F.);
#24975=ORIENTED_EDGE('',*,*,#17054,.F.);
#24976=ORIENTED_EDGE('',*,*,#17051,.F.);
#24977=ORIENTED_EDGE('',*,*,#17048,.F.);
#24978=ORIENTED_EDGE('',*,*,#17045,.F.);
#24979=ORIENTED_EDGE('',*,*,#17042,.F.);
#24980=ORIENTED_EDGE('',*,*,#17039,.F.);
#24981=ORIENTED_EDGE('',*,*,#17036,.F.);
#24982=ORIENTED_EDGE('',*,*,#17033,.F.);
#24983=ORIENTED_EDGE('',*,*,#17030,.F.);
#24984=ORIENTED_EDGE('',*,*,#17027,.F.);
#24985=ORIENTED_EDGE('',*,*,#17024,.F.);
#24986=ORIENTED_EDGE('',*,*,#17021,.F.);
#24987=ORIENTED_EDGE('',*,*,#17018,.F.);
#24988=ORIENTED_EDGE('',*,*,#17015,.F.);
#24989=ORIENTED_EDGE('',*,*,#17012,.F.);
#24990=ORIENTED_EDGE('',*,*,#17009,.F.);
#24991=ORIENTED_EDGE('',*,*,#17006,.F.);
#24992=ORIENTED_EDGE('',*,*,#17003,.F.);
#24993=ORIENTED_EDGE('',*,*,#17000,.F.);
#24994=ORIENTED_EDGE('',*,*,#16997,.F.);
#24995=ORIENTED_EDGE('',*,*,#16994,.F.);
#24996=ORIENTED_EDGE('',*,*,#16991,.F.);
#24997=ORIENTED_EDGE('',*,*,#16988,.F.);
#24998=ORIENTED_EDGE('',*,*,#16985,.F.);
#24999=ORIENTED_EDGE('',*,*,#16982,.F.);
#25000=ORIENTED_EDGE('',*,*,#16979,.F.);
#25001=ORIENTED_EDGE('',*,*,#16976,.F.);
#25002=ORIENTED_EDGE('',*,*,#16973,.F.);
#25003=ORIENTED_EDGE('',*,*,#16970,.F.);
#25004=ORIENTED_EDGE('',*,*,#16967,.F.);
#25005=ORIENTED_EDGE('',*,*,#16964,.F.);
#25006=ORIENTED_EDGE('',*,*,#16961,.F.);
#25007=ORIENTED_EDGE('',*,*,#16958,.F.);
#25008=ORIENTED_EDGE('',*,*,#16955,.F.);
#25009=ORIENTED_EDGE('',*,*,#16952,.F.);
#25010=ORIENTED_EDGE('',*,*,#16949,.F.);
#25011=ORIENTED_EDGE('',*,*,#16946,.F.);
#25012=ORIENTED_EDGE('',*,*,#16943,.F.);
#25013=ORIENTED_EDGE('',*,*,#16940,.F.);
#25014=ORIENTED_EDGE('',*,*,#16937,.F.);
#25015=ORIENTED_EDGE('',*,*,#16934,.F.);
#25016=ORIENTED_EDGE('',*,*,#16931,.F.);
#25017=ORIENTED_EDGE('',*,*,#17503,.F.);
#25018=ORIENTED_EDGE('',*,*,#17504,.T.);
#25019=ORIENTED_EDGE('',*,*,#17287,.T.);
#25020=ORIENTED_EDGE('',*,*,#17284,.T.);
#25021=ORIENTED_EDGE('',*,*,#17281,.T.);
#25022=ORIENTED_EDGE('',*,*,#17278,.T.);
#25023=ORIENTED_EDGE('',*,*,#17275,.T.);
#25024=ORIENTED_EDGE('',*,*,#17272,.T.);
#25025=ORIENTED_EDGE('',*,*,#17269,.T.);
#25026=ORIENTED_EDGE('',*,*,#17266,.T.);
#25027=ORIENTED_EDGE('',*,*,#17263,.T.);
#25028=ORIENTED_EDGE('',*,*,#17260,.T.);
#25029=ORIENTED_EDGE('',*,*,#17257,.T.);
#25030=ORIENTED_EDGE('',*,*,#17254,.T.);
#25031=ORIENTED_EDGE('',*,*,#17251,.T.);
#25032=ORIENTED_EDGE('',*,*,#17248,.T.);
#25033=ORIENTED_EDGE('',*,*,#17245,.T.);
#25034=ORIENTED_EDGE('',*,*,#17242,.T.);
#25035=ORIENTED_EDGE('',*,*,#17239,.T.);
#25036=ORIENTED_EDGE('',*,*,#17236,.T.);
#25037=ORIENTED_EDGE('',*,*,#17233,.T.);
#25038=ORIENTED_EDGE('',*,*,#17230,.T.);
#25039=ORIENTED_EDGE('',*,*,#17227,.T.);
#25040=ORIENTED_EDGE('',*,*,#17224,.T.);
#25041=ORIENTED_EDGE('',*,*,#17221,.T.);
#25042=ORIENTED_EDGE('',*,*,#17218,.T.);
#25043=ORIENTED_EDGE('',*,*,#17215,.T.);
#25044=ORIENTED_EDGE('',*,*,#17212,.T.);
#25045=ORIENTED_EDGE('',*,*,#17209,.T.);
#25046=ORIENTED_EDGE('',*,*,#17206,.T.);
#25047=ORIENTED_EDGE('',*,*,#17203,.T.);
#25048=ORIENTED_EDGE('',*,*,#17200,.T.);
#25049=ORIENTED_EDGE('',*,*,#17197,.T.);
#25050=ORIENTED_EDGE('',*,*,#17194,.T.);
#25051=ORIENTED_EDGE('',*,*,#17191,.T.);
#25052=ORIENTED_EDGE('',*,*,#17188,.T.);
#25053=ORIENTED_EDGE('',*,*,#17185,.T.);
#25054=ORIENTED_EDGE('',*,*,#17182,.T.);
#25055=ORIENTED_EDGE('',*,*,#17179,.T.);
#25056=ORIENTED_EDGE('',*,*,#17176,.T.);
#25057=ORIENTED_EDGE('',*,*,#17173,.T.);
#25058=ORIENTED_EDGE('',*,*,#17170,.T.);
#25059=ORIENTED_EDGE('',*,*,#17167,.T.);
#25060=ORIENTED_EDGE('',*,*,#17164,.T.);
#25061=ORIENTED_EDGE('',*,*,#17161,.T.);
#25062=ORIENTED_EDGE('',*,*,#17158,.T.);
#25063=ORIENTED_EDGE('',*,*,#17155,.T.);
#25064=ORIENTED_EDGE('',*,*,#17152,.T.);
#25065=ORIENTED_EDGE('',*,*,#17149,.T.);
#25066=ORIENTED_EDGE('',*,*,#17146,.T.);
#25067=ORIENTED_EDGE('',*,*,#17143,.T.);
#25068=ORIENTED_EDGE('',*,*,#17140,.T.);
#25069=ORIENTED_EDGE('',*,*,#17137,.T.);
#25070=ORIENTED_EDGE('',*,*,#17134,.T.);
#25071=ORIENTED_EDGE('',*,*,#17131,.T.);
#25072=ORIENTED_EDGE('',*,*,#17128,.T.);
#25073=ORIENTED_EDGE('',*,*,#17125,.T.);
#25074=ORIENTED_EDGE('',*,*,#17122,.T.);
#25075=ORIENTED_EDGE('',*,*,#17119,.T.);
#25076=ORIENTED_EDGE('',*,*,#17116,.T.);
#25077=ORIENTED_EDGE('',*,*,#17113,.T.);
#25078=ORIENTED_EDGE('',*,*,#17505,.T.);
#25079=ORIENTED_EDGE('',*,*,#17506,.T.);
#25080=ORIENTED_EDGE('',*,*,#17507,.T.);
#25081=ORIENTED_EDGE('',*,*,#17508,.T.);
#25082=ORIENTED_EDGE('',*,*,#17503,.T.);
#25083=ORIENTED_EDGE('',*,*,#17285,.T.);
#25084=ORIENTED_EDGE('',*,*,#17504,.F.);
#25085=ORIENTED_EDGE('',*,*,#17508,.F.);
#25086=ORIENTED_EDGE('',*,*,#17509,.T.);
#25087=ORIENTED_EDGE('',*,*,#17498,.F.);
#25088=ORIENTED_EDGE('',*,*,#17111,.F.);
#25089=ORIENTED_EDGE('',*,*,#17115,.F.);
#25090=ORIENTED_EDGE('',*,*,#17118,.F.);
#25091=ORIENTED_EDGE('',*,*,#17121,.F.);
#25092=ORIENTED_EDGE('',*,*,#17124,.F.);
#25093=ORIENTED_EDGE('',*,*,#17127,.F.);
#25094=ORIENTED_EDGE('',*,*,#17130,.F.);
#25095=ORIENTED_EDGE('',*,*,#17133,.F.);
#25096=ORIENTED_EDGE('',*,*,#17136,.F.);
#25097=ORIENTED_EDGE('',*,*,#17139,.F.);
#25098=ORIENTED_EDGE('',*,*,#17142,.F.);
#25099=ORIENTED_EDGE('',*,*,#17145,.F.);
#25100=ORIENTED_EDGE('',*,*,#17148,.F.);
#25101=ORIENTED_EDGE('',*,*,#17151,.F.);
#25102=ORIENTED_EDGE('',*,*,#17154,.F.);
#25103=ORIENTED_EDGE('',*,*,#17157,.F.);
#25104=ORIENTED_EDGE('',*,*,#17160,.F.);
#25105=ORIENTED_EDGE('',*,*,#17163,.F.);
#25106=ORIENTED_EDGE('',*,*,#17166,.F.);
#25107=ORIENTED_EDGE('',*,*,#17169,.F.);
#25108=ORIENTED_EDGE('',*,*,#17172,.F.);
#25109=ORIENTED_EDGE('',*,*,#17175,.F.);
#25110=ORIENTED_EDGE('',*,*,#17178,.F.);
#25111=ORIENTED_EDGE('',*,*,#17181,.F.);
#25112=ORIENTED_EDGE('',*,*,#17184,.F.);
#25113=ORIENTED_EDGE('',*,*,#17187,.F.);
#25114=ORIENTED_EDGE('',*,*,#17190,.F.);
#25115=ORIENTED_EDGE('',*,*,#17193,.F.);
#25116=ORIENTED_EDGE('',*,*,#17196,.F.);
#25117=ORIENTED_EDGE('',*,*,#17199,.F.);
#25118=ORIENTED_EDGE('',*,*,#17202,.F.);
#25119=ORIENTED_EDGE('',*,*,#17205,.F.);
#25120=ORIENTED_EDGE('',*,*,#17208,.F.);
#25121=ORIENTED_EDGE('',*,*,#17211,.F.);
#25122=ORIENTED_EDGE('',*,*,#17214,.F.);
#25123=ORIENTED_EDGE('',*,*,#17217,.F.);
#25124=ORIENTED_EDGE('',*,*,#17220,.F.);
#25125=ORIENTED_EDGE('',*,*,#17223,.F.);
#25126=ORIENTED_EDGE('',*,*,#17226,.F.);
#25127=ORIENTED_EDGE('',*,*,#17229,.F.);
#25128=ORIENTED_EDGE('',*,*,#17232,.F.);
#25129=ORIENTED_EDGE('',*,*,#17235,.F.);
#25130=ORIENTED_EDGE('',*,*,#17238,.F.);
#25131=ORIENTED_EDGE('',*,*,#17241,.F.);
#25132=ORIENTED_EDGE('',*,*,#17244,.F.);
#25133=ORIENTED_EDGE('',*,*,#17247,.F.);
#25134=ORIENTED_EDGE('',*,*,#17250,.F.);
#25135=ORIENTED_EDGE('',*,*,#17253,.F.);
#25136=ORIENTED_EDGE('',*,*,#17256,.F.);
#25137=ORIENTED_EDGE('',*,*,#17259,.F.);
#25138=ORIENTED_EDGE('',*,*,#17262,.F.);
#25139=ORIENTED_EDGE('',*,*,#17265,.F.);
#25140=ORIENTED_EDGE('',*,*,#17268,.F.);
#25141=ORIENTED_EDGE('',*,*,#17271,.F.);
#25142=ORIENTED_EDGE('',*,*,#17274,.F.);
#25143=ORIENTED_EDGE('',*,*,#17277,.F.);
#25144=ORIENTED_EDGE('',*,*,#17280,.F.);
#25145=ORIENTED_EDGE('',*,*,#17283,.F.);
#25146=ORIENTED_EDGE('',*,*,#17286,.F.);
#25147=ORIENTED_EDGE('',*,*,#17509,.F.);
#25148=ORIENTED_EDGE('',*,*,#17507,.F.);
#25149=ORIENTED_EDGE('',*,*,#16929,.F.);
#25150=ORIENTED_EDGE('',*,*,#16933,.F.);
#25151=ORIENTED_EDGE('',*,*,#16936,.F.);
#25152=ORIENTED_EDGE('',*,*,#16939,.F.);
#25153=ORIENTED_EDGE('',*,*,#16942,.F.);
#25154=ORIENTED_EDGE('',*,*,#16945,.F.);
#25155=ORIENTED_EDGE('',*,*,#16948,.F.);
#25156=ORIENTED_EDGE('',*,*,#16951,.F.);
#25157=ORIENTED_EDGE('',*,*,#16954,.F.);
#25158=ORIENTED_EDGE('',*,*,#16957,.F.);
#25159=ORIENTED_EDGE('',*,*,#16960,.F.);
#25160=ORIENTED_EDGE('',*,*,#16963,.F.);
#25161=ORIENTED_EDGE('',*,*,#16966,.F.);
#25162=ORIENTED_EDGE('',*,*,#16969,.F.);
#25163=ORIENTED_EDGE('',*,*,#16972,.F.);
#25164=ORIENTED_EDGE('',*,*,#16975,.F.);
#25165=ORIENTED_EDGE('',*,*,#16978,.F.);
#25166=ORIENTED_EDGE('',*,*,#16981,.F.);
#25167=ORIENTED_EDGE('',*,*,#16984,.F.);
#25168=ORIENTED_EDGE('',*,*,#16987,.F.);
#25169=ORIENTED_EDGE('',*,*,#16990,.F.);
#25170=ORIENTED_EDGE('',*,*,#16993,.F.);
#25171=ORIENTED_EDGE('',*,*,#16996,.F.);
#25172=ORIENTED_EDGE('',*,*,#16999,.F.);
#25173=ORIENTED_EDGE('',*,*,#17002,.F.);
#25174=ORIENTED_EDGE('',*,*,#17005,.F.);
#25175=ORIENTED_EDGE('',*,*,#17008,.F.);
#25176=ORIENTED_EDGE('',*,*,#17011,.F.);
#25177=ORIENTED_EDGE('',*,*,#17014,.F.);
#25178=ORIENTED_EDGE('',*,*,#17017,.F.);
#25179=ORIENTED_EDGE('',*,*,#17020,.F.);
#25180=ORIENTED_EDGE('',*,*,#17023,.F.);
#25181=ORIENTED_EDGE('',*,*,#17026,.F.);
#25182=ORIENTED_EDGE('',*,*,#17029,.F.);
#25183=ORIENTED_EDGE('',*,*,#17032,.F.);
#25184=ORIENTED_EDGE('',*,*,#17035,.F.);
#25185=ORIENTED_EDGE('',*,*,#17038,.F.);
#25186=ORIENTED_EDGE('',*,*,#17041,.F.);
#25187=ORIENTED_EDGE('',*,*,#17044,.F.);
#25188=ORIENTED_EDGE('',*,*,#17047,.F.);
#25189=ORIENTED_EDGE('',*,*,#17050,.F.);
#25190=ORIENTED_EDGE('',*,*,#17053,.F.);
#25191=ORIENTED_EDGE('',*,*,#17056,.F.);
#25192=ORIENTED_EDGE('',*,*,#17059,.F.);
#25193=ORIENTED_EDGE('',*,*,#17062,.F.);
#25194=ORIENTED_EDGE('',*,*,#17065,.F.);
#25195=ORIENTED_EDGE('',*,*,#17068,.F.);
#25196=ORIENTED_EDGE('',*,*,#17071,.F.);
#25197=ORIENTED_EDGE('',*,*,#17074,.F.);
#25198=ORIENTED_EDGE('',*,*,#17077,.F.);
#25199=ORIENTED_EDGE('',*,*,#17080,.F.);
#25200=ORIENTED_EDGE('',*,*,#17083,.F.);
#25201=ORIENTED_EDGE('',*,*,#17086,.F.);
#25202=ORIENTED_EDGE('',*,*,#17089,.F.);
#25203=ORIENTED_EDGE('',*,*,#17092,.F.);
#25204=ORIENTED_EDGE('',*,*,#17095,.F.);
#25205=ORIENTED_EDGE('',*,*,#17098,.F.);
#25206=ORIENTED_EDGE('',*,*,#17101,.F.);
#25207=ORIENTED_EDGE('',*,*,#17104,.F.);
#25208=ORIENTED_EDGE('',*,*,#17108,.F.);
#25209=ORIENTED_EDGE('',*,*,#17510,.T.);
#25210=ORIENTED_EDGE('',*,*,#17511,.T.);
#25211=ORIENTED_EDGE('',*,*,#17499,.T.);
#25212=ORIENTED_EDGE('',*,*,#17107,.T.);
#25213=ORIENTED_EDGE('',*,*,#17512,.T.);
#25214=ORIENTED_EDGE('',*,*,#17500,.T.);
#25215=ORIENTED_EDGE('',*,*,#17511,.F.);
#25216=ORIENTED_EDGE('',*,*,#17513,.F.);
#25217=ORIENTED_EDGE('',*,*,#17514,.F.);
#25218=ORIENTED_EDGE('',*,*,#17515,.F.);
#25219=ORIENTED_EDGE('',*,*,#17516,.F.);
#25220=ORIENTED_EDGE('',*,*,#17517,.F.);
#25221=ORIENTED_EDGE('',*,*,#17518,.F.);
#25222=ORIENTED_EDGE('',*,*,#17510,.F.);
#25223=ORIENTED_EDGE('',*,*,#17106,.T.);
#25224=ORIENTED_EDGE('',*,*,#17502,.T.);
#25225=ORIENTED_EDGE('',*,*,#17512,.F.);
#25226=ORIENTED_EDGE('',*,*,#17519,.F.);
#25227=ORIENTED_EDGE('',*,*,#17520,.F.);
#25228=ORIENTED_EDGE('',*,*,#17521,.F.);
#25229=ORIENTED_EDGE('',*,*,#17522,.F.);
#25230=ORIENTED_EDGE('',*,*,#17523,.F.);
#25231=ORIENTED_EDGE('',*,*,#17524,.T.);
#25232=ORIENTED_EDGE('',*,*,#17525,.F.);
#25233=ORIENTED_EDGE('',*,*,#17524,.F.);
#25234=ORIENTED_EDGE('',*,*,#17526,.F.);
#25235=ORIENTED_EDGE('',*,*,#17527,.F.);
#25236=ORIENTED_EDGE('',*,*,#17522,.T.);
#25237=ORIENTED_EDGE('',*,*,#17528,.F.);
#25238=ORIENTED_EDGE('',*,*,#17517,.T.);
#25239=ORIENTED_EDGE('',*,*,#17529,.T.);
#25240=ORIENTED_EDGE('',*,*,#17521,.T.);
#25241=ORIENTED_EDGE('',*,*,#17530,.F.);
#25242=ORIENTED_EDGE('',*,*,#17518,.T.);
#25243=ORIENTED_EDGE('',*,*,#17528,.T.);
#25244=ORIENTED_EDGE('',*,*,#17520,.T.);
#25245=ORIENTED_EDGE('',*,*,#17531,.F.);
#25246=ORIENTED_EDGE('',*,*,#17513,.T.);
#25247=ORIENTED_EDGE('',*,*,#17530,.T.);
#25248=ORIENTED_EDGE('',*,*,#17519,.T.);
#25249=ORIENTED_EDGE('',*,*,#17532,.F.);
#25250=ORIENTED_EDGE('',*,*,#17514,.T.);
#25251=ORIENTED_EDGE('',*,*,#17531,.T.);
#25252=ORIENTED_EDGE('',*,*,#17527,.T.);
#25253=ORIENTED_EDGE('',*,*,#17533,.F.);
#25254=ORIENTED_EDGE('',*,*,#17515,.T.);
#25255=ORIENTED_EDGE('',*,*,#17532,.T.);
#25256=ORIENTED_EDGE('',*,*,#17526,.T.);
#25257=ORIENTED_EDGE('',*,*,#17523,.T.);
#25258=ORIENTED_EDGE('',*,*,#17529,.F.);
#25259=ORIENTED_EDGE('',*,*,#17516,.T.);
#25260=ORIENTED_EDGE('',*,*,#17533,.T.);
#25261=ORIENTED_EDGE('',*,*,#17525,.T.);
#25262=ORIENTED_EDGE('',*,*,#17450,.T.);
#25263=ORIENTED_EDGE('',*,*,#17496,.T.);
#25264=ORIENTED_EDGE('',*,*,#17493,.T.);
#25265=ORIENTED_EDGE('',*,*,#17490,.T.);
#25266=ORIENTED_EDGE('',*,*,#17487,.T.);
#25267=ORIENTED_EDGE('',*,*,#17484,.T.);
#25268=ORIENTED_EDGE('',*,*,#17481,.T.);
#25269=ORIENTED_EDGE('',*,*,#17478,.T.);
#25270=ORIENTED_EDGE('',*,*,#17475,.T.);
#25271=ORIENTED_EDGE('',*,*,#17472,.T.);
#25272=ORIENTED_EDGE('',*,*,#17469,.T.);
#25273=ORIENTED_EDGE('',*,*,#17466,.T.);
#25274=ORIENTED_EDGE('',*,*,#17463,.T.);
#25275=ORIENTED_EDGE('',*,*,#17460,.T.);
#25276=ORIENTED_EDGE('',*,*,#17457,.T.);
#25277=ORIENTED_EDGE('',*,*,#17454,.T.);
#25278=ORIENTED_EDGE('',*,*,#17387,.T.);
#25279=ORIENTED_EDGE('',*,*,#17397,.T.);
#25280=ORIENTED_EDGE('',*,*,#17394,.T.);
#25281=ORIENTED_EDGE('',*,*,#17391,.T.);
#25282=ORIENTED_EDGE('',*,*,#17339,.T.);
#25283=ORIENTED_EDGE('',*,*,#17385,.T.);
#25284=ORIENTED_EDGE('',*,*,#17382,.T.);
#25285=ORIENTED_EDGE('',*,*,#17379,.T.);
#25286=ORIENTED_EDGE('',*,*,#17376,.T.);
#25287=ORIENTED_EDGE('',*,*,#17373,.T.);
#25288=ORIENTED_EDGE('',*,*,#17370,.T.);
#25289=ORIENTED_EDGE('',*,*,#17367,.T.);
#25290=ORIENTED_EDGE('',*,*,#17364,.T.);
#25291=ORIENTED_EDGE('',*,*,#17361,.T.);
#25292=ORIENTED_EDGE('',*,*,#17358,.T.);
#25293=ORIENTED_EDGE('',*,*,#17355,.T.);
#25294=ORIENTED_EDGE('',*,*,#17352,.T.);
#25295=ORIENTED_EDGE('',*,*,#17349,.T.);
#25296=ORIENTED_EDGE('',*,*,#17346,.T.);
#25297=ORIENTED_EDGE('',*,*,#17343,.T.);
#25298=ORIENTED_EDGE('',*,*,#17534,.F.);
#25299=ORIENTED_EDGE('',*,*,#17505,.F.);
#25300=ORIENTED_EDGE('',*,*,#16930,.F.);
#25301=ORIENTED_EDGE('',*,*,#17506,.F.);
#25302=ORIENTED_EDGE('',*,*,#17535,.T.);
#25303=ORIENTED_EDGE('',*,*,#17534,.T.);
#25304=ORIENTED_EDGE('',*,*,#17535,.F.);
#26803=PLANE('',#30407);
#26804=PLANE('',#30408);
#26805=PLANE('',#30409);
#26806=PLANE('',#30410);
#26807=PLANE('',#30411);
#26808=PLANE('',#30412);
#26809=PLANE('',#30413);
#26810=PLANE('',#30414);
#26811=PLANE('',#30415);
#26812=PLANE('',#30416);
#26813=PLANE('',#30417);
#26814=PLANE('',#30418);
#26815=PLANE('',#30421);
#26816=PLANE('',#30430);
#26817=PLANE('',#30434);
#26818=PLANE('',#30435);
#26819=PLANE('',#30436);
#26820=PLANE('',#30437);
#26821=PLANE('',#30438);
#26822=PLANE('',#30439);
#26823=PLANE('',#30440);
#26824=PLANE('',#30441);
#28071=ADVANCED_FACE('',(#4163),#1709,.T.);
#28072=ADVANCED_FACE('',(#4164),#1710,.T.);
#28073=ADVANCED_FACE('',(#4165),#1711,.T.);
#28074=ADVANCED_FACE('',(#4166),#1712,.T.);
#28075=ADVANCED_FACE('',(#4167),#1713,.T.);
#28076=ADVANCED_FACE('',(#4168),#1714,.T.);
#28077=ADVANCED_FACE('',(#4169),#1715,.T.);
#28078=ADVANCED_FACE('',(#4170),#1716,.T.);
#28079=ADVANCED_FACE('',(#4171),#1717,.T.);
#28080=ADVANCED_FACE('',(#4172),#1718,.T.);
#28081=ADVANCED_FACE('',(#4173),#1719,.T.);
#28082=ADVANCED_FACE('',(#4174),#1720,.T.);
#28083=ADVANCED_FACE('',(#4175),#1721,.T.);
#28084=ADVANCED_FACE('',(#4176),#1722,.T.);
#28085=ADVANCED_FACE('',(#4177),#1723,.T.);
#28086=ADVANCED_FACE('',(#4178),#1724,.T.);
#28087=ADVANCED_FACE('',(#4179),#1725,.T.);
#28088=ADVANCED_FACE('',(#4180),#1726,.T.);
#28089=ADVANCED_FACE('',(#4181),#1727,.T.);
#28090=ADVANCED_FACE('',(#4182),#1728,.T.);
#28091=ADVANCED_FACE('',(#4183),#1729,.T.);
#28092=ADVANCED_FACE('',(#4184),#1730,.T.);
#28093=ADVANCED_FACE('',(#4185),#1731,.T.);
#28094=ADVANCED_FACE('',(#4186),#1732,.T.);
#28095=ADVANCED_FACE('',(#4187),#1733,.T.);
#28096=ADVANCED_FACE('',(#4188),#1734,.T.);
#28097=ADVANCED_FACE('',(#4189),#1735,.T.);
#28098=ADVANCED_FACE('',(#4190),#1736,.T.);
#28099=ADVANCED_FACE('',(#4191),#1737,.T.);
#28100=ADVANCED_FACE('',(#4192),#1738,.T.);
#28101=ADVANCED_FACE('',(#4193),#1739,.T.);
#28102=ADVANCED_FACE('',(#4194),#1740,.T.);
#28103=ADVANCED_FACE('',(#4195),#1741,.T.);
#28104=ADVANCED_FACE('',(#4196),#1742,.T.);
#28105=ADVANCED_FACE('',(#4197),#1743,.T.);
#28106=ADVANCED_FACE('',(#4198),#1744,.T.);
#28107=ADVANCED_FACE('',(#4199),#1745,.T.);
#28108=ADVANCED_FACE('',(#4200),#1746,.T.);
#28109=ADVANCED_FACE('',(#4201),#1747,.T.);
#28110=ADVANCED_FACE('',(#4202),#1748,.T.);
#28111=ADVANCED_FACE('',(#4203),#1749,.T.);
#28112=ADVANCED_FACE('',(#4204),#1750,.T.);
#28113=ADVANCED_FACE('',(#4205),#1751,.T.);
#28114=ADVANCED_FACE('',(#4206),#1752,.T.);
#28115=ADVANCED_FACE('',(#4207),#1753,.T.);
#28116=ADVANCED_FACE('',(#4208),#1754,.T.);
#28117=ADVANCED_FACE('',(#4209),#1755,.T.);
#28118=ADVANCED_FACE('',(#4210),#1756,.T.);
#28119=ADVANCED_FACE('',(#4211),#1757,.T.);
#28120=ADVANCED_FACE('',(#4212),#1758,.T.);
#28121=ADVANCED_FACE('',(#4213),#1759,.T.);
#28122=ADVANCED_FACE('',(#4214),#1760,.T.);
#28123=ADVANCED_FACE('',(#4215),#1761,.T.);
#28124=ADVANCED_FACE('',(#4216),#1762,.T.);
#28125=ADVANCED_FACE('',(#4217),#1763,.T.);
#28126=ADVANCED_FACE('',(#4218),#1764,.T.);
#28127=ADVANCED_FACE('',(#4219),#1765,.T.);
#28128=ADVANCED_FACE('',(#4220),#1766,.T.);
#28129=ADVANCED_FACE('',(#4221),#1767,.T.);
#28130=ADVANCED_FACE('',(#4222),#1768,.T.);
#28131=ADVANCED_FACE('',(#4223),#1769,.T.);
#28132=ADVANCED_FACE('',(#4224),#1770,.T.);
#28133=ADVANCED_FACE('',(#4225),#1771,.T.);
#28134=ADVANCED_FACE('',(#4226),#1772,.T.);
#28135=ADVANCED_FACE('',(#4227),#1773,.T.);
#28136=ADVANCED_FACE('',(#4228),#1774,.T.);
#28137=ADVANCED_FACE('',(#4229),#1775,.T.);
#28138=ADVANCED_FACE('',(#4230),#1776,.T.);
#28139=ADVANCED_FACE('',(#4231),#1777,.T.);
#28140=ADVANCED_FACE('',(#4232),#1778,.T.);
#28141=ADVANCED_FACE('',(#4233),#1779,.T.);
#28142=ADVANCED_FACE('',(#4234),#1780,.T.);
#28143=ADVANCED_FACE('',(#4235),#1781,.T.);
#28144=ADVANCED_FACE('',(#4236),#1782,.T.);
#28145=ADVANCED_FACE('',(#4237),#1783,.T.);
#28146=ADVANCED_FACE('',(#4238),#1784,.T.);
#28147=ADVANCED_FACE('',(#4239),#1785,.T.);
#28148=ADVANCED_FACE('',(#4240),#1786,.T.);
#28149=ADVANCED_FACE('',(#4241),#1787,.T.);
#28150=ADVANCED_FACE('',(#4242),#1788,.T.);
#28151=ADVANCED_FACE('',(#4243),#1789,.T.);
#28152=ADVANCED_FACE('',(#4244),#1790,.T.);
#28153=ADVANCED_FACE('',(#4245),#1791,.T.);
#28154=ADVANCED_FACE('',(#4246),#1792,.T.);
#28155=ADVANCED_FACE('',(#4247),#1793,.T.);
#28156=ADVANCED_FACE('',(#4248),#1794,.T.);
#28157=ADVANCED_FACE('',(#4249),#1795,.T.);
#28158=ADVANCED_FACE('',(#4250),#1796,.T.);
#28159=ADVANCED_FACE('',(#4251),#1797,.T.);
#28160=ADVANCED_FACE('',(#4252),#1798,.T.);
#28161=ADVANCED_FACE('',(#4253),#1799,.T.);
#28162=ADVANCED_FACE('',(#4254),#1800,.T.);
#28163=ADVANCED_FACE('',(#4255),#1801,.T.);
#28164=ADVANCED_FACE('',(#4256),#1802,.T.);
#28165=ADVANCED_FACE('',(#4257),#1803,.T.);
#28166=ADVANCED_FACE('',(#4258),#1804,.T.);
#28167=ADVANCED_FACE('',(#4259),#1805,.T.);
#28168=ADVANCED_FACE('',(#4260),#1806,.T.);
#28169=ADVANCED_FACE('',(#4261),#1807,.T.);
#28170=ADVANCED_FACE('',(#4262),#1808,.T.);
#28171=ADVANCED_FACE('',(#4263),#1809,.T.);
#28172=ADVANCED_FACE('',(#4264),#1810,.T.);
#28173=ADVANCED_FACE('',(#4265),#1811,.T.);
#28174=ADVANCED_FACE('',(#4266),#1812,.T.);
#28175=ADVANCED_FACE('',(#4267),#1813,.T.);
#28176=ADVANCED_FACE('',(#4268),#1814,.T.);
#28177=ADVANCED_FACE('',(#4269),#1815,.T.);
#28178=ADVANCED_FACE('',(#4270),#1816,.T.);
#28179=ADVANCED_FACE('',(#4271),#1817,.T.);
#28180=ADVANCED_FACE('',(#4272),#1818,.T.);
#28181=ADVANCED_FACE('',(#4273),#1819,.T.);
#28182=ADVANCED_FACE('',(#4274),#1820,.T.);
#28183=ADVANCED_FACE('',(#4275),#1821,.T.);
#28184=ADVANCED_FACE('',(#4276),#1822,.T.);
#28185=ADVANCED_FACE('',(#4277),#1823,.T.);
#28186=ADVANCED_FACE('',(#4278),#1824,.T.);
#28187=ADVANCED_FACE('',(#4279),#1825,.T.);
#28188=ADVANCED_FACE('',(#4280),#1826,.T.);
#28189=ADVANCED_FACE('',(#4281),#1827,.T.);
#28190=ADVANCED_FACE('',(#4282),#1464,.F.);
#28191=ADVANCED_FACE('',(#4283),#1465,.F.);
#28192=ADVANCED_FACE('',(#4284),#1466,.F.);
#28193=ADVANCED_FACE('',(#4285),#1467,.F.);
#28194=ADVANCED_FACE('',(#4286),#1468,.F.);
#28195=ADVANCED_FACE('',(#4287),#1469,.F.);
#28196=ADVANCED_FACE('',(#4288),#1470,.F.);
#28197=ADVANCED_FACE('',(#4289),#1471,.F.);
#28198=ADVANCED_FACE('',(#4290),#1472,.F.);
#28199=ADVANCED_FACE('',(#4291),#1473,.F.);
#28200=ADVANCED_FACE('',(#4292),#1474,.F.);
#28201=ADVANCED_FACE('',(#4293),#1475,.F.);
#28202=ADVANCED_FACE('',(#4294),#1476,.F.);
#28203=ADVANCED_FACE('',(#4295),#1477,.F.);
#28204=ADVANCED_FACE('',(#4296),#1478,.F.);
#28205=ADVANCED_FACE('',(#4297),#1479,.F.);
#28206=ADVANCED_FACE('',(#4298),#1480,.F.);
#28207=ADVANCED_FACE('',(#4299),#1481,.F.);
#28208=ADVANCED_FACE('',(#4300),#1482,.F.);
#28209=ADVANCED_FACE('',(#4301),#1483,.F.);
#28210=ADVANCED_FACE('',(#4302),#1484,.F.);
#28211=ADVANCED_FACE('',(#4303),#1485,.F.);
#28212=ADVANCED_FACE('',(#4304),#1486,.F.);
#28213=ADVANCED_FACE('',(#4305),#1487,.F.);
#28214=ADVANCED_FACE('',(#4306),#1488,.F.);
#28215=ADVANCED_FACE('',(#4307),#1489,.F.);
#28216=ADVANCED_FACE('',(#4308),#1490,.F.);
#28217=ADVANCED_FACE('',(#4309),#1491,.F.);
#28218=ADVANCED_FACE('',(#4310),#1492,.F.);
#28219=ADVANCED_FACE('',(#4311),#1493,.F.);
#28220=ADVANCED_FACE('',(#4312),#1494,.F.);
#28221=ADVANCED_FACE('',(#4313),#1495,.F.);
#28222=ADVANCED_FACE('',(#4314),#1496,.F.);
#28223=ADVANCED_FACE('',(#4315,#1976,#1977),#26803,.T.);
#28224=ADVANCED_FACE('',(#4316),#26804,.F.);
#28225=ADVANCED_FACE('',(#4317),#26805,.F.);
#28226=ADVANCED_FACE('',(#4318),#26806,.F.);
#28227=ADVANCED_FACE('',(#4319),#26807,.F.);
#28228=ADVANCED_FACE('',(#4320),#26808,.F.);
#28229=ADVANCED_FACE('',(#4321),#1497,.F.);
#28230=ADVANCED_FACE('',(#4322),#1498,.F.);
#28231=ADVANCED_FACE('',(#4323),#1499,.F.);
#28232=ADVANCED_FACE('',(#4324),#1500,.F.);
#28233=ADVANCED_FACE('',(#4325),#1501,.F.);
#28234=ADVANCED_FACE('',(#4326),#1502,.F.);
#28235=ADVANCED_FACE('',(#4327),#1503,.F.);
#28236=ADVANCED_FACE('',(#4328),#1504,.F.);
#28237=ADVANCED_FACE('',(#4329),#1505,.F.);
#28238=ADVANCED_FACE('',(#4330),#1506,.F.);
#28239=ADVANCED_FACE('',(#4331),#1507,.F.);
#28240=ADVANCED_FACE('',(#4332),#1508,.F.);
#28241=ADVANCED_FACE('',(#4333),#1509,.F.);
#28242=ADVANCED_FACE('',(#4334),#1510,.F.);
#28243=ADVANCED_FACE('',(#4335),#1511,.F.);
#28244=ADVANCED_FACE('',(#4336),#1512,.F.);
#28245=ADVANCED_FACE('',(#4337),#1513,.F.);
#28246=ADVANCED_FACE('',(#4338),#1514,.F.);
#28247=ADVANCED_FACE('',(#4339),#1515,.F.);
#28248=ADVANCED_FACE('',(#4340),#1516,.F.);
#28249=ADVANCED_FACE('',(#4341),#1517,.F.);
#28250=ADVANCED_FACE('',(#4342),#1518,.F.);
#28251=ADVANCED_FACE('',(#4343),#1519,.F.);
#28252=ADVANCED_FACE('',(#4344),#1520,.F.);
#28253=ADVANCED_FACE('',(#4345),#1521,.F.);
#28254=ADVANCED_FACE('',(#4346),#1522,.F.);
#28255=ADVANCED_FACE('',(#4347),#1523,.F.);
#28256=ADVANCED_FACE('',(#4348),#1524,.F.);
#28257=ADVANCED_FACE('',(#4349),#1525,.F.);
#28258=ADVANCED_FACE('',(#4350),#1526,.F.);
#28259=ADVANCED_FACE('',(#4351),#1527,.F.);
#28260=ADVANCED_FACE('',(#4352),#1528,.F.);
#28261=ADVANCED_FACE('',(#4353),#1529,.F.);
#28262=ADVANCED_FACE('',(#4354,#1978,#1979),#26809,.T.);
#28263=ADVANCED_FACE('',(#4355),#26810,.T.);
#28264=ADVANCED_FACE('',(#4356),#26811,.T.);
#28265=ADVANCED_FACE('',(#4357),#26812,.T.);
#28266=ADVANCED_FACE('',(#4358),#26813,.T.);
#28267=ADVANCED_FACE('',(#4359),#26814,.F.);
#28268=ADVANCED_FACE('',(#4360),#1530,.F.);
#28269=ADVANCED_FACE('',(#4361),#26815,.T.);
#28270=ADVANCED_FACE('',(#4362),#1828,.T.);
#28271=ADVANCED_FACE('',(#4363),#1531,.F.);
#28272=ADVANCED_FACE('',(#4364),#381,.F.);
#28273=ADVANCED_FACE('',(#4365,#1980),#26816,.F.);
#28274=ADVANCED_FACE('',(#4366),#1829,.T.);
#28275=ADVANCED_FACE('',(#4367),#2893,.T.);
#28276=ADVANCED_FACE('',(#4368),#26817,.T.);
#28277=ADVANCED_FACE('',(#4369),#26818,.T.);
#28278=ADVANCED_FACE('',(#4370),#26819,.T.);
#28279=ADVANCED_FACE('',(#4371),#26820,.T.);
#28280=ADVANCED_FACE('',(#4372),#26821,.T.);
#28281=ADVANCED_FACE('',(#4373),#26822,.T.);
#28282=ADVANCED_FACE('',(#4374,#1981,#1982,#1983),#26823,.T.);
#28283=ADVANCED_FACE('',(#4375),#26824,.T.);
#28284=ADVANCED_FACE('',(#4376),#2894,.T.);
#28473=CLOSED_SHELL('',(#28071,#28072,#28073,#28074,#28075,#28076,#28077,
#28078,#28079,#28080,#28081,#28082,#28083,#28084,#28085,#28086,#28087,#28088,
#28089,#28090,#28091,#28092,#28093,#28094,#28095,#28096,#28097,#28098,#28099,
#28100,#28101,#28102,#28103,#28104,#28105,#28106,#28107,#28108,#28109,#28110,
#28111,#28112,#28113,#28114,#28115,#28116,#28117,#28118,#28119,#28120,#28121,
#28122,#28123,#28124,#28125,#28126,#28127,#28128,#28129,#28130,#28131,#28132,
#28133,#28134,#28135,#28136,#28137,#28138,#28139,#28140,#28141,#28142,#28143,
#28144,#28145,#28146,#28147,#28148,#28149,#28150,#28151,#28152,#28153,#28154,
#28155,#28156,#28157,#28158,#28159,#28160,#28161,#28162,#28163,#28164,#28165,
#28166,#28167,#28168,#28169,#28170,#28171,#28172,#28173,#28174,#28175,#28176,
#28177,#28178,#28179,#28180,#28181,#28182,#28183,#28184,#28185,#28186,#28187,
#28188,#28189,#28190,#28191,#28192,#28193,#28194,#28195,#28196,#28197,#28198,
#28199,#28200,#28201,#28202,#28203,#28204,#28205,#28206,#28207,#28208,#28209,
#28210,#28211,#28212,#28213,#28214,#28215,#28216,#28217,#28218,#28219,#28220,
#28221,#28222,#28223,#28224,#28225,#28226,#28227,#28228,#28229,#28230,#28231,
#28232,#28233,#28234,#28235,#28236,#28237,#28238,#28239,#28240,#28241,#28242,
#28243,#28244,#28245,#28246,#28247,#28248,#28249,#28250,#28251,#28252,#28253,
#28254,#28255,#28256,#28257,#28258,#28259,#28260,#28261,#28262,#28263,#28264,
#28265,#28266,#28267,#28268,#28269,#28270,#28271,#28272,#28273,#28274,#28275,
#28276,#28277,#28278,#28279,#28280,#28281,#28282,#28283,#28284));
#30284=AXIS2_PLACEMENT_3D('',#59077,#36123,#36124);
#30285=AXIS2_PLACEMENT_3D('',#59078,#36125,#36126);
#30286=AXIS2_PLACEMENT_3D('',#59094,#36128,#36129);
#30287=AXIS2_PLACEMENT_3D('',#59105,#36130,#36131);
#30288=AXIS2_PLACEMENT_3D('',#59171,#36133,#36134);
#30289=AXIS2_PLACEMENT_3D('',#59231,#36136,#36137);
#30290=AXIS2_PLACEMENT_3D('',#59291,#36139,#36140);
#30291=AXIS2_PLACEMENT_3D('',#59354,#36142,#36143);
#30292=AXIS2_PLACEMENT_3D('',#59414,#36145,#36146);
#30293=AXIS2_PLACEMENT_3D('',#59474,#36148,#36149);
#30294=AXIS2_PLACEMENT_3D('',#59537,#36151,#36152);
#30295=AXIS2_PLACEMENT_3D('',#59597,#36154,#36155);
#30296=AXIS2_PLACEMENT_3D('',#59663,#36157,#36158);
#30297=AXIS2_PLACEMENT_3D('',#59732,#36160,#36161);
#30298=AXIS2_PLACEMENT_3D('',#59798,#36163,#36164);
#30299=AXIS2_PLACEMENT_3D('',#59858,#36166,#36167);
#30300=AXIS2_PLACEMENT_3D('',#59921,#36169,#36170);
#30301=AXIS2_PLACEMENT_3D('',#59987,#36172,#36173);
#30302=AXIS2_PLACEMENT_3D('',#60047,#36175,#36176);
#30303=AXIS2_PLACEMENT_3D('',#60101,#36178,#36179);
#30304=AXIS2_PLACEMENT_3D('',#60155,#36181,#36182);
#30305=AXIS2_PLACEMENT_3D('',#60215,#36184,#36185);
#30306=AXIS2_PLACEMENT_3D('',#60281,#36187,#36188);
#30307=AXIS2_PLACEMENT_3D('',#60347,#36190,#36191);
#30308=AXIS2_PLACEMENT_3D('',#60416,#36193,#36194);
#30309=AXIS2_PLACEMENT_3D('',#60476,#36196,#36197);
#30310=AXIS2_PLACEMENT_3D('',#60539,#36199,#36200);
#30311=AXIS2_PLACEMENT_3D('',#60605,#36202,#36203);
#30312=AXIS2_PLACEMENT_3D('',#60671,#36205,#36206);
#30313=AXIS2_PLACEMENT_3D('',#60725,#36208,#36209);
#30314=AXIS2_PLACEMENT_3D('',#60779,#36211,#36212);
#30315=AXIS2_PLACEMENT_3D('',#60842,#36214,#36215);
#30316=AXIS2_PLACEMENT_3D('',#60908,#36217,#36218);
#30317=AXIS2_PLACEMENT_3D('',#60959,#36220,#36221);
#30318=AXIS2_PLACEMENT_3D('',#61022,#36223,#36224);
#30319=AXIS2_PLACEMENT_3D('',#61076,#36226,#36227);
#30320=AXIS2_PLACEMENT_3D('',#61139,#36229,#36230);
#30321=AXIS2_PLACEMENT_3D('',#61208,#36232,#36233);
#30322=AXIS2_PLACEMENT_3D('',#61271,#36235,#36236);
#30323=AXIS2_PLACEMENT_3D('',#61325,#36238,#36239);
#30324=AXIS2_PLACEMENT_3D('',#61385,#36241,#36242);
#30325=AXIS2_PLACEMENT_3D('',#61445,#36244,#36245);
#30326=AXIS2_PLACEMENT_3D('',#61505,#36247,#36248);
#30327=AXIS2_PLACEMENT_3D('',#61568,#36250,#36251);
#30328=AXIS2_PLACEMENT_3D('',#61622,#36253,#36254);
#30329=AXIS2_PLACEMENT_3D('',#61676,#36256,#36257);
#30330=AXIS2_PLACEMENT_3D('',#61742,#36259,#36260);
#30331=AXIS2_PLACEMENT_3D('',#61811,#36262,#36263);
#30332=AXIS2_PLACEMENT_3D('',#61874,#36265,#36266);
#30333=AXIS2_PLACEMENT_3D('',#61928,#36268,#36269);
#30334=AXIS2_PLACEMENT_3D('',#61994,#36271,#36272);
#30335=AXIS2_PLACEMENT_3D('',#62060,#36274,#36275);
#30336=AXIS2_PLACEMENT_3D('',#62120,#36277,#36278);
#30337=AXIS2_PLACEMENT_3D('',#62180,#36280,#36281);
#30338=AXIS2_PLACEMENT_3D('',#62234,#36283,#36284);
#30339=AXIS2_PLACEMENT_3D('',#62291,#36286,#36287);
#30340=AXIS2_PLACEMENT_3D('',#62357,#36289,#36290);
#30341=AXIS2_PLACEMENT_3D('',#62426,#36292,#36293);
#30342=AXIS2_PLACEMENT_3D('',#62489,#36295,#36296);
#30343=AXIS2_PLACEMENT_3D('',#62543,#36298,#36299);
#30344=AXIS2_PLACEMENT_3D('',#62609,#36301,#36302);
#30345=AXIS2_PLACEMENT_3D('',#62675,#36304,#36305);
#30346=AXIS2_PLACEMENT_3D('',#62680,#36307,#36308);
#30347=AXIS2_PLACEMENT_3D('',#62734,#36309,#36310);
#30348=AXIS2_PLACEMENT_3D('',#62756,#36312,#36313);
#30349=AXIS2_PLACEMENT_3D('',#62765,#36314,#36315);
#30350=AXIS2_PLACEMENT_3D('',#62795,#36317,#36318);
#30351=AXIS2_PLACEMENT_3D('',#62825,#36320,#36321);
#30352=AXIS2_PLACEMENT_3D('',#62870,#36323,#36324);
#30353=AXIS2_PLACEMENT_3D('',#62915,#36326,#36327);
#30354=AXIS2_PLACEMENT_3D('',#62945,#36329,#36330);
#30355=AXIS2_PLACEMENT_3D('',#62975,#36332,#36333);
#30356=AXIS2_PLACEMENT_3D('',#63004,#36335,#36336);
#30357=AXIS2_PLACEMENT_3D('',#63046,#36338,#36339);
#30358=AXIS2_PLACEMENT_3D('',#63076,#36341,#36342);
#30359=AXIS2_PLACEMENT_3D('',#63118,#36344,#36345);
#30360=AXIS2_PLACEMENT_3D('',#63148,#36347,#36348);
#30361=AXIS2_PLACEMENT_3D('',#63178,#36350,#36351);
#30362=AXIS2_PLACEMENT_3D('',#63220,#36353,#36354);
#30363=AXIS2_PLACEMENT_3D('',#63262,#36356,#36357);
#30364=AXIS2_PLACEMENT_3D('',#63292,#36359,#36360);
#30365=AXIS2_PLACEMENT_3D('',#63322,#36362,#36363);
#30366=AXIS2_PLACEMENT_3D('',#63364,#36365,#36366);
#30367=AXIS2_PLACEMENT_3D('',#63418,#36368,#36369);
#30368=AXIS2_PLACEMENT_3D('',#63448,#36371,#36372);
#30369=AXIS2_PLACEMENT_3D('',#63490,#36374,#36375);
#30370=AXIS2_PLACEMENT_3D('',#63519,#36377,#36378);
#30371=AXIS2_PLACEMENT_3D('',#63549,#36380,#36381);
#30372=AXIS2_PLACEMENT_3D('',#63592,#36383,#36384);
#30373=AXIS2_PLACEMENT_3D('',#63634,#36386,#36387);
#30374=AXIS2_PLACEMENT_3D('',#63664,#36389,#36390);
#30375=AXIS2_PLACEMENT_3D('',#63693,#36392,#36393);
#30376=AXIS2_PLACEMENT_3D('',#63735,#36395,#36396);
#30377=AXIS2_PLACEMENT_3D('',#63792,#36398,#36399);
#30378=AXIS2_PLACEMENT_3D('',#63821,#36401,#36402);
#30379=AXIS2_PLACEMENT_3D('',#63848,#36404,#36405);
#30380=AXIS2_PLACEMENT_3D('',#63877,#36407,#36408);
#30381=AXIS2_PLACEMENT_3D('',#63922,#36410,#36411);
#30382=AXIS2_PLACEMENT_3D('',#63965,#36413,#36414);
#30383=AXIS2_PLACEMENT_3D('',#64010,#36416,#36417);
#30384=AXIS2_PLACEMENT_3D('',#64040,#36419,#36420);
#30385=AXIS2_PLACEMENT_3D('',#64070,#36422,#36423);
#30386=AXIS2_PLACEMENT_3D('',#64099,#36425,#36426);
#30387=AXIS2_PLACEMENT_3D('',#64145,#36428,#36429);
#30388=AXIS2_PLACEMENT_3D('',#64175,#36431,#36432);
#30389=AXIS2_PLACEMENT_3D('',#64205,#36434,#36435);
#30390=AXIS2_PLACEMENT_3D('',#64234,#36437,#36438);
#30391=AXIS2_PLACEMENT_3D('',#64276,#36440,#36441);
#30392=AXIS2_PLACEMENT_3D('',#64319,#36443,#36444);
#30393=AXIS2_PLACEMENT_3D('',#64361,#36446,#36447);
#30394=AXIS2_PLACEMENT_3D('',#64391,#36449,#36450);
#30395=AXIS2_PLACEMENT_3D('',#64421,#36452,#36453);
#30396=AXIS2_PLACEMENT_3D('',#64450,#36455,#36456);
#30397=AXIS2_PLACEMENT_3D('',#64492,#36458,#36459);
#30398=AXIS2_PLACEMENT_3D('',#64523,#36461,#36462);
#30399=AXIS2_PLACEMENT_3D('',#64553,#36464,#36465);
#30400=AXIS2_PLACEMENT_3D('',#64595,#36467,#36468);
#30401=AXIS2_PLACEMENT_3D('',#64637,#36470,#36471);
#30402=AXIS2_PLACEMENT_3D('',#64668,#36473,#36474);
#30403=AXIS2_PLACEMENT_3D('',#64710,#36476,#36477);
#30404=AXIS2_PLACEMENT_3D('',#64740,#36479,#36480);
#30405=AXIS2_PLACEMENT_3D('',#64769,#36482,#36483);
#30406=AXIS2_PLACEMENT_3D('',#64799,#36485,#36486);
#30407=AXIS2_PLACEMENT_3D('',#65336,#36521,#36522);
#30408=AXIS2_PLACEMENT_3D('',#65337,#36523,#36524);
#30409=AXIS2_PLACEMENT_3D('',#65346,#36529,#36530);
#30410=AXIS2_PLACEMENT_3D('',#65352,#36534,#36535);
#30411=AXIS2_PLACEMENT_3D('',#65358,#36539,#36540);
#30412=AXIS2_PLACEMENT_3D('',#65361,#36543,#36544);
#30413=AXIS2_PLACEMENT_3D('',#65857,#36578,#36579);
#30414=AXIS2_PLACEMENT_3D('',#65858,#36580,#36581);
#30415=AXIS2_PLACEMENT_3D('',#65859,#36582,#36583);
#30416=AXIS2_PLACEMENT_3D('',#65860,#36584,#36585);
#30417=AXIS2_PLACEMENT_3D('',#65861,#36586,#36587);
#30418=AXIS2_PLACEMENT_3D('',#65862,#36588,#36589);
#30419=AXIS2_PLACEMENT_3D('',#65937,#36590,#36591);
#30420=AXIS2_PLACEMENT_3D('',#65939,#36592,#36593);
#30421=AXIS2_PLACEMENT_3D('',#68257,#36594,#36595);
#30422=AXIS2_PLACEMENT_3D('',#68259,#36596,#36597);
#30423=AXIS2_PLACEMENT_3D('',#68260,#36598,#36599);
#30424=AXIS2_PLACEMENT_3D('',#68338,#36600,#36601);
#30425=AXIS2_PLACEMENT_3D('',#68339,#36602,#36603);
#30426=AXIS2_PLACEMENT_3D('',#70502,#36604,#36605);
#30427=AXIS2_PLACEMENT_3D('',#70504,#36606,#36607);
#30428=AXIS2_PLACEMENT_3D('',#70505,#36608,#36609);
#30429=AXIS2_PLACEMENT_3D('',#70506,#36610,#36611);
#30430=AXIS2_PLACEMENT_3D('',#70507,#36612,#36613);
#30431=AXIS2_PLACEMENT_3D('',#70520,#36620,#36621);
#30432=AXIS2_PLACEMENT_3D('',#70521,#36622,#36623);
#30433=AXIS2_PLACEMENT_3D('',#70545,#36625,#36626);
#30434=AXIS2_PLACEMENT_3D('',#70553,#36627,#36628);
#30435=AXIS2_PLACEMENT_3D('',#70556,#36631,#36632);
#30436=AXIS2_PLACEMENT_3D('',#70558,#36634,#36635);
#30437=AXIS2_PLACEMENT_3D('',#70560,#36637,#36638);
#30438=AXIS2_PLACEMENT_3D('',#70562,#36640,#36641);
#30439=AXIS2_PLACEMENT_3D('',#70564,#36643,#36644);
#30440=AXIS2_PLACEMENT_3D('',#70565,#36645,#36646);
#30441=AXIS2_PLACEMENT_3D('',#70566,#36647,#36648);
#30442=AXIS2_PLACEMENT_3D('',#70568,#36649,#36650);
#30443=AXIS2_PLACEMENT_3D('',#70569,#36651,#36652);
#36123=DIRECTION('axis',(0.,0.,1.));
#36124=DIRECTION('refdir',(1.,0.,0.));
#36125=DIRECTION('center_axis',(0.,0.,1.));
#36126=DIRECTION('ref_axis',(1.,0.,0.));
#36127=DIRECTION('',(0.,0.,-1.));
#36128=DIRECTION('center_axis',(0.,0.,1.));
#36129=DIRECTION('ref_axis',(1.,0.,0.));
#36130=DIRECTION('center_axis',(0.,0.,1.));
#36131=DIRECTION('ref_axis',(1.,0.,0.));
#36132=DIRECTION('',(0.,0.,-1.));
#36133=DIRECTION('center_axis',(0.,0.,1.));
#36134=DIRECTION('ref_axis',(1.,0.,0.));
#36135=DIRECTION('',(0.,0.,-1.));
#36136=DIRECTION('center_axis',(0.,0.,1.));
#36137=DIRECTION('ref_axis',(1.,0.,0.));
#36138=DIRECTION('',(0.,0.,-1.));
#36139=DIRECTION('center_axis',(0.,0.,1.));
#36140=DIRECTION('ref_axis',(1.,0.,0.));
#36141=DIRECTION('',(0.,0.,-1.));
#36142=DIRECTION('center_axis',(0.,0.,1.));
#36143=DIRECTION('ref_axis',(1.,0.,0.));
#36144=DIRECTION('',(0.,0.,-1.));
#36145=DIRECTION('center_axis',(0.,0.,1.));
#36146=DIRECTION('ref_axis',(1.,0.,0.));
#36147=DIRECTION('',(0.,0.,-1.));
#36148=DIRECTION('center_axis',(0.,0.,1.));
#36149=DIRECTION('ref_axis',(1.,0.,0.));
#36150=DIRECTION('',(0.,0.,-1.));
#36151=DIRECTION('center_axis',(0.,0.,1.));
#36152=DIRECTION('ref_axis',(1.,0.,0.));
#36153=DIRECTION('',(0.,0.,-1.));
#36154=DIRECTION('center_axis',(0.,0.,1.));
#36155=DIRECTION('ref_axis',(1.,0.,0.));
#36156=DIRECTION('',(0.,0.,-1.));
#36157=DIRECTION('center_axis',(0.,0.,1.));
#36158=DIRECTION('ref_axis',(1.,0.,0.));
#36159=DIRECTION('',(0.,0.,-1.));
#36160=DIRECTION('center_axis',(0.,0.,1.));
#36161=DIRECTION('ref_axis',(1.,0.,0.));
#36162=DIRECTION('',(0.,0.,-1.));
#36163=DIRECTION('center_axis',(0.,0.,1.));
#36164=DIRECTION('ref_axis',(1.,0.,0.));
#36165=DIRECTION('',(0.,0.,-1.));
#36166=DIRECTION('center_axis',(0.,0.,1.));
#36167=DIRECTION('ref_axis',(1.,0.,0.));
#36168=DIRECTION('',(0.,0.,-1.));
#36169=DIRECTION('center_axis',(0.,0.,1.));
#36170=DIRECTION('ref_axis',(1.,0.,0.));
#36171=DIRECTION('',(0.,0.,-1.));
#36172=DIRECTION('center_axis',(0.,0.,1.));
#36173=DIRECTION('ref_axis',(1.,0.,0.));
#36174=DIRECTION('',(0.,0.,-1.));
#36175=DIRECTION('center_axis',(0.,0.,1.));
#36176=DIRECTION('ref_axis',(1.,0.,0.));
#36177=DIRECTION('',(0.,0.,-1.));
#36178=DIRECTION('center_axis',(0.,0.,1.));
#36179=DIRECTION('ref_axis',(1.,0.,0.));
#36180=DIRECTION('',(0.,0.,-1.));
#36181=DIRECTION('center_axis',(0.,0.,1.));
#36182=DIRECTION('ref_axis',(1.,0.,0.));
#36183=DIRECTION('',(0.,0.,-1.));
#36184=DIRECTION('center_axis',(0.,0.,1.));
#36185=DIRECTION('ref_axis',(1.,0.,0.));
#36186=DIRECTION('',(0.,0.,-1.));
#36187=DIRECTION('center_axis',(0.,0.,1.));
#36188=DIRECTION('ref_axis',(1.,0.,0.));
#36189=DIRECTION('',(0.,0.,-1.));
#36190=DIRECTION('center_axis',(0.,0.,1.));
#36191=DIRECTION('ref_axis',(1.,0.,0.));
#36192=DIRECTION('',(0.,0.,-1.));
#36193=DIRECTION('center_axis',(0.,0.,1.));
#36194=DIRECTION('ref_axis',(1.,0.,0.));
#36195=DIRECTION('',(0.,0.,-1.));
#36196=DIRECTION('center_axis',(0.,0.,1.));
#36197=DIRECTION('ref_axis',(1.,0.,0.));
#36198=DIRECTION('',(0.,0.,-1.));
#36199=DIRECTION('center_axis',(0.,0.,1.));
#36200=DIRECTION('ref_axis',(1.,0.,0.));
#36201=DIRECTION('',(0.,0.,-1.));
#36202=DIRECTION('center_axis',(0.,0.,1.));
#36203=DIRECTION('ref_axis',(1.,0.,0.));
#36204=DIRECTION('',(0.,0.,-1.));
#36205=DIRECTION('center_axis',(0.,0.,1.));
#36206=DIRECTION('ref_axis',(1.,0.,0.));
#36207=DIRECTION('',(0.,0.,-1.));
#36208=DIRECTION('center_axis',(0.,0.,1.));
#36209=DIRECTION('ref_axis',(1.,0.,0.));
#36210=DIRECTION('',(0.,0.,-1.));
#36211=DIRECTION('center_axis',(0.,0.,1.));
#36212=DIRECTION('ref_axis',(1.,0.,0.));
#36213=DIRECTION('',(0.,0.,-1.));
#36214=DIRECTION('center_axis',(0.,0.,1.));
#36215=DIRECTION('ref_axis',(1.,0.,0.));
#36216=DIRECTION('',(0.,0.,-1.));
#36217=DIRECTION('center_axis',(0.,0.,1.));
#36218=DIRECTION('ref_axis',(1.,0.,0.));
#36219=DIRECTION('',(0.,0.,-1.));
#36220=DIRECTION('center_axis',(0.,0.,1.));
#36221=DIRECTION('ref_axis',(1.,0.,0.));
#36222=DIRECTION('',(0.,0.,-1.));
#36223=DIRECTION('center_axis',(0.,0.,1.));
#36224=DIRECTION('ref_axis',(1.,0.,0.));
#36225=DIRECTION('',(0.,0.,-1.));
#36226=DIRECTION('center_axis',(0.,0.,1.));
#36227=DIRECTION('ref_axis',(1.,0.,0.));
#36228=DIRECTION('',(0.,0.,-1.));
#36229=DIRECTION('center_axis',(0.,0.,1.));
#36230=DIRECTION('ref_axis',(1.,0.,0.));
#36231=DIRECTION('',(0.,0.,-1.));
#36232=DIRECTION('center_axis',(0.,0.,1.));
#36233=DIRECTION('ref_axis',(1.,0.,0.));
#36234=DIRECTION('',(0.,0.,-1.));
#36235=DIRECTION('center_axis',(0.,0.,1.));
#36236=DIRECTION('ref_axis',(1.,0.,0.));
#36237=DIRECTION('',(0.,0.,-1.));
#36238=DIRECTION('center_axis',(0.,0.,1.));
#36239=DIRECTION('ref_axis',(1.,0.,0.));
#36240=DIRECTION('',(0.,0.,-1.));
#36241=DIRECTION('center_axis',(0.,0.,1.));
#36242=DIRECTION('ref_axis',(1.,0.,0.));
#36243=DIRECTION('',(0.,0.,-1.));
#36244=DIRECTION('center_axis',(0.,0.,1.));
#36245=DIRECTION('ref_axis',(1.,0.,0.));
#36246=DIRECTION('',(0.,0.,-1.));
#36247=DIRECTION('center_axis',(0.,0.,1.));
#36248=DIRECTION('ref_axis',(1.,0.,0.));
#36249=DIRECTION('',(0.,0.,-1.));
#36250=DIRECTION('center_axis',(0.,0.,1.));
#36251=DIRECTION('ref_axis',(1.,0.,0.));
#36252=DIRECTION('',(0.,0.,-1.));
#36253=DIRECTION('center_axis',(0.,0.,1.));
#36254=DIRECTION('ref_axis',(1.,0.,0.));
#36255=DIRECTION('',(0.,0.,-1.));
#36256=DIRECTION('center_axis',(0.,0.,1.));
#36257=DIRECTION('ref_axis',(1.,0.,0.));
#36258=DIRECTION('',(0.,0.,-1.));
#36259=DIRECTION('center_axis',(0.,0.,1.));
#36260=DIRECTION('ref_axis',(1.,0.,0.));
#36261=DIRECTION('',(0.,0.,-1.));
#36262=DIRECTION('center_axis',(0.,0.,1.));
#36263=DIRECTION('ref_axis',(1.,0.,0.));
#36264=DIRECTION('',(0.,0.,-1.));
#36265=DIRECTION('center_axis',(0.,0.,1.));
#36266=DIRECTION('ref_axis',(1.,0.,0.));
#36267=DIRECTION('',(0.,0.,-1.));
#36268=DIRECTION('center_axis',(0.,0.,1.));
#36269=DIRECTION('ref_axis',(1.,0.,0.));
#36270=DIRECTION('',(0.,0.,-1.));
#36271=DIRECTION('center_axis',(0.,0.,1.));
#36272=DIRECTION('ref_axis',(1.,0.,0.));
#36273=DIRECTION('',(0.,0.,-1.));
#36274=DIRECTION('center_axis',(0.,0.,1.));
#36275=DIRECTION('ref_axis',(1.,0.,0.));
#36276=DIRECTION('',(0.,0.,-1.));
#36277=DIRECTION('center_axis',(0.,0.,1.));
#36278=DIRECTION('ref_axis',(1.,0.,0.));
#36279=DIRECTION('',(0.,0.,-1.));
#36280=DIRECTION('center_axis',(0.,0.,1.));
#36281=DIRECTION('ref_axis',(1.,0.,0.));
#36282=DIRECTION('',(0.,0.,-1.));
#36283=DIRECTION('center_axis',(0.,0.,1.));
#36284=DIRECTION('ref_axis',(1.,0.,0.));
#36285=DIRECTION('',(0.,0.,-1.));
#36286=DIRECTION('center_axis',(0.,0.,1.));
#36287=DIRECTION('ref_axis',(1.,0.,0.));
#36288=DIRECTION('',(0.,0.,-1.));
#36289=DIRECTION('center_axis',(0.,0.,1.));
#36290=DIRECTION('ref_axis',(1.,0.,0.));
#36291=DIRECTION('',(0.,0.,-1.));
#36292=DIRECTION('center_axis',(0.,0.,1.));
#36293=DIRECTION('ref_axis',(1.,0.,0.));
#36294=DIRECTION('',(0.,0.,-1.));
#36295=DIRECTION('center_axis',(0.,0.,1.));
#36296=DIRECTION('ref_axis',(1.,0.,0.));
#36297=DIRECTION('',(0.,0.,-1.));
#36298=DIRECTION('center_axis',(0.,0.,1.));
#36299=DIRECTION('ref_axis',(1.,0.,0.));
#36300=DIRECTION('',(0.,0.,-1.));
#36301=DIRECTION('center_axis',(0.,0.,1.));
#36302=DIRECTION('ref_axis',(1.,0.,0.));
#36303=DIRECTION('',(0.,0.,-1.));
#36304=DIRECTION('center_axis',(0.,0.,1.));
#36305=DIRECTION('ref_axis',(1.,0.,0.));
#36306=DIRECTION('',(0.,0.,-1.));
#36307=DIRECTION('center_axis',(0.,0.,1.));
#36308=DIRECTION('ref_axis',(1.,0.,0.));
#36309=DIRECTION('center_axis',(0.,0.,1.));
#36310=DIRECTION('ref_axis',(0.288063002257283,-0.957611459168342,0.));
#36311=DIRECTION('',(0.,0.,1.));
#36312=DIRECTION('center_axis',(0.,0.,1.));
#36313=DIRECTION('ref_axis',(1.,-9.05137471385603E-13,0.));
#36314=DIRECTION('center_axis',(0.,0.,1.));
#36315=DIRECTION('ref_axis',(1.,-9.05137471385603E-13,0.));
#36316=DIRECTION('',(0.,0.,1.));
#36317=DIRECTION('center_axis',(0.,0.,1.));
#36318=DIRECTION('ref_axis',(1.,-9.05137471385603E-13,0.));
#36319=DIRECTION('',(0.,0.,1.));
#36320=DIRECTION('center_axis',(0.,0.,1.));
#36321=DIRECTION('ref_axis',(1.,-9.05137471385603E-13,0.));
#36322=DIRECTION('',(0.,0.,1.));
#36323=DIRECTION('center_axis',(0.,0.,1.));
#36324=DIRECTION('ref_axis',(1.,-9.05137471385603E-13,0.));
#36325=DIRECTION('',(0.,0.,1.));
#36326=DIRECTION('center_axis',(0.,0.,1.));
#36327=DIRECTION('ref_axis',(1.,-9.05137471385603E-13,0.));
#36328=DIRECTION('',(0.,0.,1.));
#36329=DIRECTION('center_axis',(0.,0.,1.));
#36330=DIRECTION('ref_axis',(1.,-9.05137471385603E-13,0.));
#36331=DIRECTION('',(0.,0.,1.));
#36332=DIRECTION('center_axis',(0.,0.,1.));
#36333=DIRECTION('ref_axis',(1.,-9.05137471385603E-13,0.));
#36334=DIRECTION('',(0.,0.,1.));
#36335=DIRECTION('center_axis',(0.,0.,1.));
#36336=DIRECTION('ref_axis',(1.,-9.05137471385603E-13,0.));
#36337=DIRECTION('',(0.,0.,1.));
#36338=DIRECTION('center_axis',(0.,0.,1.));
#36339=DIRECTION('ref_axis',(1.,-9.05137471385603E-13,0.));
#36340=DIRECTION('',(0.,0.,1.));
#36341=DIRECTION('center_axis',(0.,0.,1.));
#36342=DIRECTION('ref_axis',(1.,-9.05137471385603E-13,0.));
#36343=DIRECTION('',(0.,0.,1.));
#36344=DIRECTION('center_axis',(0.,0.,1.));
#36345=DIRECTION('ref_axis',(1.,-9.05137471385603E-13,0.));
#36346=DIRECTION('',(0.,0.,1.));
#36347=DIRECTION('center_axis',(0.,0.,1.));
#36348=DIRECTION('ref_axis',(1.,-9.05137471385603E-13,0.));
#36349=DIRECTION('',(0.,0.,1.));
#36350=DIRECTION('center_axis',(0.,0.,1.));
#36351=DIRECTION('ref_axis',(1.,-9.05137471385603E-13,0.));
#36352=DIRECTION('',(0.,0.,1.));
#36353=DIRECTION('center_axis',(0.,0.,1.));
#36354=DIRECTION('ref_axis',(1.,-9.05137471385603E-13,0.));
#36355=DIRECTION('',(0.,0.,1.));
#36356=DIRECTION('center_axis',(0.,0.,1.));
#36357=DIRECTION('ref_axis',(1.,-9.05137471385603E-13,0.));
#36358=DIRECTION('',(0.,0.,1.));
#36359=DIRECTION('center_axis',(0.,0.,1.));
#36360=DIRECTION('ref_axis',(1.,-9.05137471385603E-13,0.));
#36361=DIRECTION('',(0.,0.,1.));
#36362=DIRECTION('center_axis',(0.,0.,1.));
#36363=DIRECTION('ref_axis',(1.,-9.05137471385603E-13,0.));
#36364=DIRECTION('',(0.,0.,1.));
#36365=DIRECTION('center_axis',(0.,0.,1.));
#36366=DIRECTION('ref_axis',(1.,-9.05137471385603E-13,0.));
#36367=DIRECTION('',(0.,0.,1.));
#36368=DIRECTION('center_axis',(0.,0.,1.));
#36369=DIRECTION('ref_axis',(1.,-9.05137471385603E-13,0.));
#36370=DIRECTION('',(0.,0.,1.));
#36371=DIRECTION('center_axis',(0.,0.,1.));
#36372=DIRECTION('ref_axis',(1.,-9.05137471385603E-13,0.));
#36373=DIRECTION('',(0.,0.,1.));
#36374=DIRECTION('center_axis',(0.,0.,1.));
#36375=DIRECTION('ref_axis',(1.,-9.05137471385603E-13,0.));
#36376=DIRECTION('',(0.,0.,1.));
#36377=DIRECTION('center_axis',(0.,0.,1.));
#36378=DIRECTION('ref_axis',(1.,-9.05137471385603E-13,0.));
#36379=DIRECTION('',(0.,0.,1.));
#36380=DIRECTION('center_axis',(0.,0.,1.));
#36381=DIRECTION('ref_axis',(1.,-9.05137471385603E-13,0.));
#36382=DIRECTION('',(0.,0.,1.));
#36383=DIRECTION('center_axis',(0.,0.,1.));
#36384=DIRECTION('ref_axis',(1.,-9.05137471385603E-13,0.));
#36385=DIRECTION('',(0.,0.,1.));
#36386=DIRECTION('center_axis',(0.,0.,1.));
#36387=DIRECTION('ref_axis',(1.,-9.05137471385603E-13,0.));
#36388=DIRECTION('',(0.,0.,1.));
#36389=DIRECTION('center_axis',(0.,0.,1.));
#36390=DIRECTION('ref_axis',(1.,-9.05137471385603E-13,0.));
#36391=DIRECTION('',(0.,0.,1.));
#36392=DIRECTION('center_axis',(0.,0.,1.));
#36393=DIRECTION('ref_axis',(1.,-9.05137471385603E-13,0.));
#36394=DIRECTION('',(0.,0.,1.));
#36395=DIRECTION('center_axis',(0.,0.,1.));
#36396=DIRECTION('ref_axis',(1.,-9.05137471385603E-13,0.));
#36397=DIRECTION('',(0.,0.,1.));
#36398=DIRECTION('center_axis',(0.,0.,1.));
#36399=DIRECTION('ref_axis',(1.,-9.05137471385603E-13,0.));
#36400=DIRECTION('',(0.,0.,1.));
#36401=DIRECTION('center_axis',(0.,0.,1.));
#36402=DIRECTION('ref_axis',(1.,-9.05137471385603E-13,0.));
#36403=DIRECTION('',(0.,0.,1.));
#36404=DIRECTION('center_axis',(0.,0.,1.));
#36405=DIRECTION('ref_axis',(1.,-9.05137471385603E-13,0.));
#36406=DIRECTION('',(0.,0.,1.));
#36407=DIRECTION('center_axis',(0.,0.,1.));
#36408=DIRECTION('ref_axis',(1.,-9.05137471385603E-13,0.));
#36409=DIRECTION('',(0.,0.,1.));
#36410=DIRECTION('center_axis',(0.,0.,1.));
#36411=DIRECTION('ref_axis',(1.,-9.05137471385603E-13,0.));
#36412=DIRECTION('',(0.,0.,1.));
#36413=DIRECTION('center_axis',(0.,0.,1.));
#36414=DIRECTION('ref_axis',(1.,-9.05137471385603E-13,0.));
#36415=DIRECTION('',(0.,0.,1.));
#36416=DIRECTION('center_axis',(0.,0.,1.));
#36417=DIRECTION('ref_axis',(1.,-9.05137471385603E-13,0.));
#36418=DIRECTION('',(0.,0.,1.));
#36419=DIRECTION('center_axis',(0.,0.,1.));
#36420=DIRECTION('ref_axis',(1.,-9.05137471385603E-13,0.));
#36421=DIRECTION('',(0.,0.,1.));
#36422=DIRECTION('center_axis',(0.,0.,1.));
#36423=DIRECTION('ref_axis',(1.,-9.05137471385603E-13,0.));
#36424=DIRECTION('',(0.,0.,1.));
#36425=DIRECTION('center_axis',(0.,0.,1.));
#36426=DIRECTION('ref_axis',(1.,-9.05137471385603E-13,0.));
#36427=DIRECTION('',(0.,0.,1.));
#36428=DIRECTION('center_axis',(0.,0.,1.));
#36429=DIRECTION('ref_axis',(1.,-9.05137471385603E-13,0.));
#36430=DIRECTION('',(0.,0.,1.));
#36431=DIRECTION('center_axis',(0.,0.,1.));
#36432=DIRECTION('ref_axis',(1.,-9.05137471385603E-13,0.));
#36433=DIRECTION('',(0.,0.,1.));
#36434=DIRECTION('center_axis',(0.,0.,1.));
#36435=DIRECTION('ref_axis',(1.,-9.05137471385603E-13,0.));
#36436=DIRECTION('',(0.,0.,1.));
#36437=DIRECTION('center_axis',(0.,0.,1.));
#36438=DIRECTION('ref_axis',(1.,-9.05137471385603E-13,0.));
#36439=DIRECTION('',(0.,0.,1.));
#36440=DIRECTION('center_axis',(0.,0.,1.));
#36441=DIRECTION('ref_axis',(1.,-9.05137471385603E-13,0.));
#36442=DIRECTION('',(0.,0.,1.));
#36443=DIRECTION('center_axis',(0.,0.,1.));
#36444=DIRECTION('ref_axis',(1.,-9.05137471385603E-13,0.));
#36445=DIRECTION('',(0.,0.,1.));
#36446=DIRECTION('center_axis',(0.,0.,1.));
#36447=DIRECTION('ref_axis',(1.,-9.05137471385603E-13,0.));
#36448=DIRECTION('',(0.,0.,1.));
#36449=DIRECTION('center_axis',(0.,0.,1.));
#36450=DIRECTION('ref_axis',(1.,-9.05137471385603E-13,0.));
#36451=DIRECTION('',(0.,0.,1.));
#36452=DIRECTION('center_axis',(0.,0.,1.));
#36453=DIRECTION('ref_axis',(1.,-9.05137471385603E-13,0.));
#36454=DIRECTION('',(0.,0.,1.));
#36455=DIRECTION('center_axis',(0.,0.,1.));
#36456=DIRECTION('ref_axis',(1.,-9.05137471385603E-13,0.));
#36457=DIRECTION('',(0.,0.,1.));
#36458=DIRECTION('center_axis',(0.,0.,1.));
#36459=DIRECTION('ref_axis',(1.,-9.05137471385603E-13,0.));
#36460=DIRECTION('',(0.,0.,1.));
#36461=DIRECTION('center_axis',(0.,0.,1.));
#36462=DIRECTION('ref_axis',(1.,-9.05137471385603E-13,0.));
#36463=DIRECTION('',(0.,0.,1.));
#36464=DIRECTION('center_axis',(0.,0.,1.));
#36465=DIRECTION('ref_axis',(1.,-9.05137471385603E-13,0.));
#36466=DIRECTION('',(0.,0.,1.));
#36467=DIRECTION('center_axis',(0.,0.,1.));
#36468=DIRECTION('ref_axis',(1.,-9.05137471385603E-13,0.));
#36469=DIRECTION('',(0.,0.,1.));
#36470=DIRECTION('center_axis',(0.,0.,1.));
#36471=DIRECTION('ref_axis',(1.,-9.05137471385603E-13,0.));
#36472=DIRECTION('',(0.,0.,1.));
#36473=DIRECTION('center_axis',(0.,0.,1.));
#36474=DIRECTION('ref_axis',(1.,-9.05137471385603E-13,0.));
#36475=DIRECTION('',(0.,0.,1.));
#36476=DIRECTION('center_axis',(0.,0.,1.));
#36477=DIRECTION('ref_axis',(1.,-9.05137471385603E-13,0.));
#36478=DIRECTION('',(0.,0.,1.));
#36479=DIRECTION('center_axis',(0.,0.,1.));
#36480=DIRECTION('ref_axis',(1.,-9.05137471385603E-13,0.));
#36481=DIRECTION('',(0.,0.,1.));
#36482=DIRECTION('center_axis',(0.,0.,1.));
#36483=DIRECTION('ref_axis',(1.,-9.05137471385603E-13,0.));
#36484=DIRECTION('',(0.,0.,1.));
#36485=DIRECTION('center_axis',(0.,0.,1.));
#36486=DIRECTION('ref_axis',(1.,-9.05137471385603E-13,0.));
#36487=DIRECTION('',(0.,0.,1.));
#36488=DIRECTION('',(0.,0.,-1.));
#36489=DIRECTION('',(0.,0.,-1.));
#36490=DIRECTION('',(0.,0.,-1.));
#36491=DIRECTION('',(0.,0.,-1.));
#36492=DIRECTION('',(0.,0.,-1.));
#36493=DIRECTION('',(0.,0.,-1.));
#36494=DIRECTION('',(0.,0.,-1.));
#36495=DIRECTION('',(0.,0.,-1.));
#36496=DIRECTION('',(0.,0.,-1.));
#36497=DIRECTION('',(0.,0.,-1.));
#36498=DIRECTION('',(0.,0.,-1.));
#36499=DIRECTION('',(0.,0.,-1.));
#36500=DIRECTION('',(0.,0.,-1.));
#36501=DIRECTION('',(0.,0.,-1.));
#36502=DIRECTION('',(0.,0.,-1.));
#36503=DIRECTION('',(0.,0.,-1.));
#36504=DIRECTION('',(0.,0.,-1.));
#36505=DIRECTION('',(0.,0.,-1.));
#36506=DIRECTION('',(0.,0.,-1.));
#36507=DIRECTION('',(0.,0.,-1.));
#36508=DIRECTION('',(0.,0.,-1.));
#36509=DIRECTION('',(0.,0.,-1.));
#36510=DIRECTION('',(0.,0.,-1.));
#36511=DIRECTION('',(0.,0.,-1.));
#36512=DIRECTION('',(0.,0.,-1.));
#36513=DIRECTION('',(0.,0.,-1.));
#36514=DIRECTION('',(0.,0.,-1.));
#36515=DIRECTION('',(0.,0.,-1.));
#36516=DIRECTION('',(0.,0.,-1.));
#36517=DIRECTION('',(0.,0.,-1.));
#36518=DIRECTION('',(0.,0.,-1.));
#36519=DIRECTION('',(0.,0.,-1.));
#36520=DIRECTION('',(0.,0.,-1.));
#36521=DIRECTION('center_axis',(0.,0.,1.));
#36522=DIRECTION('ref_axis',(1.,0.,0.));
#36523=DIRECTION('center_axis',(0.,1.,0.));
#36524=DIRECTION('ref_axis',(1.,0.,0.));
#36525=DIRECTION('',(1.,0.,0.));
#36526=DIRECTION('',(0.,0.,-1.));
#36527=DIRECTION('',(1.,0.,0.));
#36528=DIRECTION('',(0.,0.,-1.));
#36529=DIRECTION('center_axis',(-1.,0.,0.));
#36530=DIRECTION('ref_axis',(0.,1.,0.));
#36531=DIRECTION('',(0.,1.,0.));
#36532=DIRECTION('',(0.,0.,-1.));
#36533=DIRECTION('',(0.,1.,0.));
#36534=DIRECTION('center_axis',(0.,-1.,0.));
#36535=DIRECTION('ref_axis',(-1.,0.,0.));
#36536=DIRECTION('',(-1.,0.,0.));
#36537=DIRECTION('',(0.,0.,-1.));
#36538=DIRECTION('',(-1.,0.,0.));
#36539=DIRECTION('center_axis',(1.,0.,0.));
#36540=DIRECTION('ref_axis',(0.,-1.,0.));
#36541=DIRECTION('',(0.,-1.,0.));
#36542=DIRECTION('',(0.,-1.,0.));
#36543=DIRECTION('center_axis',(0.,0.,-1.));
#36544=DIRECTION('ref_axis',(-1.,0.,0.));
#36545=DIRECTION('',(0.,0.,-1.));
#36546=DIRECTION('',(0.,0.,-1.));
#36547=DIRECTION('',(0.,0.,-1.));
#36548=DIRECTION('',(0.,0.,-1.));
#36549=DIRECTION('',(0.,0.,-1.));
#36550=DIRECTION('',(0.,0.,-1.));
#36551=DIRECTION('',(0.,0.,-1.));
#36552=DIRECTION('',(0.,0.,-1.));
#36553=DIRECTION('',(0.,0.,-1.));
#36554=DIRECTION('',(0.,0.,-1.));
#36555=DIRECTION('',(0.,0.,-1.));
#36556=DIRECTION('',(0.,0.,-1.));
#36557=DIRECTION('',(0.,0.,-1.));
#36558=DIRECTION('',(0.,0.,-1.));
#36559=DIRECTION('',(0.,0.,-1.));
#36560=DIRECTION('',(0.,0.,-1.));
#36561=DIRECTION('',(0.,0.,-1.));
#36562=DIRECTION('',(0.,0.,-1.));
#36563=DIRECTION('',(0.,0.,-1.));
#36564=DIRECTION('',(0.,0.,-1.));
#36565=DIRECTION('',(0.,0.,-1.));
#36566=DIRECTION('',(0.,0.,-1.));
#36567=DIRECTION('',(0.,0.,-1.));
#36568=DIRECTION('',(0.,0.,-1.));
#36569=DIRECTION('',(0.,0.,-1.));
#36570=DIRECTION('',(0.,0.,-1.));
#36571=DIRECTION('',(0.,0.,-1.));
#36572=DIRECTION('',(0.,0.,-1.));
#36573=DIRECTION('',(0.,0.,-1.));
#36574=DIRECTION('',(0.,0.,-1.));
#36575=DIRECTION('',(0.,0.,-1.));
#36576=DIRECTION('',(0.,0.,-1.));
#36577=DIRECTION('',(0.,0.,-1.));
#36578=DIRECTION('center_axis',(0.,0.,1.));
#36579=DIRECTION('ref_axis',(1.,0.,0.));
#36580=DIRECTION('center_axis',(0.,0.,1.));
#36581=DIRECTION('ref_axis',(1.,0.,0.));
#36582=DIRECTION('center_axis',(0.,0.,1.));
#36583=DIRECTION('ref_axis',(1.,0.,0.));
#36584=DIRECTION('center_axis',(0.,0.,1.));
#36585=DIRECTION('ref_axis',(1.,0.,0.));
#36586=DIRECTION('center_axis',(0.,0.,1.));
#36587=DIRECTION('ref_axis',(1.,0.,0.));
#36588=DIRECTION('center_axis',(0.,0.,1.));
#36589=DIRECTION('ref_axis',(1.,0.,0.));
#36590=DIRECTION('center_axis',(0.,0.,1.));
#36591=DIRECTION('ref_axis',(1.,0.,0.));
#36592=DIRECTION('center_axis',(0.,0.,1.));
#36593=DIRECTION('ref_axis',(1.,0.,0.));
#36594=DIRECTION('center_axis',(0.,0.,1.));
#36595=DIRECTION('ref_axis',(1.,0.,0.));
#36596=DIRECTION('center_axis',(0.,0.,1.));
#36597=DIRECTION('ref_axis',(1.,0.,0.));
#36598=DIRECTION('center_axis',(0.,0.,1.));
#36599=DIRECTION('ref_axis',(1.,0.,0.));
#36600=DIRECTION('center_axis',(0.,0.,-1.));
#36601=DIRECTION('ref_axis',(1.,-9.05137471385603E-13,0.));
#36602=DIRECTION('center_axis',(0.,0.,1.));
#36603=DIRECTION('ref_axis',(1.,-9.05137471385603E-13,0.));
#36604=DIRECTION('center_axis',(0.,0.,-1.));
#36605=DIRECTION('ref_axis',(-1.,0.,0.));
#36606=DIRECTION('center_axis',(0.,0.,-1.));
#36607=DIRECTION('ref_axis',(1.,0.,0.));
#36608=DIRECTION('center_axis',(-1.22464679914735E-16,-1.,0.));
#36609=DIRECTION('ref_axis',(1.,-1.22464679914735E-16,0.));
#36610=DIRECTION('center_axis',(0.,0.,1.));
#36611=DIRECTION('ref_axis',(1.,0.,0.));
#36612=DIRECTION('center_axis',(0.,0.,1.));
#36613=DIRECTION('ref_axis',(1.,0.,0.));
#36614=DIRECTION('',(3.20493781063927E-16,1.,0.));
#36615=DIRECTION('',(0.866025403784439,0.5,0.));
#36616=DIRECTION('',(0.866025403784439,-0.5,0.));
#36617=DIRECTION('',(1.60246890531964E-16,-1.,0.));
#36618=DIRECTION('',(-0.866025403784439,-0.5,0.));
#36619=DIRECTION('',(-0.866025403784439,0.5,0.));
#36620=DIRECTION('center_axis',(0.,0.,1.));
#36621=DIRECTION('ref_axis',(-0.978821812799614,-0.204714090349635,0.));
#36622=DIRECTION('center_axis',(0.,0.,-1.));
#36623=DIRECTION('ref_axis',(1.,0.,0.));
#36624=DIRECTION('',(0.866025403784438,1.06057523872491E-16,0.5));
#36625=DIRECTION('center_axis',(0.,0.,1.));
#36626=DIRECTION('ref_axis',(1.,0.,0.));
#36627=DIRECTION('center_axis',(-0.5,0.866025403784439,0.));
#36628=DIRECTION('ref_axis',(-0.866025403784439,-0.5,0.));
#36629=DIRECTION('',(0.,0.,1.));
#36630=DIRECTION('',(0.,0.,1.));
#36631=DIRECTION('center_axis',(0.5,0.866025403784439,0.));
#36632=DIRECTION('ref_axis',(-0.866025403784439,0.5,0.));
#36633=DIRECTION('',(0.,0.,1.));
#36634=DIRECTION('center_axis',(1.,-3.20493781063927E-16,0.));
#36635=DIRECTION('ref_axis',(3.20493781063927E-16,1.,0.));
#36636=DIRECTION('',(0.,0.,1.));
#36637=DIRECTION('center_axis',(0.5,-0.866025403784439,0.));
#36638=DIRECTION('ref_axis',(0.866025403784439,0.5,0.));
#36639=DIRECTION('',(0.,0.,1.));
#36640=DIRECTION('center_axis',(-0.5,-0.866025403784439,0.));
#36641=DIRECTION('ref_axis',(0.866025403784439,-0.5,0.));
#36642=DIRECTION('',(0.,0.,1.));
#36643=DIRECTION('center_axis',(-1.,-1.60246890531964E-16,0.));
#36644=DIRECTION('ref_axis',(1.60246890531964E-16,-1.,0.));
#36645=DIRECTION('center_axis',(0.,0.,1.));
#36646=DIRECTION('ref_axis',(1.,0.,0.));
#36647=DIRECTION('center_axis',(0.,0.,-1.));
#36648=DIRECTION('ref_axis',(-1.,0.,0.));
#36649=DIRECTION('center_axis',(0.,0.,1.));
#36650=DIRECTION('ref_axis',(1.,0.,0.));
#36651=DIRECTION('center_axis',(0.,0.,1.));
#36652=DIRECTION('ref_axis',(1.,0.,0.));
#36653=DIRECTION('',(0.707106781186549,8.65956056235495E-17,-0.707106781186546));
#59077=CARTESIAN_POINT('',(0.,0.,0.));
#59078=CARTESIAN_POINT('Origin',(0.,0.,-5.925));
#59079=CARTESIAN_POINT('',(-0.792288171380763,0.000226347567109431,-11.8446668491763));
#59080=CARTESIAN_POINT('',(-0.791102747452279,4.01306674567125E-6,-11.8731331508237));
#59081=CARTESIAN_POINT('',(-0.7911,-9.68818082805471E-17,-5.925));
#59082=CARTESIAN_POINT('',(0.342278108299983,0.713534253311202,-11.9089));
#59083=CARTESIAN_POINT('Ctrl Pts',(-0.7911,-5.38458166943201E-15,-11.8446668491763));
#59084=CARTESIAN_POINT('Ctrl Pts',(-0.791100000000001,0.220167589666669,
-11.8535255927496));
#59085=CARTESIAN_POINT('Ctrl Pts',(-0.694214576672377,0.438610418338673,
-11.8623843363228));
#59086=CARTESIAN_POINT('Ctrl Pts',(-0.531017389080339,0.586395551223148,
-11.8712430798961));
#59087=CARTESIAN_POINT('Ctrl Pts',(-0.367820201488301,0.734180684107624,
-11.8801018234694));
#59088=CARTESIAN_POINT('Ctrl Pts',(-0.140868175871764,0.808992666571332,
-11.8889605670427));
#59089=CARTESIAN_POINT('Ctrl Pts',(0.0782205473247431,0.787223447298299,
-11.8978193106159));
#59090=CARTESIAN_POINT('Ctrl Pts',(0.169567364519674,0.778146992497718,
-11.901512873744));
#59091=CARTESIAN_POINT('Ctrl Pts',(0.259296389908129,0.753014751000273,
-11.905206436872));
#59092=CARTESIAN_POINT('Ctrl Pts',(0.342067962509849,0.713322310757459,
-11.9089));
#59093=CARTESIAN_POINT('',(-0.342067962509551,0.713322310757602,-11.9089));
#59094=CARTESIAN_POINT('Origin',(0.,0.,-11.9089));
#59095=CARTESIAN_POINT('Ctrl Pts',(-0.34206796250955,0.713322310757602,
-11.9089));
#59096=CARTESIAN_POINT('Ctrl Pts',(-0.46073916563555,0.656414492160488,
-11.9036044671685));
#59097=CARTESIAN_POINT('Ctrl Pts',(-0.564730701364708,0.569550653783437,
-11.8983089343371));
#59098=CARTESIAN_POINT('Ctrl Pts',(-0.641730011423605,0.462747660298155,
-11.8930134015056));
#59099=CARTESIAN_POINT('Ctrl Pts',(-0.718729321482501,0.355944666812873,
-11.8877178686741));
#59100=CARTESIAN_POINT('Ctrl Pts',(-0.768736405871138,0.229202518219359,
-11.8824223358427));
#59101=CARTESIAN_POINT('Ctrl Pts',(-0.785095797833949,0.0988017982372159,
-11.8771268030112));
#59102=CARTESIAN_POINT('Ctrl Pts',(-0.789208303196394,0.0660210163223179,
-11.8757955856154));
#59103=CARTESIAN_POINT('Ctrl Pts',(-0.791194462610664,0.0330090331603962,
-11.8744643682195));
#59104=CARTESIAN_POINT('Ctrl Pts',(-0.791102747452279,4.01306674567134E-6,
-11.8731331508237));
#59105=CARTESIAN_POINT('Origin',(0.,0.,-5.925));
#59106=CARTESIAN_POINT('',(-0.790012975131354,0.0005491902118549,-11.6446668491763));
#59107=CARTESIAN_POINT('',(-0.79040343262036,8.06582135657781E-6,-11.6731331508237));
#59108=CARTESIAN_POINT('',(-0.7911,-9.68818082805471E-17,-5.925));
#59109=CARTESIAN_POINT('Ctrl Pts',(-0.790012975131354,0.0005491902118549,
-11.6446668491763));
#59110=CARTESIAN_POINT('Ctrl Pts',(-0.790590861888083,0.105013430132942,
-11.6488501997533));
#59111=CARTESIAN_POINT('Ctrl Pts',(-0.771472741075023,0.209260755864815,
-11.6530335503304));
#59112=CARTESIAN_POINT('Ctrl Pts',(-0.731721227296555,0.304762699534902,
-11.6572169009074));
#59113=CARTESIAN_POINT('Ctrl Pts',(-0.63108158811855,0.546546728322295,
-11.6678079665704));
#59114=CARTESIAN_POINT('Ctrl Pts',(-0.398190192648554,0.732276372886272,
-11.6783990322333));
#59115=CARTESIAN_POINT('Ctrl Pts',(-0.140344232552206,0.779437657881449,
-11.6889900978962));
#59116=CARTESIAN_POINT('Ctrl Pts',(-0.0114212525040319,0.803018300379038,
-11.6942856307277));
#59117=CARTESIAN_POINT('Ctrl Pts',(0.12374036870073,0.791956852984427,-11.6995811635591));
#59118=CARTESIAN_POINT('Ctrl Pts',(0.249075376653612,0.750270516544755,
-11.7048766963906));
#59119=CARTESIAN_POINT('Ctrl Pts',(0.374410384606493,0.708584180105084,
-11.7101722292221));
#59120=CARTESIAN_POINT('Ctrl Pts',(0.489918779307494,0.636272954620351,
-11.7154677620535));
#59121=CARTESIAN_POINT('Ctrl Pts',(0.579225354855548,0.540248340915313,
-11.720763294885));
#59122=CARTESIAN_POINT('Ctrl Pts',(0.757838505951657,0.348199113505236,
-11.7313543605479));
#59123=CARTESIAN_POINT('Ctrl Pts',(0.831644380435981,0.0612963332139369,
-11.7419454262109));
#59124=CARTESIAN_POINT('Ctrl Pts',(0.768045306521618,-0.193562270365957,
-11.7525364918738));
#59125=CARTESIAN_POINT('Ctrl Pts',(0.736245769564436,-0.320991572155904,
-11.7578320247052));
#59126=CARTESIAN_POINT('Ctrl Pts',(0.670094995507583,-0.440409829767999,
-11.7631275575367));
#59127=CARTESIAN_POINT('Ctrl Pts',(0.580367540765873,-0.537139674991059,
-11.7684230903682));
#59128=CARTESIAN_POINT('Ctrl Pts',(0.490640086024162,-0.633869520214118,
-11.7737186231996));
#59129=CARTESIAN_POINT('Ctrl Pts',(0.377335950597594,-0.707910953048141,
-11.7790141560311));
#59130=CARTESIAN_POINT('Ctrl Pts',(0.253024067411846,-0.749801060819932,
-11.7843096888626));
#59131=CARTESIAN_POINT('Ctrl Pts',(0.128712184226097,-0.791691168591722,
-11.789605221694));
#59132=CARTESIAN_POINT('Ctrl Pts',(-0.00660744671883115,-0.801429951301279,
-11.7949007545255));
#59133=CARTESIAN_POINT('Ctrl Pts',(-0.136544532071595,-0.778895785431844,
-11.800196287357));
#59134=CARTESIAN_POINT('Ctrl Pts',(-0.266481617424357,-0.756361619562409,
-11.8054918201884));
#59135=CARTESIAN_POINT('Ctrl Pts',(-0.391036157184956,-0.701554505113982,
-11.8107873530199));
#59136=CARTESIAN_POINT('Ctrl Pts',(-0.49348933853164,-0.619414227979409,
-11.8160828858514));
#59137=CARTESIAN_POINT('Ctrl Pts',(-0.677828231414856,-0.471623329257867,
-11.8256108736263));
#59138=CARTESIAN_POINT('Ctrl Pts',(-0.790618379347089,-0.235346761505971,
-11.8351388614013));
#59139=CARTESIAN_POINT('Ctrl Pts',(-0.792288171380763,0.000226347567109431,
-11.8446668491763));
#59140=CARTESIAN_POINT('Ctrl Pts',(-0.791102747452279,4.01306674567134E-6,
-11.8731331508237));
#59141=CARTESIAN_POINT('Ctrl Pts',(-0.790829623153274,-0.0982836978797118,
-11.8691688353881));
#59142=CARTESIAN_POINT('Ctrl Pts',(-0.772129365994563,-0.19650965852332,
-11.8652045199524));
#59143=CARTESIAN_POINT('Ctrl Pts',(-0.736282073336785,-0.288384104892399,
-11.8612402045168));
#59144=CARTESIAN_POINT('Ctrl Pts',(-0.688397257339822,-0.411109996669098,
-11.8559446716854));
#59145=CARTESIAN_POINT('Ctrl Pts',(-0.60991592580891,-0.522502488851721,
-11.8506491388539));
#59146=CARTESIAN_POINT('Ctrl Pts',(-0.509058409110686,-0.606702005847251,
-11.8453536060224));
#59147=CARTESIAN_POINT('Ctrl Pts',(-0.307343375714237,-0.77510103983831,
-11.8347625403595));
#59148=CARTESIAN_POINT('Ctrl Pts',(-0.0161236016485408,-0.834728173080993,
-11.8241714746966));
#59149=CARTESIAN_POINT('Ctrl Pts',(0.233939335027844,-0.757220177092663,
-11.8135804090336));
#59150=CARTESIAN_POINT('Ctrl Pts',(0.484002271704228,-0.679712181104333,
-11.8029893433707));
#59151=CARTESIAN_POINT('Ctrl Pts',(0.692908370991301,-0.465069055884989,
-11.7923982777078));
#59152=CARTESIAN_POINT('Ctrl Pts',(0.763430372307437,-0.212979240313773,
-11.7818072120449));
#59153=CARTESIAN_POINT('Ctrl Pts',(0.833952373623573,0.0391105752574421,
-11.7712161463819));
#59154=CARTESIAN_POINT('Ctrl Pts',(0.766090276968773,0.328647081180532,
-11.760625080719));
#59155=CARTESIAN_POINT('Ctrl Pts',(0.592385804055834,0.525627978917452,
-11.7500340150561));
#59156=CARTESIAN_POINT('Ctrl Pts',(0.505533567599364,0.624118427785913,
-11.7447384822246));
#59157=CARTESIAN_POINT('Ctrl Pts',(0.39222073707836,0.699469974607832,-11.7394429493931));
#59158=CARTESIAN_POINT('Ctrl Pts',(0.268071565851031,0.743949386305491,
-11.7341474165617));
#59159=CARTESIAN_POINT('Ctrl Pts',(0.143922394623702,0.788428798003151,
-11.7288518837302));
#59160=CARTESIAN_POINT('Ctrl Pts',(0.0089368826900479,0.802036074576551,
-11.7235563508987));
#59161=CARTESIAN_POINT('Ctrl Pts',(-0.120716544232802,0.7820807665739,-11.7182608180673));
#59162=CARTESIAN_POINT('Ctrl Pts',(-0.250369971155652,0.762125458571248,
-11.7129652852358));
#59163=CARTESIAN_POINT('Ctrl Pts',(-0.374691313067697,0.708607565992544,
-11.7076697524044));
#59164=CARTESIAN_POINT('Ctrl Pts',(-0.479675261807679,0.628694803568363,
-11.7023742195729));
#59165=CARTESIAN_POINT('Ctrl Pts',(-0.58465921054766,0.548782041144181,
-11.6970786867414));
#59166=CARTESIAN_POINT('Ctrl Pts',(-0.670305766115577,0.442474408874522,
-11.69178315391));
#59167=CARTESIAN_POINT('Ctrl Pts',(-0.723483356181124,0.322384519957157,
-11.6864876210785));
#59168=CARTESIAN_POINT('Ctrl Pts',(-0.768185092994327,0.221435481053854,
-11.6820361309935));
#59169=CARTESIAN_POINT('Ctrl Pts',(-0.789943315386619,0.110747499155085,
-11.6775846409086));
#59170=CARTESIAN_POINT('Ctrl Pts',(-0.789527040486882,1.82139033282201E-5,
-11.6731331508237));
#59171=CARTESIAN_POINT('Origin',(0.,0.,-5.925));
#59172=CARTESIAN_POINT('',(-0.790545294603651,-0.000683398138164537,-11.4446668491763));
#59173=CARTESIAN_POINT('',(-0.7911,-5.52280443599784E-13,-11.4731331508237));
#59174=CARTESIAN_POINT('',(-0.7911,-9.68818082805471E-17,-5.925));
#59175=CARTESIAN_POINT('Ctrl Pts',(-0.790545294603651,-0.000683398138164537,
-11.4446668491763));
#59176=CARTESIAN_POINT('Ctrl Pts',(-0.788780870289845,0.180895070368877,
-11.4519704724424));
#59177=CARTESIAN_POINT('Ctrl Pts',(-0.726011118514491,0.36333336139957,
-11.4592740957086));
#59178=CARTESIAN_POINT('Ctrl Pts',(-0.611539636809332,0.503228087254033,
-11.4665777189747));
#59179=CARTESIAN_POINT('Ctrl Pts',(-0.528541449807152,0.604659539386308,
-11.4718732518062));
#59180=CARTESIAN_POINT('Ctrl Pts',(-0.418363373867963,0.68372560107528,
-11.4771687846376));
#59181=CARTESIAN_POINT('Ctrl Pts',(-0.295847636573397,0.733088687506037,
-11.4824643174691));
#59182=CARTESIAN_POINT('Ctrl Pts',(-0.173331899278832,0.782451773936795,
-11.4877598503006));
#59183=CARTESIAN_POINT('Ctrl Pts',(-0.0384785006288894,0.802111885109338,
-11.493055383132));
#59184=CARTESIAN_POINT('Ctrl Pts',(0.0917517255541586,0.786735608339574,
-11.4983509159635));
#59185=CARTESIAN_POINT('Ctrl Pts',(0.352212177920255,0.755983054800047,
-11.5089419816264));
#59186=CARTESIAN_POINT('Ctrl Pts',(0.594179940418773,0.585084949491291,
-11.5195330472894));
#59187=CARTESIAN_POINT('Ctrl Pts',(0.710697704171871,0.349664281229984,
-11.5301241129523));
#59188=CARTESIAN_POINT('Ctrl Pts',(0.76895658604842,0.231953947099331,-11.5354196457837));
#59189=CARTESIAN_POINT('Ctrl Pts',(0.795852968238614,0.0981129722305401,
-11.5407151786152));
#59190=CARTESIAN_POINT('Ctrl Pts',(0.790075348975073,-0.0336997945528526,
-11.5460107114467));
#59191=CARTESIAN_POINT('Ctrl Pts',(0.784297729711532,-0.165512561336244,
-11.5513062442781));
#59192=CARTESIAN_POINT('Ctrl Pts',(0.745846108994256,-0.295297120034238,
-11.5566017771096));
#59193=CARTESIAN_POINT('Ctrl Pts',(0.67822489890413,-0.407697544259937,
-11.5618973099411));
#59194=CARTESIAN_POINT('Ctrl Pts',(0.610603688814002,-0.520097968485637,
-11.5671928427725));
#59195=CARTESIAN_POINT('Ctrl Pts',(0.513812889351022,-0.615114258239043,
-11.572488375604));
#59196=CARTESIAN_POINT('Ctrl Pts',(0.400176763834465,-0.682055607413933,
-11.5777839084355));
#59197=CARTESIAN_POINT('Ctrl Pts',(0.286540638317908,-0.748996956588823,
-11.5830794412669));
#59198=CARTESIAN_POINT('Ctrl Pts',(0.156059186747776,-0.787863365185198,
-11.5883749740984));
#59199=CARTESIAN_POINT('Ctrl Pts',(0.0247893579774138,-0.791581102442525,
-11.5936705069299));
#59200=CARTESIAN_POINT('Ctrl Pts',(-0.237750299563309,-0.799016576957179,
-11.6042615725928));
#59201=CARTESIAN_POINT('Ctrl Pts',(-0.50344346590495,-0.665857366115643,
-11.6148526382557));
#59202=CARTESIAN_POINT('Ctrl Pts',(-0.652096107632763,-0.450358554189471,
-11.6254437039186));
#59203=CARTESIAN_POINT('Ctrl Pts',(-0.742032645208044,-0.319979323985716,
-11.6318514190045));
#59204=CARTESIAN_POINT('Ctrl Pts',(-0.789127815348344,-0.159460609050876,
-11.6382591340904));
#59205=CARTESIAN_POINT('Ctrl Pts',(-0.790012975131354,0.0005491902118549,
-11.6446668491763));
#59206=CARTESIAN_POINT('Ctrl Pts',(-0.7911,-5.48172618408671E-13,-11.6731331508237));
#59207=CARTESIAN_POINT('Ctrl Pts',(-0.791099999999848,-0.220167589667223,
-11.6642744072504));
#59208=CARTESIAN_POINT('Ctrl Pts',(-0.69421457667207,-0.43861041833916,
-11.6554156636771));
#59209=CARTESIAN_POINT('Ctrl Pts',(-0.531017389079927,-0.586395551223521,
-11.6465569201039));
#59210=CARTESIAN_POINT('Ctrl Pts',(-0.367820201487785,-0.734180684107883,
-11.6376981765306));
#59211=CARTESIAN_POINT('Ctrl Pts',(-0.140868175871194,-0.808992666571432,
-11.6288394329573));
#59212=CARTESIAN_POINT('Ctrl Pts',(0.0782205473252975,-0.787223447298244,
-11.619980689384));
#59213=CARTESIAN_POINT('Ctrl Pts',(0.297309270521789,-0.765454228025056,
-11.6111219458108));
#59214=CARTESIAN_POINT('Ctrl Pts',(0.505102072676036,-0.647444880833887,
-11.6022632022375));
#59215=CARTESIAN_POINT('Ctrl Pts',(0.636026795762051,-0.470435038100542,
-11.5934044586642));
#59216=CARTESIAN_POINT('Ctrl Pts',(0.766951518848066,-0.293425195367197,
-11.5845457150909));
#59217=CARTESIAN_POINT('Ctrl Pts',(0.818956872247111,-0.0601881960093751,
-11.5756869715177));
#59218=CARTESIAN_POINT('Ctrl Pts',(0.775631781004105,0.155674501111777,
-11.5668282279444));
#59219=CARTESIAN_POINT('Ctrl Pts',(0.732306689761099,0.37153719823293,-11.5579694843711));
#59220=CARTESIAN_POINT('Ctrl Pts',(0.594329958849832,0.566643518936898,
-11.5491107407979));
#59221=CARTESIAN_POINT('Ctrl Pts',(0.405242230243583,0.679424716085018,
-11.5402519972246));
#59222=CARTESIAN_POINT('Ctrl Pts',(0.216154501637335,0.792205913233137,
-11.5313932536513));
#59223=CARTESIAN_POINT('Ctrl Pts',(-0.021081652930565,0.820894963712988,
-11.522534510078));
#59224=CARTESIAN_POINT('Ctrl Pts',(-0.231602780753722,0.756438604215269,
-11.5136757665048));
#59225=CARTESIAN_POINT('Ctrl Pts',(-0.442123908576878,0.691982244717549,
-11.5048170229315));
#59226=CARTESIAN_POINT('Ctrl Pts',(-0.622631625634527,0.535390358803125,
-11.4959582793582));
#59227=CARTESIAN_POINT('Ctrl Pts',(-0.716163994722375,0.336077881841828,
-11.487099535785));
#59228=CARTESIAN_POINT('Ctrl Pts',(-0.765317280859639,0.231334857514026,
-11.4824440741312));
#59229=CARTESIAN_POINT('Ctrl Pts',(-0.791100000000078,0.115702837835999,
-11.4777886124774));
#59230=CARTESIAN_POINT('Ctrl Pts',(-0.7911,-5.29742916199893E-13,-11.4731331508237));
#59231=CARTESIAN_POINT('Origin',(0.,0.,-5.925));
#59232=CARTESIAN_POINT('',(-0.791998230343716,8.528260225521E-5,-11.2446668491763));
#59233=CARTESIAN_POINT('',(-0.7911,-5.52058398994859E-13,-11.2731331508237));
#59234=CARTESIAN_POINT('',(-0.7911,-9.68818082805471E-17,-5.925));
#59235=CARTESIAN_POINT('Ctrl Pts',(-0.791998230343716,8.528260225521E-5,
-11.2446668491763));
#59236=CARTESIAN_POINT('Ctrl Pts',(-0.792178295342062,0.127006680560579,
-11.2497952123001));
#59237=CARTESIAN_POINT('Ctrl Pts',(-0.759545080480787,0.253992239431632,
-11.2549235754238));
#59238=CARTESIAN_POINT('Ctrl Pts',(-0.700059092435406,0.367235780460078,
-11.2600519385476));
#59239=CARTESIAN_POINT('Ctrl Pts',(-0.638634034360461,0.484170731241736,
-11.265347471379));
#59240=CARTESIAN_POINT('Ctrl Pts',(-0.548577025685627,0.586453162772788,
-11.2706430042105));
#59241=CARTESIAN_POINT('Ctrl Pts',(-0.439362873703711,0.659038358226858,
-11.275938537042));
#59242=CARTESIAN_POINT('Ctrl Pts',(-0.22093456973988,0.804208749134998,
-11.2865296027049));
#59243=CARTESIAN_POINT('Ctrl Pts',(0.0741223074522833,0.830590195735207,
-11.2971206683678));
#59244=CARTESIAN_POINT('Ctrl Pts',(0.315331238093299,0.726582783969357,
-11.3077117340308));
#59245=CARTESIAN_POINT('Ctrl Pts',(0.435935703413807,0.674579078086432,
-11.3130072668622));
#59246=CARTESIAN_POINT('Ctrl Pts',(0.543078182096528,0.589978157611991,
-11.3183027996937));
#59247=CARTESIAN_POINT('Ctrl Pts',(0.624003832575897,0.48577151940361,-11.3235983325252));
#59248=CARTESIAN_POINT('Ctrl Pts',(0.704929483055266,0.381564881195229,
-11.3288938653566));
#59249=CARTESIAN_POINT('Ctrl Pts',(0.759638305331283,0.257752525252907,
-11.3341893981881));
#59250=CARTESIAN_POINT('Ctrl Pts',(0.78086075150283,0.128307203301138,-11.3394849310195));
#59251=CARTESIAN_POINT('Ctrl Pts',(0.802083197674377,-0.00113811865063054,
-11.344780463851));
#59252=CARTESIAN_POINT('Ctrl Pts',(0.789819267741456,-0.136216406611844,
-11.3500759966825));
#59253=CARTESIAN_POINT('Ctrl Pts',(0.746541473664785,-0.260801113101208,
-11.3553715295139));
#59254=CARTESIAN_POINT('Ctrl Pts',(0.703263679588115,-0.385385819590573,
-11.3606670623454));
#59255=CARTESIAN_POINT('Ctrl Pts',(0.628972021367694,-0.499476944608087,
-11.3659625951769));
#59256=CARTESIAN_POINT('Ctrl Pts',(0.531326032698895,-0.587288413821764,
-11.3712581280083));
#59257=CARTESIAN_POINT('Ctrl Pts',(0.336034055361296,-0.762911352249118,
-11.3818491936713));
#59258=CARTESIAN_POINT('Ctrl Pts',(0.0473247562301771,-0.833415667461127,
-11.3924402593342));
#59259=CARTESIAN_POINT('Ctrl Pts',(-0.205480744072948,-0.765395119469284,
-11.4030313249971));
#59260=CARTESIAN_POINT('Ctrl Pts',(-0.458286244376074,-0.697374571477442,
-11.41362239066));
#59261=CARTESIAN_POINT('Ctrl Pts',(-0.675187945851208,-0.490829160281748,
-11.424213456323));
#59262=CARTESIAN_POINT('Ctrl Pts',(-0.755000387460612,-0.241394221665018,
-11.4348045219859));
#59263=CARTESIAN_POINT('Ctrl Pts',(-0.779773985575188,-0.163970191019942,
-11.4380919643827));
#59264=CARTESIAN_POINT('Ctrl Pts',(-0.791339481691865,-0.0824138946279092,
-11.4413794067795));
#59265=CARTESIAN_POINT('Ctrl Pts',(-0.790545294603651,-0.000683398138164537,
-11.4446668491763));
#59266=CARTESIAN_POINT('Ctrl Pts',(-0.7911,-5.29742916199893E-13,-11.4731331508237));
#59267=CARTESIAN_POINT('Ctrl Pts',(-0.791099999999853,-0.220167589667203,
-11.4642744072504));
#59268=CARTESIAN_POINT('Ctrl Pts',(-0.694214576672081,-0.438610418339141,
-11.4554156636771));
#59269=CARTESIAN_POINT('Ctrl Pts',(-0.531017389079944,-0.586395551223506,
-11.4465569201039));
#59270=CARTESIAN_POINT('Ctrl Pts',(-0.367820201487807,-0.734180684107871,
-11.4376981765306));
#59271=CARTESIAN_POINT('Ctrl Pts',(-0.140868175871221,-0.808992666571427,
-11.4288394329573));
#59272=CARTESIAN_POINT('Ctrl Pts',(0.0782205473252707,-0.787223447298247,
-11.419980689384));
#59273=CARTESIAN_POINT('Ctrl Pts',(0.297309270521762,-0.765454228025067,
-11.4111219458108));
#59274=CARTESIAN_POINT('Ctrl Pts',(0.505102072676012,-0.647444880833905,
-11.4022632022375));
#59275=CARTESIAN_POINT('Ctrl Pts',(0.636026795762033,-0.470435038100567,
-11.3934044586642));
#59276=CARTESIAN_POINT('Ctrl Pts',(0.766951518848054,-0.293425195367228,
-11.3845457150909));
#59277=CARTESIAN_POINT('Ctrl Pts',(0.818956872247108,-0.0601881960094103,
-11.3756869715177));
#59278=CARTESIAN_POINT('Ctrl Pts',(0.775631781004112,0.155674501111743,
-11.3668282279444));
#59279=CARTESIAN_POINT('Ctrl Pts',(0.732306689761116,0.371537198232896,
-11.3579694843711));
#59280=CARTESIAN_POINT('Ctrl Pts',(0.594329958849859,0.566643518936869,
-11.3491107407979));
#59281=CARTESIAN_POINT('Ctrl Pts',(0.405242230243617,0.679424716084997,
-11.3402519972246));
#59282=CARTESIAN_POINT('Ctrl Pts',(0.216154501637376,0.792205913233126,
-11.3313932536513));
#59283=CARTESIAN_POINT('Ctrl Pts',(-0.021081652930521,0.820894963712989,
-11.322534510078));
#59284=CARTESIAN_POINT('Ctrl Pts',(-0.23160278075368,0.756438604215281,
-11.3136757665048));
#59285=CARTESIAN_POINT('Ctrl Pts',(-0.442123908576839,0.691982244717574,
-11.3048170229315));
#59286=CARTESIAN_POINT('Ctrl Pts',(-0.622631625634495,0.535390358803162,
-11.2959582793582));
#59287=CARTESIAN_POINT('Ctrl Pts',(-0.716163994722355,0.336077881841871,
-11.287099535785));
#59288=CARTESIAN_POINT('Ctrl Pts',(-0.765317280859636,0.23133485751405,
-11.2824440741312));
#59289=CARTESIAN_POINT('Ctrl Pts',(-0.791100000000082,0.115702837835997,
-11.2777886124774));
#59290=CARTESIAN_POINT('Ctrl Pts',(-0.7911,-5.57609514117985E-13,-11.2731331508237));
#59291=CARTESIAN_POINT('Origin',(0.,0.,-5.925));
#59292=CARTESIAN_POINT('',(-0.7911,2.07056594092592E-14,-11.0446668491763));
#59293=CARTESIAN_POINT('',(-0.791256742313348,0.000223351368557853,-11.0731331508237));
#59294=CARTESIAN_POINT('',(-0.7911,-9.68818082805471E-17,-5.925));
#59295=CARTESIAN_POINT('Ctrl Pts',(-0.791038879775141,0.000560250703841913,
-11.0446668491763));
#59296=CARTESIAN_POINT('Ctrl Pts',(-0.791423651940124,0.0741512003445719,
-11.0476199521577));
#59297=CARTESIAN_POINT('Ctrl Pts',(-0.78172570506452,0.14761201439333,-11.0505730551391));
#59298=CARTESIAN_POINT('Ctrl Pts',(-0.761508425370342,0.217890363424224,
-11.0535261581205));
#59299=CARTESIAN_POINT('Ctrl Pts',(-0.689000782353362,0.469937993987601,
-11.0641172237834));
#59300=CARTESIAN_POINT('Ctrl Pts',(-0.481189233708814,0.681051474651298,
-11.0747082894463));
#59301=CARTESIAN_POINT('Ctrl Pts',(-0.230012551894391,0.757925166261443,
-11.0852993551093));
#59302=CARTESIAN_POINT('Ctrl Pts',(-0.104424210987177,0.796362012066516,
-11.0905948879407));
#59303=CARTESIAN_POINT('Ctrl Pts',(0.0320054132125054,0.8012389106082,-11.0958904207722));
#59304=CARTESIAN_POINT('Ctrl Pts',(0.161144620509277,0.774200983873756,
-11.1011859536036));
#59305=CARTESIAN_POINT('Ctrl Pts',(0.290283827806048,0.747163057139313,
-11.1064814864351));
#59306=CARTESIAN_POINT('Ctrl Pts',(0.412132618199907,0.688210305128744,
-11.1117770192666));
#59307=CARTESIAN_POINT('Ctrl Pts',(0.512104914632304,0.603286671475527,
-11.117072552098));
#59308=CARTESIAN_POINT('Ctrl Pts',(0.612077211064701,0.51836303782231,-11.1223680849295));
#59309=CARTESIAN_POINT('Ctrl Pts',(0.690173013535636,0.407468522526445,
-11.127663617761));
#59310=CARTESIAN_POINT('Ctrl Pts',(0.737837287880873,0.284495218519558,
-11.1329591505924));
#59311=CARTESIAN_POINT('Ctrl Pts',(0.785501562226111,0.161521914512671,
-11.1382546834239));
#59312=CARTESIAN_POINT('Ctrl Pts',(0.802734308445651,0.0264698217947621,
-11.1435502162554));
#59313=CARTESIAN_POINT('Ctrl Pts',(0.785154399946323,-0.103670640969592,
-11.1488457490868));
#59314=CARTESIAN_POINT('Ctrl Pts',(0.749994582947666,-0.363951566498299,
-11.1594368147498));
#59315=CARTESIAN_POINT('Ctrl Pts',(0.575584147073533,-0.604585972212789,
-11.1700278804127));
#59316=CARTESIAN_POINT('Ctrl Pts',(0.338864849532643,-0.716395588408117,
-11.1806189460756));
#59317=CARTESIAN_POINT('Ctrl Pts',(0.102145551991752,-0.828205204603444,
-11.1912100117385));
#59318=CARTESIAN_POINT('Ctrl Pts',(-0.196882607215897,-0.811190031279611,
-11.2018010774015));
#59319=CARTESIAN_POINT('Ctrl Pts',(-0.419187228122118,-0.672739789110212,
-11.2123921430644));
#59320=CARTESIAN_POINT('Ctrl Pts',(-0.641491849028339,-0.534289546940814,
-11.2229832087273));
#59321=CARTESIAN_POINT('Ctrl Pts',(-0.787072931633131,-0.274404235925851,
-11.2335742743902));
#59322=CARTESIAN_POINT('Ctrl Pts',(-0.791875815867984,-0.0123258388778453,
-11.2441653400532));
#59323=CARTESIAN_POINT('Ctrl Pts',(-0.791951624741163,-0.00818918536021873,
-11.2443325097609));
#59324=CARTESIAN_POINT('Ctrl Pts',(-0.79199236074899,-0.00405198546671845,
-11.2444996794686));
#59325=CARTESIAN_POINT('Ctrl Pts',(-0.791998230343716,8.528260225521E-5,
-11.2446668491763));
#59326=CARTESIAN_POINT('Ctrl Pts',(-0.791333191223927,-2.41016881485458E-5,
-11.2731331508237));
#59327=CARTESIAN_POINT('Ctrl Pts',(-0.791326629821211,-0.128692147081735,
-11.2679385877924));
#59328=CARTESIAN_POINT('Ctrl Pts',(-0.75873374763038,-0.257269522733714,
-11.2627440247611));
#59329=CARTESIAN_POINT('Ctrl Pts',(-0.698053215585031,-0.371586410333449,
-11.2575494617299));
#59330=CARTESIAN_POINT('Ctrl Pts',(-0.636193200076023,-0.48812534302732,
-11.2522539288984));
#59331=CARTESIAN_POINT('Ctrl Pts',(-0.545143010043687,-0.589844020655748,
-11.2469583960669));
#59332=CARTESIAN_POINT('Ctrl Pts',(-0.435241086870445,-0.661756396250121,
-11.2416628632355));
#59333=CARTESIAN_POINT('Ctrl Pts',(-0.215437240523961,-0.805581147438867,
-11.2310717975725));
#59334=CARTESIAN_POINT('Ctrl Pts',(0.0797735383861531,-0.8301806904914,
-11.2204807319096));
#59335=CARTESIAN_POINT('Ctrl Pts',(0.31985801956751,-0.724611716522641,
-11.2098896662467));
#59336=CARTESIAN_POINT('Ctrl Pts',(0.439900260158188,-0.671827229538261,
-11.2045941334152));
#59337=CARTESIAN_POINT('Ctrl Pts',(0.546160926316679,-0.586500613298557,
-11.1992986005838));
#59338=CARTESIAN_POINT('Ctrl Pts',(0.626725961646807,-0.481829243974973,
-11.1940030677523));
#59339=CARTESIAN_POINT('Ctrl Pts',(0.707290996976935,-0.377157874651387,
-11.1887075349208));
#59340=CARTESIAN_POINT('Ctrl Pts',(0.762160401478703,-0.25314175224392,
-11.1834120020894));
#59341=CARTESIAN_POINT('Ctrl Pts',(0.782262440283046,-0.123631341427009,
-11.1781164692579));
#59342=CARTESIAN_POINT('Ctrl Pts',(0.822466517891732,0.135389480206813,
-11.167525403595));
#59343=CARTESIAN_POINT('Ctrl Pts',(0.723601132710717,0.416387455478408,
-11.156934337932));
#59344=CARTESIAN_POINT('Ctrl Pts',(0.528327196544448,0.590903654976208,
-11.1463432722691));
#59345=CARTESIAN_POINT('Ctrl Pts',(0.33305326037818,0.765419854474006,-11.1357522066062));
#59346=CARTESIAN_POINT('Ctrl Pts',(0.0413707732266558,0.833454278198008,
-11.1251611409433));
#59347=CARTESIAN_POINT('Ctrl Pts',(-0.211013810741115,0.763888209763645,
-11.1145700752803));
#59348=CARTESIAN_POINT('Ctrl Pts',(-0.463398394708886,0.694322141329282,
-11.1039790096174));
#59349=CARTESIAN_POINT('Ctrl Pts',(-0.676485075492905,0.487155580736554,
-11.0933879439545));
#59350=CARTESIAN_POINT('Ctrl Pts',(-0.755751859692147,0.236757597821015,
-11.0827968782915));
#59351=CARTESIAN_POINT('Ctrl Pts',(-0.779860626588515,0.160599763711617,
-11.0795756358022));
#59352=CARTESIAN_POINT('Ctrl Pts',(-0.791590318129958,0.0804427856162157,
-11.076354393313));
#59353=CARTESIAN_POINT('Ctrl Pts',(-0.791256742313348,0.000223351368557853,
-11.0731331508237));
#59354=CARTESIAN_POINT('Origin',(0.,0.,-5.925));
#59355=CARTESIAN_POINT('',(-0.7911,3.99680288865056E-15,-10.8446668491763));
#59356=CARTESIAN_POINT('',(-0.789614839096957,4.0911287493315E-5,-10.8731331508237));
#59357=CARTESIAN_POINT('',(-0.7911,-9.68818082805471E-17,-5.925));
#59358=CARTESIAN_POINT('Ctrl Pts',(-0.7911,-7.21644966006352E-15,-10.8446668491763));
#59359=CARTESIAN_POINT('Ctrl Pts',(-0.791100000000002,0.220167589666667,
-10.8535255927496));
#59360=CARTESIAN_POINT('Ctrl Pts',(-0.694214576672378,0.438610418338671,
-10.8623843363228));
#59361=CARTESIAN_POINT('Ctrl Pts',(-0.53101738908034,0.586395551223147,
-10.8712430798961));
#59362=CARTESIAN_POINT('Ctrl Pts',(-0.367820201488302,0.734180684107623,
-10.8801018234694));
#59363=CARTESIAN_POINT('Ctrl Pts',(-0.140868175871765,0.808992666571332,
-10.8889605670427));
#59364=CARTESIAN_POINT('Ctrl Pts',(0.0782205473247419,0.787223447298299,
-10.8978193106159));
#59365=CARTESIAN_POINT('Ctrl Pts',(0.297309270521249,0.765454228025266,
-10.9066780541892));
#59366=CARTESIAN_POINT('Ctrl Pts',(0.505102072675578,0.647444880834243,
-10.9155367977625));
#59367=CARTESIAN_POINT('Ctrl Pts',(0.636026795761718,0.470435038100992,
-10.9243955413357));
#59368=CARTESIAN_POINT('Ctrl Pts',(0.766951518847858,0.29342519536774,-10.933254284909));
#59369=CARTESIAN_POINT('Ctrl Pts',(0.818956872247068,0.0601881960099554,
-10.9421130284823));
#59370=CARTESIAN_POINT('Ctrl Pts',(0.775631781004215,-0.155674501111227,
-10.9509717720556));
#59371=CARTESIAN_POINT('Ctrl Pts',(0.732306689761362,-0.37153719823241,
-10.9598305156288));
#59372=CARTESIAN_POINT('Ctrl Pts',(0.594329958850234,-0.566643518936476,
-10.9686892592021));
#59373=CARTESIAN_POINT('Ctrl Pts',(0.405242230244066,-0.679424716084729,
-10.9775480027754));
#59374=CARTESIAN_POINT('Ctrl Pts',(0.216154501637899,-0.792205913232983,
-10.9864067463487));
#59375=CARTESIAN_POINT('Ctrl Pts',(-0.0210816529299804,-0.820894963713003,
-10.9952654899219));
#59376=CARTESIAN_POINT('Ctrl Pts',(-0.231602780753183,-0.756438604215434,
-11.0041242334952));
#59377=CARTESIAN_POINT('Ctrl Pts',(-0.442123908576385,-0.691982244717864,
-11.0129829770685));
#59378=CARTESIAN_POINT('Ctrl Pts',(-0.622631625634145,-0.53539035880357,
-11.0218417206417));
#59379=CARTESIAN_POINT('Ctrl Pts',(-0.716163994722135,-0.336077881842339,
-11.030700464215));
#59380=CARTESIAN_POINT('Ctrl Pts',(-0.765317280859481,-0.231334857514556,
-11.0353559258688));
#59381=CARTESIAN_POINT('Ctrl Pts',(-0.791100000000003,-0.115702837836527,
-11.0400113875225));
#59382=CARTESIAN_POINT('Ctrl Pts',(-0.7911,2.07056594092592E-14,-11.0446668491763));
#59383=CARTESIAN_POINT('Ctrl Pts',(-0.791256742313348,0.000223351368557853,
-11.0731331508237));
#59384=CARTESIAN_POINT('Ctrl Pts',(-0.791041939144359,-0.0514332371274546,
-11.0710588604815));
#59385=CARTESIAN_POINT('Ctrl Pts',(-0.785824980273388,-0.103115723698081,
-11.0689845701393));
#59386=CARTESIAN_POINT('Ctrl Pts',(-0.775690191700812,-0.153772947058482,
-11.0669102797971));
#59387=CARTESIAN_POINT('Ctrl Pts',(-0.749816713656429,-0.283097653441737,
-11.0616147469657));
#59388=CARTESIAN_POINT('Ctrl Pts',(-0.691891339614235,-0.405740219169775,
-11.0563192141342));
#59389=CARTESIAN_POINT('Ctrl Pts',(-0.607960482036218,-0.506547434948466,
-11.0510236813027));
#59390=CARTESIAN_POINT('Ctrl Pts',(-0.524029624458202,-0.607354650727156,
-11.0457281484713));
#59391=CARTESIAN_POINT('Ctrl Pts',(-0.414093283344361,-0.686326516556501,
-11.0404326156398));
#59392=CARTESIAN_POINT('Ctrl Pts',(-0.29150238721463,-0.735106189878946,
-11.0351370828084));
#59393=CARTESIAN_POINT('Ctrl Pts',(-0.1689114910849,-0.783885863201392,
-11.0298415499769));
#59394=CARTESIAN_POINT('Ctrl Pts',(-0.0336660399392779,-0.80247334401694,
-11.0245460171454));
#59395=CARTESIAN_POINT('Ctrl Pts',(0.0966528472069954,-0.786139020026476,
-11.019250484314));
#59396=CARTESIAN_POINT('Ctrl Pts',(0.357290621499545,-0.753470372045547,
-11.008659418651));
#59397=CARTESIAN_POINT('Ctrl Pts',(0.598222139794698,-0.581114504840562,
-10.9980683529881));
#59398=CARTESIAN_POINT('Ctrl Pts',(0.712871995411302,-0.345231531789129,
-10.9874772873252));
#59399=CARTESIAN_POINT('Ctrl Pts',(0.770196923219604,-0.227290045263412,
-10.9821817544937));
#59400=CARTESIAN_POINT('Ctrl Pts',(0.795951435358268,-0.0934667822760847,
-10.9768862216622));
#59401=CARTESIAN_POINT('Ctrl Pts',(0.789598100866673,0.0384667449812388,
-10.9715906888308));
#59402=CARTESIAN_POINT('Ctrl Pts',(0.783244766375078,0.170400272238561,
-10.9662951559993));
#59403=CARTESIAN_POINT('Ctrl Pts',(0.744783585253222,0.300444063765881,
-10.9609996231678));
#59404=CARTESIAN_POINT('Ctrl Pts',(0.6762662963784,0.412168813037878,-10.9557040903364));
#59405=CARTESIAN_POINT('Ctrl Pts',(0.539231718628754,0.635618311581874,
-10.9451130246735));
#59406=CARTESIAN_POINT('Ctrl Pts',(0.281972709867238,0.785791641104585,
-10.9345219590105));
#59407=CARTESIAN_POINT('Ctrl Pts',(0.0201632244658906,0.792395229952745,
-10.9239308933476));
#59408=CARTESIAN_POINT('Ctrl Pts',(-0.241646260935457,0.798998818800906,
-10.9133398276847));
#59409=CARTESIAN_POINT('Ctrl Pts',(-0.508006222976634,0.662032666974516,
-10.9027487620217));
#59410=CARTESIAN_POINT('Ctrl Pts',(-0.655337672110363,0.445628276542215,
-10.8921576963588));
#59411=CARTESIAN_POINT('Ctrl Pts',(-0.74355397164707,0.316053805920492,
-10.8858161811804));
#59412=CARTESIAN_POINT('Ctrl Pts',(-0.789096820830231,0.157999573193716,
-10.879474666002));
#59413=CARTESIAN_POINT('Ctrl Pts',(-0.789614839096957,4.0911287493315E-5,
-10.8731331508237));
#59414=CARTESIAN_POINT('Origin',(0.,0.,-5.925));
#59415=CARTESIAN_POINT('',(-0.7911,-1.38777878078145E-15,-10.6446668491763));
#59416=CARTESIAN_POINT('',(-0.792077588667444,-0.000904661696636211,-10.6731331508237));
#59417=CARTESIAN_POINT('',(-0.7911,-9.68818082805471E-17,-5.925));
#59418=CARTESIAN_POINT('Ctrl Pts',(-0.7911,9.82547376793264E-15,-10.6446668491763));
#59419=CARTESIAN_POINT('Ctrl Pts',(-0.791099999999997,0.220167589666684,
-10.6535255927496));
#59420=CARTESIAN_POINT('Ctrl Pts',(-0.694214576672368,0.438610418338686,
-10.6623843363228));
#59421=CARTESIAN_POINT('Ctrl Pts',(-0.531017389080327,0.586395551223159,
-10.6712430798961));
#59422=CARTESIAN_POINT('Ctrl Pts',(-0.367820201488286,0.734180684107631,
-10.6801018234694));
#59423=CARTESIAN_POINT('Ctrl Pts',(-0.140868175871747,0.808992666571335,
-10.6889605670427));
#59424=CARTESIAN_POINT('Ctrl Pts',(0.078220547324759,0.787223447298297,
-10.6978193106159));
#59425=CARTESIAN_POINT('Ctrl Pts',(0.297309270521265,0.76545422802526,-10.7066780541892));
#59426=CARTESIAN_POINT('Ctrl Pts',(0.505102072675592,0.647444880834232,
-10.7155367977625));
#59427=CARTESIAN_POINT('Ctrl Pts',(0.636026795761728,0.470435038100978,
-10.7243955413357));
#59428=CARTESIAN_POINT('Ctrl Pts',(0.766951518847865,0.293425195367723,
-10.733254284909));
#59429=CARTESIAN_POINT('Ctrl Pts',(0.818956872247069,0.0601881960099378,
-10.7421130284823));
#59430=CARTESIAN_POINT('Ctrl Pts',(0.775631781004212,-0.155674501111244,
-10.7509717720556));
#59431=CARTESIAN_POINT('Ctrl Pts',(0.732306689761354,-0.371537198232426,
-10.7598305156288));
#59432=CARTESIAN_POINT('Ctrl Pts',(0.594329958850222,-0.566643518936489,
-10.7686892592021));
#59433=CARTESIAN_POINT('Ctrl Pts',(0.405242230244052,-0.679424716084738,
-10.7775480027754));
#59434=CARTESIAN_POINT('Ctrl Pts',(0.216154501637882,-0.792205913232988,
-10.7864067463487));
#59435=CARTESIAN_POINT('Ctrl Pts',(-0.021081652929998,-0.820894963713003,
-10.7952654899219));
#59436=CARTESIAN_POINT('Ctrl Pts',(-0.231602780753199,-0.756438604215429,
-10.8041242334952));
#59437=CARTESIAN_POINT('Ctrl Pts',(-0.4421239085764,-0.691982244717854,
-10.8129829770685));
#59438=CARTESIAN_POINT('Ctrl Pts',(-0.622631625634156,-0.535390358803556,
-10.8218417206417));
#59439=CARTESIAN_POINT('Ctrl Pts',(-0.716163994722142,-0.336077881842324,
-10.830700464215));
#59440=CARTESIAN_POINT('Ctrl Pts',(-0.76531728085948,-0.231334857514553,
-10.8353559258688));
#59441=CARTESIAN_POINT('Ctrl Pts',(-0.791099999999999,-0.11570283783654,
-10.8400113875225));
#59442=CARTESIAN_POINT('Ctrl Pts',(-0.7911,-7.21644966006352E-15,-10.8446668491763));
#59443=CARTESIAN_POINT('Ctrl Pts',(-0.789614839096957,4.0911287493315E-5,
-10.8731331508237));
#59444=CARTESIAN_POINT('Ctrl Pts',(-0.789961971401216,-0.105809707903876,
-10.8688836003391));
#59445=CARTESIAN_POINT('Ctrl Pts',(-0.770090460703084,-0.211617410503161,
-10.8646340498546));
#59446=CARTESIAN_POINT('Ctrl Pts',(-0.729292731490852,-0.308783330747756,
-10.86038449937));
#59447=CARTESIAN_POINT('Ctrl Pts',(-0.678453068501093,-0.429865624657486,
-10.8550889665386));
#59448=CARTESIAN_POINT('Ctrl Pts',(-0.595117839959883,-0.537528408262529,
-10.8497934337071));
#59449=CARTESIAN_POINT('Ctrl Pts',(-0.491678650585443,-0.619349253092896,
-10.8444979008756));
#59450=CARTESIAN_POINT('Ctrl Pts',(-0.388239461211004,-0.701170097923264,
-10.8392023680442));
#59451=CARTESIAN_POINT('Ctrl Pts',(-0.26469631100334,-0.757149003978955,
-10.8339068352127));
#59452=CARTESIAN_POINT('Ctrl Pts',(-0.13546718676572,-0.779650494055077,
-10.8286113023812));
#59453=CARTESIAN_POINT('Ctrl Pts',(-0.00623806252809894,-0.8021519841312,
-10.8233157695498));
#59454=CARTESIAN_POINT('Ctrl Pts',(0.128677035739474,-0.79117605822775,
-10.8180202367183));
#59455=CARTESIAN_POINT('Ctrl Pts',(0.253692330652354,-0.748995963619501,
-10.8127247038868));
#59456=CARTESIAN_POINT('Ctrl Pts',(0.378707625565232,-0.706815869011252,
-10.8074291710554));
#59457=CARTESIAN_POINT('Ctrl Pts',(0.493823117123418,-0.633431605698205,
-10.8021336382239));
#59458=CARTESIAN_POINT('Ctrl Pts',(0.58257691189074,-0.536619486613459,
-10.7968381053924));
#59459=CARTESIAN_POINT('Ctrl Pts',(0.760084501425384,-0.342995248443968,
-10.7862470397295));
#59460=CARTESIAN_POINT('Ctrl Pts',(0.832145303796571,-0.0556595871876777,
-10.7756559740666));
#59461=CARTESIAN_POINT('Ctrl Pts',(0.766830956709737,0.198347110426995,
-10.7650649084037));
#59462=CARTESIAN_POINT('Ctrl Pts',(0.734173783166319,0.325350459234334,
-10.7597693755722));
#59463=CARTESIAN_POINT('Ctrl Pts',(0.667172822258395,0.444021567131268,
-10.7544738427407));
#59464=CARTESIAN_POINT('Ctrl Pts',(0.576922880519699,0.540467243498233,
-10.7491783099093));
#59465=CARTESIAN_POINT('Ctrl Pts',(0.486672938781004,0.636912919865197,
-10.7438827770778));
#59466=CARTESIAN_POINT('Ctrl Pts',(0.373174016211536,0.711133164702193,
-10.7385872442463));
#59467=CARTESIAN_POINT('Ctrl Pts',(0.248625480727413,0.751933909590113,
-10.7332917114149));
#59468=CARTESIAN_POINT('Ctrl Pts',(-0.000471590240832209,0.833535399365951,
-10.7227006457519));
#59469=CARTESIAN_POINT('Ctrl Pts',(-0.293767112867703,0.781458889345488,
-10.712109580089));
#59470=CARTESIAN_POINT('Ctrl Pts',(-0.497590747514042,0.617009079399273,
-10.7015185144261));
#59471=CARTESIAN_POINT('Ctrl Pts',(-0.679681582825412,0.470093814582901,
-10.6920567265586));
#59472=CARTESIAN_POINT('Ctrl Pts',(-0.790363295957457,0.233491399028885,
-10.6825949386912));
#59473=CARTESIAN_POINT('Ctrl Pts',(-0.792077588667444,-0.000904661696636211,
-10.6731331508237));
#59474=CARTESIAN_POINT('Origin',(0.,0.,-5.925));
#59475=CARTESIAN_POINT('',(-0.7911,-6.82787160144471E-15,-10.4446668491763));
#59476=CARTESIAN_POINT('',(-0.791602053176032,0.00100009030957082,-10.4731331508237));
#59477=CARTESIAN_POINT('',(-0.7911,-9.68818082805471E-17,-5.925));
#59478=CARTESIAN_POINT('Ctrl Pts',(-0.7911,-1.24344978758018E-14,-10.4446668491763));
#59479=CARTESIAN_POINT('Ctrl Pts',(-0.791100000000003,0.220167589666665,
-10.4535255927496));
#59480=CARTESIAN_POINT('Ctrl Pts',(-0.694214576672377,0.438610418338674,
-10.4623843363228));
#59481=CARTESIAN_POINT('Ctrl Pts',(-0.531017389080335,0.586395551223151,
-10.4712430798961));
#59482=CARTESIAN_POINT('Ctrl Pts',(-0.367820201488294,0.734180684107628,
-10.4801018234694));
#59483=CARTESIAN_POINT('Ctrl Pts',(-0.140868175871751,0.808992666571336,
-10.4889605670427));
#59484=CARTESIAN_POINT('Ctrl Pts',(0.0782205473247591,0.787223447298297,
-10.4978193106159));
#59485=CARTESIAN_POINT('Ctrl Pts',(0.297309270521269,0.765454228025259,
-10.5066780541892));
#59486=CARTESIAN_POINT('Ctrl Pts',(0.5051020726756,0.647444880834228,-10.5155367977625));
#59487=CARTESIAN_POINT('Ctrl Pts',(0.636026795761735,0.470435038100969,
-10.5243955413357));
#59488=CARTESIAN_POINT('Ctrl Pts',(0.766951518847871,0.293425195367709,
-10.533254284909));
#59489=CARTESIAN_POINT('Ctrl Pts',(0.818956872247071,0.060188196009918,
-10.5421130284823));
#59490=CARTESIAN_POINT('Ctrl Pts',(0.775631781004207,-0.155674501111266,
-10.5509717720556));
#59491=CARTESIAN_POINT('Ctrl Pts',(0.732306689761343,-0.37153719823245,
-10.5598305156288));
#59492=CARTESIAN_POINT('Ctrl Pts',(0.594329958850201,-0.566643518936512,
-10.5686892592021));
#59493=CARTESIAN_POINT('Ctrl Pts',(0.405242230244022,-0.679424716084756,
-10.5775480027754));
#59494=CARTESIAN_POINT('Ctrl Pts',(0.216154501637844,-0.792205913232999,
-10.5864067463487));
#59495=CARTESIAN_POINT('Ctrl Pts',(-0.0210816529300414,-0.820894963713003,
-10.5952654899219));
#59496=CARTESIAN_POINT('Ctrl Pts',(-0.231602780753242,-0.756438604215415,
-10.6041242334952));
#59497=CARTESIAN_POINT('Ctrl Pts',(-0.442123908576443,-0.691982244717828,
-10.6129829770685));
#59498=CARTESIAN_POINT('Ctrl Pts',(-0.622631625634193,-0.535390358803515,
-10.6218417206417));
#59499=CARTESIAN_POINT('Ctrl Pts',(-0.716163994722166,-0.336077881842273,
-10.630700464215));
#59500=CARTESIAN_POINT('Ctrl Pts',(-0.765317280859491,-0.23133485751451,
-10.6353559258688));
#59501=CARTESIAN_POINT('Ctrl Pts',(-0.791100000000001,-0.11570283783651,
-10.6400113875225));
#59502=CARTESIAN_POINT('Ctrl Pts',(-0.7911,9.82547376793264E-15,-10.6446668491763));
#59503=CARTESIAN_POINT('Ctrl Pts',(-0.792077588667444,-0.000904661696636211,
-10.6731331508237));
#59504=CARTESIAN_POINT('Ctrl Pts',(-0.792282191932643,-0.0288801638351418,
-10.6720038730282));
#59505=CARTESIAN_POINT('Ctrl Pts',(-0.790934580348652,-0.0568242369766668,
-10.6708745952328));
#59506=CARTESIAN_POINT('Ctrl Pts',(-0.787970899835483,-0.0845806499944255,
-10.6697453174373));
#59507=CARTESIAN_POINT('Ctrl Pts',(-0.760175670844775,-0.344897459569937,
-10.6591542517744));
#59508=CARTESIAN_POINT('Ctrl Pts',(-0.590233466197554,-0.588707968848993,
-10.6485631861114));
#59509=CARTESIAN_POINT('Ctrl Pts',(-0.35596858505029,-0.70746123569448,
-10.6379721204485));
#59510=CARTESIAN_POINT('Ctrl Pts',(-0.238836144476656,-0.766837869117224,
-10.632676587617));
#59511=CARTESIAN_POINT('Ctrl Pts',(-0.105623034778013,-0.794950191931574,
-10.6273810547856));
#59512=CARTESIAN_POINT('Ctrl Pts',(0.0261842875608677,-0.79035167857934,
-10.6220855219541));
#59513=CARTESIAN_POINT('Ctrl Pts',(0.157991609899747,-0.785753165227106,
-10.6167899891227));
#59514=CARTESIAN_POINT('Ctrl Pts',(0.288393144878865,-0.748443815708286,
-10.6114944562912));
#59515=CARTESIAN_POINT('Ctrl Pts',(0.401456790697708,-0.68193745810979,
-10.6061989234597));
#59516=CARTESIAN_POINT('Ctrl Pts',(0.514520436516553,-0.615431100511294,
-10.6009033906283));
#59517=CARTESIAN_POINT('Ctrl Pts',(0.610246193175124,-0.519727734833122,
-10.5956078577968));
#59518=CARTESIAN_POINT('Ctrl Pts',(0.67822631641647,-0.406649500024621,
-10.5903123249653));
#59519=CARTESIAN_POINT('Ctrl Pts',(0.746206439657815,-0.293571265216123,
-10.5850167921339));
#59520=CARTESIAN_POINT('Ctrl Pts',(0.786440929481935,-0.163118161277295,
-10.5797212593024));
#59521=CARTESIAN_POINT('Ctrl Pts',(0.791416696910816,-0.0318738691127503,
-10.5744257264709));
#59522=CARTESIAN_POINT('Ctrl Pts',(0.801368231768579,0.230614715216342,
-10.563834660808));
#59523=CARTESIAN_POINT('Ctrl Pts',(0.67028487704539,0.49626805244831,-10.5532435951451));
#59524=CARTESIAN_POINT('Ctrl Pts',(0.456071030378218,0.647588223821943,
-10.5426525294821));
#59525=CARTESIAN_POINT('Ctrl Pts',(0.348964107044634,0.723248309508759,
-10.5373569966507));
#59526=CARTESIAN_POINT('Ctrl Pts',(0.221074560725051,0.770325103730992,
-10.5320614638192));
#59527=CARTESIAN_POINT('Ctrl Pts',(0.0898525416784706,0.785411594080227,
-10.5267659309878));
#59528=CARTESIAN_POINT('Ctrl Pts',(-0.0413694773681122,0.800498084429462,
-10.5214703981563));
#59529=CARTESIAN_POINT('Ctrl Pts',(-0.175923969141694,0.783594270905701,
-10.5161748653248));
#59530=CARTESIAN_POINT('Ctrl Pts',(-0.297266180137799,0.734065427741078,
-10.5108793324933));
#59531=CARTESIAN_POINT('Ctrl Pts',(-0.539950602130008,0.635007741411831,
-10.5002882668304));
#59532=CARTESIAN_POINT('Ctrl Pts',(-0.7297859010123,0.405449936519141,-10.4896972011675));
#59533=CARTESIAN_POINT('Ctrl Pts',(-0.778681420574774,0.148162077888954,
-10.4791061355046));
#59534=CARTESIAN_POINT('Ctrl Pts',(-0.787873199085899,0.099795008036908,
-10.4771151406109));
#59535=CARTESIAN_POINT('Ctrl Pts',(-0.792084229722408,0.0504479706633907,
-10.4751241457173));
#59536=CARTESIAN_POINT('Ctrl Pts',(-0.791602053176032,0.00100009030957082,
-10.4731331508237));
#59537=CARTESIAN_POINT('Origin',(0.,0.,-5.925));
#59538=CARTESIAN_POINT('',(-0.7911,-1.2267964422108E-14,-10.2446668491763));
#59539=CARTESIAN_POINT('',(-0.789494028330408,-8.20471835821903E-5,-10.2731331508237));
#59540=CARTESIAN_POINT('',(-0.7911,-9.68818082805471E-17,-5.925));
#59541=CARTESIAN_POINT('Ctrl Pts',(-0.7911,4.55191440096314E-15,-10.2446668491763));
#59542=CARTESIAN_POINT('Ctrl Pts',(-0.791099999999999,0.220167589666681,
-10.2535255927496));
#59543=CARTESIAN_POINT('Ctrl Pts',(-0.694214576672369,0.438610418338685,
-10.2623843363228));
#59544=CARTESIAN_POINT('Ctrl Pts',(-0.531017389080327,0.586395551223159,
-10.2712430798961));
#59545=CARTESIAN_POINT('Ctrl Pts',(-0.367820201488285,0.734180684107633,
-10.2801018234694));
#59546=CARTESIAN_POINT('Ctrl Pts',(-0.140868175871743,0.808992666571336,
-10.2889605670427));
#59547=CARTESIAN_POINT('Ctrl Pts',(0.0782205473247649,0.787223447298297,
-10.2978193106159));
#59548=CARTESIAN_POINT('Ctrl Pts',(0.297309270521273,0.765454228025257,
-10.3066780541892));
#59549=CARTESIAN_POINT('Ctrl Pts',(0.505102072675601,0.647444880834227,
-10.3155367977625));
#59550=CARTESIAN_POINT('Ctrl Pts',(0.636026795761735,0.470435038100968,
-10.3243955413357));
#59551=CARTESIAN_POINT('Ctrl Pts',(0.76695151884787,0.29342519536771,-10.333254284909));
#59552=CARTESIAN_POINT('Ctrl Pts',(0.818956872247071,0.0601881960099218,
-10.3421130284823));
#59553=CARTESIAN_POINT('Ctrl Pts',(0.775631781004208,-0.155674501111261,
-10.3509717720556));
#59554=CARTESIAN_POINT('Ctrl Pts',(0.732306689761346,-0.371537198232443,
-10.3598305156288));
#59555=CARTESIAN_POINT('Ctrl Pts',(0.594329958850207,-0.566643518936505,
-10.3686892592021));
#59556=CARTESIAN_POINT('Ctrl Pts',(0.405242230244032,-0.67942471608475,
-10.3775480027754));
#59557=CARTESIAN_POINT('Ctrl Pts',(0.216154501637857,-0.792205913232995,
-10.3864067463487));
#59558=CARTESIAN_POINT('Ctrl Pts',(-0.0210816529300259,-0.820894963713002,
-10.3952654899219));
#59559=CARTESIAN_POINT('Ctrl Pts',(-0.231602780753226,-0.75643860421542,
-10.4041242334952));
#59560=CARTESIAN_POINT('Ctrl Pts',(-0.442123908576426,-0.691982244717838,
-10.4129829770685));
#59561=CARTESIAN_POINT('Ctrl Pts',(-0.622631625634179,-0.535390358803531,
-10.4218417206417));
#59562=CARTESIAN_POINT('Ctrl Pts',(-0.716163994722157,-0.336077881842293,
-10.430700464215));
#59563=CARTESIAN_POINT('Ctrl Pts',(-0.765317280859485,-0.231334857514532,
-10.4353559258688));
#59564=CARTESIAN_POINT('Ctrl Pts',(-0.791099999999998,-0.115702837836532,
-10.4400113875225));
#59565=CARTESIAN_POINT('Ctrl Pts',(-0.7911,-1.24344978758018E-14,-10.4446668491763));
#59566=CARTESIAN_POINT('Ctrl Pts',(-0.791602053176032,0.00100009030957082,
-10.4731331508237));
#59567=CARTESIAN_POINT('Ctrl Pts',(-0.789519299254671,-0.212589242236902,
-10.4645330800544));
#59568=CARTESIAN_POINT('Ctrl Pts',(-0.699870954088247,-0.428060097343416,
-10.4559330092851));
#59569=CARTESIAN_POINT('Ctrl Pts',(-0.545830694696212,-0.574561465875036,
-10.4473329385158));
#59570=CARTESIAN_POINT('Ctrl Pts',(-0.356128709012524,-0.754979238641152,
-10.4367418728528));
#59571=CARTESIAN_POINT('Ctrl Pts',(-0.0687689974024994,-0.830796871805704,
-10.4261508071899));
#59572=CARTESIAN_POINT('Ctrl Pts',(0.186660758624119,-0.769657582787913,
-10.415559741527));
#59573=CARTESIAN_POINT('Ctrl Pts',(0.314375636637429,-0.739087938279018,
-10.4102642086955));
#59574=CARTESIAN_POINT('Ctrl Pts',(0.434108025754885,-0.674279063224538,
-10.4049686758641));
#59575=CARTESIAN_POINT('Ctrl Pts',(0.531593497608413,-0.585448329102326,
-10.3996731430326));
#59576=CARTESIAN_POINT('Ctrl Pts',(0.629078969461942,-0.496617594980113,
-10.3943776102011));
#59577=CARTESIAN_POINT('Ctrl Pts',(0.70431752405154,-0.38376500179017,-10.3890820773697));
#59578=CARTESIAN_POINT('Ctrl Pts',(0.747440544825585,-0.25988244173352,
-10.3837865445382));
#59579=CARTESIAN_POINT('Ctrl Pts',(0.790563565599631,-0.135999881676871,
-10.3784910117067));
#59580=CARTESIAN_POINT('Ctrl Pts',(0.801571052558123,-0.00108735475351671,
-10.3731954788753));
#59581=CARTESIAN_POINT('Ctrl Pts',(0.780183408902627,0.129106934837772,
-10.3678999460438));
#59582=CARTESIAN_POINT('Ctrl Pts',(0.758795765247131,0.25930122442906,-10.3626044132124));
#59583=CARTESIAN_POINT('Ctrl Pts',(0.705012990977646,0.384777276688281,
-10.3573088803809));
#59584=CARTESIAN_POINT('Ctrl Pts',(0.623844164687467,0.488031545975095,
-10.3520133475494));
#59585=CARTESIAN_POINT('Ctrl Pts',(0.46150651210711,0.694540084548719,-10.3414222818865));
#59586=CARTESIAN_POINT('Ctrl Pts',(0.189624651443974,0.812161491232711,
-10.3308312162236));
#59587=CARTESIAN_POINT('Ctrl Pts',(-0.0716046547973555,0.788824483516112,
-10.3202401505606));
#59588=CARTESIAN_POINT('Ctrl Pts',(-0.202219307918021,0.777155979657812,
-10.3149446177292));
#59589=CARTESIAN_POINT('Ctrl Pts',(-0.330170822433236,0.730247872199365,
-10.3096490848977));
#59590=CARTESIAN_POINT('Ctrl Pts',(-0.439953316334173,0.656799764622589,
-10.3043535520662));
#59591=CARTESIAN_POINT('Ctrl Pts',(-0.549735810235111,0.583351657045813,
-10.2990580192348));
#59592=CARTESIAN_POINT('Ctrl Pts',(-0.641349283521772,0.483363549350709,
-10.2937624864033));
#59593=CARTESIAN_POINT('Ctrl Pts',(-0.701772585750591,0.367061945654053,
-10.2884669535718));
#59594=CARTESIAN_POINT('Ctrl Pts',(-0.760093377208675,0.254807214031685,
-10.2833556859891));
#59595=CARTESIAN_POINT('Ctrl Pts',(-0.789356841601489,0.127354534696367,
-10.2782444184064));
#59596=CARTESIAN_POINT('Ctrl Pts',(-0.789494028330408,-8.20471835821903E-5,
-10.2731331508237));
#59597=CARTESIAN_POINT('Origin',(0.,0.,-5.925));
#59598=CARTESIAN_POINT('',(-0.790401422788456,-0.000312835344477125,-10.0446668491763));
#59599=CARTESIAN_POINT('',(-0.791423880525058,-0.000561432253963593,-10.0731331508237));
#59600=CARTESIAN_POINT('',(-0.7911,-9.68818082805471E-17,-5.925));
#59601=CARTESIAN_POINT('Ctrl Pts',(-0.790401422788456,-0.000312835344477125,
-10.0446668491763));
#59602=CARTESIAN_POINT('Ctrl Pts',(-0.788697176084344,0.197685440689488,
-10.0526302499402));
#59603=CARTESIAN_POINT('Ctrl Pts',(-0.714105001319401,0.396267685858613,
-10.0605936507041));
#59604=CARTESIAN_POINT('Ctrl Pts',(-0.579842908951946,0.540216832650709,
-10.0685570514681));
#59605=CARTESIAN_POINT('Ctrl Pts',(-0.401278665048899,0.731664545882161,
-10.079148117131));
#59606=CARTESIAN_POINT('Ctrl Pts',(-0.117169433251898,0.826476467771916,
-10.0897391827939));
#59607=CARTESIAN_POINT('Ctrl Pts',(0.140581802644246,0.780085580457693,
-10.1003302484568));
#59608=CARTESIAN_POINT('Ctrl Pts',(0.398333038540391,0.733694693143469,
-10.1109213141198));
#59609=CARTESIAN_POINT('Ctrl Pts',(0.629726278535683,0.546100996625268,
-10.1215123797827));
#59610=CARTESIAN_POINT('Ctrl Pts',(0.731139569969053,0.304391463881425,
-10.1321034454456));
#59611=CARTESIAN_POINT('Ctrl Pts',(0.781846215685738,0.183536697509504,
-10.1373989782771));
#59612=CARTESIAN_POINT('Ctrl Pts',(0.800057874261942,0.0491529720811725,
-10.1426945111086));
#59613=CARTESIAN_POINT('Ctrl Pts',(0.786248331162366,-0.082209568215139,
-10.14799004394));
#59614=CARTESIAN_POINT('Ctrl Pts',(0.77243878806279,-0.21357210851145,-10.1532855767715));
#59615=CARTESIAN_POINT('Ctrl Pts',(0.726608043287434,-0.341913463675741,
-10.1585811096029));
#59616=CARTESIAN_POINT('Ctrl Pts',(0.65199323215211,-0.449751172995639,
-10.1638766424344));
#59617=CARTESIAN_POINT('Ctrl Pts',(0.502763609881462,-0.665426591635433,
-10.1744677080973));
#59618=CARTESIAN_POINT('Ctrl Pts',(0.238397722170937,-0.799087426897659,
-10.1850587737603));
#59619=CARTESIAN_POINT('Ctrl Pts',(-0.0241752336446996,-0.791689263385369,
-10.1956498394232));
#59620=CARTESIAN_POINT('Ctrl Pts',(-0.155461711552519,-0.787990181629224,
-10.2009453722547));
#59621=CARTESIAN_POINT('Ctrl Pts',(-0.286299956486616,-0.749026350179451,
-10.2062409050861));
#59622=CARTESIAN_POINT('Ctrl Pts',(-0.400034001397628,-0.682149213791184,
-10.2115364379176));
#59623=CARTESIAN_POINT('Ctrl Pts',(-0.513768046308639,-0.615272077402917,
-10.2168319707491));
#59624=CARTESIAN_POINT('Ctrl Pts',(-0.610397891196563,-0.520481636076158,
-10.2221275035805));
#59625=CARTESIAN_POINT('Ctrl Pts',(-0.678000733044698,-0.408070162547321,
-10.227423036412));
#59626=CARTESIAN_POINT('Ctrl Pts',(-0.745603574892832,-0.295658689018485,
-10.2327185692435));
#59627=CARTESIAN_POINT('Ctrl Pts',(-0.784179413701176,-0.165626183287574,
-10.2380141020749));
#59628=CARTESIAN_POINT('Ctrl Pts',(-0.79005963579369,-0.0338698189808012,
-10.2433096349064));
#59629=CARTESIAN_POINT('Ctrl Pts',(-0.790561991369495,-0.0226136889884339,
-10.243762039663));
#59630=CARTESIAN_POINT('Ctrl Pts',(-0.790825717226918,-0.0113449773741918,
-10.2442144444197));
#59631=CARTESIAN_POINT('Ctrl Pts',(-0.790851609223311,-7.45956026386718E-5,
-10.2446668491763));
#59632=CARTESIAN_POINT('Ctrl Pts',(-0.789494028330408,-8.20471835821903E-5,
-10.2731331508237));
#59633=CARTESIAN_POINT('Ctrl Pts',(-0.789641106440014,-0.136707008689031,
-10.2676533527435));
#59634=CARTESIAN_POINT('Ctrl Pts',(-0.756310388284488,-0.273313467750145,
-10.2621735546633));
#59635=CARTESIAN_POINT('Ctrl Pts',(-0.689416907730222,-0.391153529203585,
-10.2566937565831));
#59636=CARTESIAN_POINT('Ctrl Pts',(-0.560128705025943,-0.618908605268401,
-10.2461026909201));
#59637=CARTESIAN_POINT('Ctrl Pts',(-0.305466379391119,-0.776561565998511,
-10.2355116252572));
#59638=CARTESIAN_POINT('Ctrl Pts',(-0.0440833857200287,-0.791270295439225,
-10.2249205595943));
#59639=CARTESIAN_POINT('Ctrl Pts',(0.217299607951058,-0.805979024879939,
-10.2143294939313));
#59640=CARTESIAN_POINT('Ctrl Pts',(0.485403269658407,-0.677743523031253,
-10.2037384282684));
#59641=CARTESIAN_POINT('Ctrl Pts',(0.640510817041626,-0.465790646971077,
-10.1931473626055));
#59642=CARTESIAN_POINT('Ctrl Pts',(0.718064590733235,-0.359814208940989,
-10.187851829774));
#59643=CARTESIAN_POINT('Ctrl Pts',(0.767369335843814,-0.232908427358027,
-10.1825562969426));
#59644=CARTESIAN_POINT('Ctrl Pts',(0.784167076252959,-0.102095001195637,
-10.1772607641111));
#59645=CARTESIAN_POINT('Ctrl Pts',(0.800964816662105,0.0287184249667539,
-10.1719652312796));
#59646=CARTESIAN_POINT('Ctrl Pts',(0.785255552369819,0.163439495708571,
-10.1666696984482));
#59647=CARTESIAN_POINT('Ctrl Pts',(0.737927847365211,0.285777437271543,
-10.1613741656167));
#59648=CARTESIAN_POINT('Ctrl Pts',(0.690600142360604,0.408115378834514,
-10.1560786327852));
#59649=CARTESIAN_POINT('Ctrl Pts',(0.611653996643675,0.518070191218638,
-10.1507830999538));
#59650=CARTESIAN_POINT('Ctrl Pts',(0.511070942247287,0.603457740144741,
-10.1454875671223));
#59651=CARTESIAN_POINT('Ctrl Pts',(0.410487887850897,0.688845289070846,
-10.1401920342908));
#59652=CARTESIAN_POINT('Ctrl Pts',(0.288267924775049,0.749665574538929,
-10.1348965014594));
#59653=CARTESIAN_POINT('Ctrl Pts',(0.159559889402088,0.775820193972442,
-10.1296009686279));
#59654=CARTESIAN_POINT('Ctrl Pts',(-0.0978561813438297,0.828129432839467,
-10.119009902965));
#59655=CARTESIAN_POINT('Ctrl Pts',(-0.381224541278192,0.741776007568202,
-10.108418837302));
#59656=CARTESIAN_POINT('Ctrl Pts',(-0.565223850966701,0.554881330269348,
-10.0978277716391));
#59657=CARTESIAN_POINT('Ctrl Pts',(-0.657223505810957,0.461433991619919,
-10.0925322388077));
#59658=CARTESIAN_POINT('Ctrl Pts',(-0.724380898093749,0.342851339963596,
-10.0872367059762));
#59659=CARTESIAN_POINT('Ctrl Pts',(-0.760509296341098,0.215801903468189,
-10.0819411731447));
#59660=CARTESIAN_POINT('Ctrl Pts',(-0.780539999471085,0.145361760291943,
-10.0790051657044));
#59661=CARTESIAN_POINT('Ctrl Pts',(-0.791032585068395,0.072318980729004,
-10.076069158264));
#59662=CARTESIAN_POINT('Ctrl Pts',(-0.791423880525058,-0.000561432253963593,
-10.0731331508237));
#59663=CARTESIAN_POINT('Origin',(0.,0.,-5.925));
#59664=CARTESIAN_POINT('',(-0.792437169753526,-0.000127296230932911,-9.8446668491763));
#59665=CARTESIAN_POINT('',(-0.791999899124744,0.000522216889476513,-9.87313315082368));
#59666=CARTESIAN_POINT('',(-0.7911,-9.68818082805471E-17,-5.925));
#59667=CARTESIAN_POINT('Ctrl Pts',(-0.792437169753526,-0.000127296230932911,
-9.8446668491763));
#59668=CARTESIAN_POINT('Ctrl Pts',(-0.792483963508099,0.0120472072685257,
-9.84515945696638));
#59669=CARTESIAN_POINT('Ctrl Pts',(-0.792227470903532,0.0242221673588838,
-9.84565206475646));
#59670=CARTESIAN_POINT('Ctrl Pts',(-0.791661615652341,0.0363855966523024,
-9.84614467254654));
#59671=CARTESIAN_POINT('Ctrl Pts',(-0.779495729846714,0.297899281427651,
-9.85673573820947));
#59672=CARTESIAN_POINT('Ctrl Pts',(-0.624327009889845,0.554082857153437,
-9.86732680387239));
#59673=CARTESIAN_POINT('Ctrl Pts',(-0.397840131682881,0.685580035951506,
-9.87791786953532));
#59674=CARTESIAN_POINT('Ctrl Pts',(-0.171353253475907,0.817077214749582,
-9.88850893519825));
#59675=CARTESIAN_POINT('Ctrl Pts',(0.126451782981168,0.823887996619928,
-9.89910000086118));
#59676=CARTESIAN_POINT('Ctrl Pts',(0.360219314034763,0.705309350465974,
-9.90969106652411));
#59677=CARTESIAN_POINT('Ctrl Pts',(0.477103079561559,0.646020027388998,
-9.91498659935558));
#59678=CARTESIAN_POINT('Ctrl Pts',(0.577977468737485,0.555383347305948,
-9.92028213218705));
#59679=CARTESIAN_POINT('Ctrl Pts',(0.652489820552396,0.446320384294988,
-9.92557766501851));
#59680=CARTESIAN_POINT('Ctrl Pts',(0.727002172367308,0.337257421284029,
-9.93087319784997));
#59681=CARTESIAN_POINT('Ctrl Pts',(0.775152486821205,0.209768175345161,
-9.93616873068143));
#59682=CARTESIAN_POINT('Ctrl Pts',(0.788090765422098,0.0792731848705502,
-9.94146426351289));
#59683=CARTESIAN_POINT('Ctrl Pts',(0.813967322623884,-0.181716796078669,
-9.95205532917582));
#59684=CARTESIAN_POINT('Ctrl Pts',(0.698995736413652,-0.454729755170857,
-9.96264639483875));
#59685=CARTESIAN_POINT('Ctrl Pts',(0.494075821794957,-0.619068182027699,
-9.97323746050169));
#59686=CARTESIAN_POINT('Ctrl Pts',(0.391615864485609,-0.701237395456121,
-9.97853299333315));
#59687=CARTESIAN_POINT('Ctrl Pts',(0.266668825074145,-0.756237975825707,
-9.98382852616462));
#59688=CARTESIAN_POINT('Ctrl Pts',(0.136688704257258,-0.778890846190016,
-9.98912405899608));
#59689=CARTESIAN_POINT('Ctrl Pts',(0.00670858344037104,-0.801543716554325,
-9.99441959182754));
#59690=CARTESIAN_POINT('Ctrl Pts',(-0.128304618781938,-0.791848876913358,
-9.99971512465901));
#59691=CARTESIAN_POINT('Ctrl Pts',(-0.252600723751825,-0.749932747605143,
-10.0050106574905));
#59692=CARTESIAN_POINT('Ctrl Pts',(-0.376896828721711,-0.708016618296928,
-10.0103061903219));
#59693=CARTESIAN_POINT('Ctrl Pts',(-0.490475836439174,-0.633879199321465,
-10.0156017231534));
#59694=CARTESIAN_POINT('Ctrl Pts',(-0.580250489386907,-0.537262284470542,
-10.0208972559849));
#59695=CARTESIAN_POINT('Ctrl Pts',(-0.670025142334639,-0.44064536961962,
-10.0261927888163));
#59696=CARTESIAN_POINT('Ctrl Pts',(-0.735995440512639,-0.321548958893238,
-10.0314883216478));
#59697=CARTESIAN_POINT('Ctrl Pts',(-0.767805763296456,-0.194137434313457,
-10.0367838544793));
#59698=CARTESIAN_POINT('Ctrl Pts',(-0.783590174660805,-0.130915318329486,
-10.0394115193783));
#59699=CARTESIAN_POINT('Ctrl Pts',(-0.790963769124703,-0.0656458677288963,
-10.0420391842773));
#59700=CARTESIAN_POINT('Ctrl Pts',(-0.790401422788456,-0.000312835344477125,
-10.0446668491763));
#59701=CARTESIAN_POINT('Ctrl Pts',(-0.791423880525058,-0.000561432253963593,
-10.0731331508237));
#59702=CARTESIAN_POINT('Ctrl Pts',(-0.791738345520185,-0.0591318509064546,
-10.0707736254326));
#59703=CARTESIAN_POINT('Ctrl Pts',(-0.785528842062187,-0.117597404296111,
-10.0684141000415));
#59704=CARTESIAN_POINT('Ctrl Pts',(-0.772503059908576,-0.174522939725115,
-10.0660545746503));
#59705=CARTESIAN_POINT('Ctrl Pts',(-0.714034982125027,-0.430041310451943,
-10.0554635089874));
#59706=CARTESIAN_POINT('Ctrl Pts',(-0.518233131926761,-0.654531537294492,
-10.0448724433245));
#59707=CARTESIAN_POINT('Ctrl Pts',(-0.272253050837869,-0.744429333370331,
-10.0342813776615));
#59708=CARTESIAN_POINT('Ctrl Pts',(-0.0262729697489752,-0.83432712944617,
-10.0236903119986));
#59709=CARTESIAN_POINT('Ctrl Pts',(0.269885342230544,-0.7896324947553,-10.0130992463357));
#59710=CARTESIAN_POINT('Ctrl Pts',(0.478630791197635,-0.631636438988873,
-10.0025081806728));
#59711=CARTESIAN_POINT('Ctrl Pts',(0.687376240164726,-0.473640383222446,
-9.99191711500984));
#59712=CARTESIAN_POINT('Ctrl Pts',(0.808708826119385,-0.202342906380464,
-9.98132604934689));
#59713=CARTESIAN_POINT('Ctrl Pts',(0.789722166415962,0.0596148758645482,
-9.97073498368396));
#59714=CARTESIAN_POINT('Ctrl Pts',(0.78022883656425,0.190593766987052,-9.9654394508525));
#59715=CARTESIAN_POINT('Ctrl Pts',(0.735655695298016,0.319237734460317,
-9.96014391802105));
#59716=CARTESIAN_POINT('Ctrl Pts',(0.663776390394953,0.429816584489825,
-9.95484838518958));
#59717=CARTESIAN_POINT('Ctrl Pts',(0.591897085491888,0.540395434519333,
-9.94955285235812));
#59718=CARTESIAN_POINT('Ctrl Pts',(0.492711616951992,0.632909167105086,
-9.94425731952665));
#59719=CARTESIAN_POINT('Ctrl Pts',(0.377443111951363,0.695516318148622,
-9.93896178669518));
#59720=CARTESIAN_POINT('Ctrl Pts',(0.262174606950734,0.758123469192158,
-9.93366625386372));
#59721=CARTESIAN_POINT('Ctrl Pts',(0.130823065489374,0.790824038693476,
-9.92837072103225));
#59722=CARTESIAN_POINT('Ctrl Pts',(-0.00111625153724639,0.7907929603459,
-9.92307518820079));
#59723=CARTESIAN_POINT('Ctrl Pts',(-0.133055568563865,0.790761881998325,
-9.91777965536932));
#59724=CARTESIAN_POINT('Ctrl Pts',(-0.265582661155748,0.757999155801856,
-9.91248412253786));
#59725=CARTESIAN_POINT('Ctrl Pts',(-0.380613999968237,0.694614507989592,
-9.90718858970639));
#59726=CARTESIAN_POINT('Ctrl Pts',(-0.61067667759322,0.567845212365061,
-9.89659752404346));
#59727=CARTESIAN_POINT('Ctrl Pts',(-0.770756340100645,0.318588230277345,
-9.88600645838054));
#59728=CARTESIAN_POINT('Ctrl Pts',(-0.790012201976854,0.0570264246712957,
-9.87541539271761));
#59729=CARTESIAN_POINT('Ctrl Pts',(-0.791395334265783,0.0382386611730939,
-9.87465464541963));
#59730=CARTESIAN_POINT('Ctrl Pts',(-0.792051896362309,0.019387411829807,
-9.87389389812165));
#59731=CARTESIAN_POINT('Ctrl Pts',(-0.791999899124744,0.000522216889476513,
-9.87313315082368));
#59732=CARTESIAN_POINT('Origin',(0.,0.,-5.925));
#59733=CARTESIAN_POINT('',(-0.790332566743882,0.00078097778472147,-9.6446668491763));
#59734=CARTESIAN_POINT('',(-0.79049273289666,5.48490963145453E-5,-9.67313315082367));
#59735=CARTESIAN_POINT('',(-0.7911,-9.68818082805471E-17,-5.925));
#59736=CARTESIAN_POINT('Ctrl Pts',(-0.790332566743882,0.00078097778472147,
-9.6446668491763));
#59737=CARTESIAN_POINT('Ctrl Pts',(-0.791021644760839,0.0909049416404772,
-9.64827972965547));
#59738=CARTESIAN_POINT('Ctrl Pts',(-0.776890865898073,0.180795718990353,
-9.65189261013465));
#59739=CARTESIAN_POINT('Ctrl Pts',(-0.747041992130169,0.265000034088506,
-9.65550549061382));
#59740=CARTESIAN_POINT('Ctrl Pts',(-0.659540790841399,0.511842805513576,
-9.66609655627675));
#59741=CARTESIAN_POINT('Ctrl Pts',(-0.436965503137771,0.709818732819205,
-9.67668762193967));
#59742=CARTESIAN_POINT('Ctrl Pts',(-0.182027863912829,0.77076915533624,
-9.6872786876026));
#59743=CARTESIAN_POINT('Ctrl Pts',(-0.0545590443003537,0.801244366594759,
-9.69257422043406));
#59744=CARTESIAN_POINT('Ctrl Pts',(0.0810003631924518,0.797463201656127,
-9.69786975326553));
#59745=CARTESIAN_POINT('Ctrl Pts',(0.208395166807512,0.762572164331347,
-9.703165286097));
#59746=CARTESIAN_POINT('Ctrl Pts',(0.335789970422572,0.727681127006567,
-9.70846081892846));
#59747=CARTESIAN_POINT('Ctrl Pts',(0.455020170159888,0.661680217295637,
-9.71375635175992));
#59748=CARTESIAN_POINT('Ctrl Pts',(0.549357855553091,0.570593759977461,
-9.71905188459139));
#59749=CARTESIAN_POINT('Ctrl Pts',(0.738033226339499,0.388420845341107,
-9.72964295025431));
#59750=CARTESIAN_POINT('Ctrl Pts',(0.827138539749452,0.105905740275768,
-9.74023401591724));
#59751=CARTESIAN_POINT('Ctrl Pts',(0.777335341547127,-0.152006902682922,
-9.75082508158017));
#59752=CARTESIAN_POINT('Ctrl Pts',(0.752433742445964,-0.280963224162265,
-9.75612061441164));
#59753=CARTESIAN_POINT('Ctrl Pts',(0.692805015441732,-0.403768930114946,
-9.76141614724311));
#59754=CARTESIAN_POINT('Ctrl Pts',(0.608399751564134,-0.505177686014364,
-9.76671168007457));
#59755=CARTESIAN_POINT('Ctrl Pts',(0.523994487686536,-0.606586441913781,
-9.77200721290603));
#59756=CARTESIAN_POINT('Ctrl Pts',(0.414812686935571,-0.686598247759937,
-9.77730274573749));
#59757=CARTESIAN_POINT('Ctrl Pts',(0.292940829352205,-0.735113543657704,
-9.78259827856896));
#59758=CARTESIAN_POINT('Ctrl Pts',(0.17106897176884,-0.78362883955547,-9.78789381140042));
#59759=CARTESIAN_POINT('Ctrl Pts',(0.0365070573530715,-0.800647625504847,
-9.79318934423189));
#59760=CARTESIAN_POINT('Ctrl Pts',(-0.0944635525894151,-0.785122939405312,
-9.79848487706336));
#59761=CARTESIAN_POINT('Ctrl Pts',(-0.225434162531902,-0.769598253305778,
-9.80378040989482));
#59762=CARTESIAN_POINT('Ctrl Pts',(-0.352813468001109,-0.721530095157332,
-9.80907594272628));
#59763=CARTESIAN_POINT('Ctrl Pts',(-0.459539163038184,-0.645010690754216,
-9.81437147555775));
#59764=CARTESIAN_POINT('Ctrl Pts',(-0.663062579771367,-0.499089967304251,
-9.82446993343059));
#59765=CARTESIAN_POINT('Ctrl Pts',(-0.791477897958024,-0.249704572895693,
-9.83456839130345));
#59766=CARTESIAN_POINT('Ctrl Pts',(-0.792437169753526,-0.000127296230932911,
-9.8446668491763));
#59767=CARTESIAN_POINT('Ctrl Pts',(-0.791999899124744,0.000522216889476513,
-9.87313315082368));
#59768=CARTESIAN_POINT('Ctrl Pts',(-0.791689945581274,-0.111932488278983,
-9.86859836529019));
#59769=CARTESIAN_POINT('Ctrl Pts',(-0.766202707297937,-0.224882723250992,
-9.8640635797567));
#59770=CARTESIAN_POINT('Ctrl Pts',(-0.719353086501239,-0.327835306675267,
-9.85952879422322));
#59771=CARTESIAN_POINT('Ctrl Pts',(-0.664644059307214,-0.448059026536213,
-9.85423326139175));
#59772=CARTESIAN_POINT('Ctrl Pts',(-0.580804024138859,-0.554649357575498,
-9.84893772856028));
#59773=CARTESIAN_POINT('Ctrl Pts',(-0.475816889973955,-0.633101509454781,
-9.84364219572882));
#59774=CARTESIAN_POINT('Ctrl Pts',(-0.26584262164415,-0.790005813213344,
-9.83305113006589));
#59775=CARTESIAN_POINT('Ctrl Pts',(0.0287200426718578,-0.834357400331918,
-9.82246006440296));
#59776=CARTESIAN_POINT('Ctrl Pts',(0.274399357588069,-0.743640873424784,
-9.81186899874004));
#59777=CARTESIAN_POINT('Ctrl Pts',(0.520078672504281,-0.652924346517651,
-9.80127793307711));
#59778=CARTESIAN_POINT('Ctrl Pts',(0.716874638020693,-0.42713970558481,
-9.79068686741418));
#59779=CARTESIAN_POINT('Ctrl Pts',(0.773699372663501,-0.171584690695658,
-9.78009580175124));
#59780=CARTESIAN_POINT('Ctrl Pts',(0.830524107306308,0.0839703241934938,
-9.76950473608831));
#59781=CARTESIAN_POINT('Ctrl Pts',(0.747377611075511,0.369295713038955,
-9.75891367042538));
#59782=CARTESIAN_POINT('Ctrl Pts',(0.563327148374181,0.556666468774327,
-9.74832260476246));
#59783=CARTESIAN_POINT('Ctrl Pts',(0.471301917023517,0.650351846642012,
-9.743027071931));
#59784=CARTESIAN_POINT('Ctrl Pts',(0.354050694055216,0.719548566232178,
-9.73773153909954));
#59785=CARTESIAN_POINT('Ctrl Pts',(0.227681461481029,0.757299508019194,
-9.73243600626807));
#59786=CARTESIAN_POINT('Ctrl Pts',(0.101312228906838,0.795050449806211,
-9.7271404734366));
#59787=CARTESIAN_POINT('Ctrl Pts',(-0.0341750132732382,0.80135561379008,
-9.72184494060513));
#59788=CARTESIAN_POINT('Ctrl Pts',(-0.162560500119688,0.774454863353173,
-9.71654940777367));
#59789=CARTESIAN_POINT('Ctrl Pts',(-0.290945986966133,0.747554112916268,
-9.7112538749422));
#59790=CARTESIAN_POINT('Ctrl Pts',(-0.412229718478951,0.687447448058585,
-9.70595834211075));
#59791=CARTESIAN_POINT('Ctrl Pts',(-0.512772535588132,0.602012523870264,
-9.70066280927928));
#59792=CARTESIAN_POINT('Ctrl Pts',(-0.613315352697312,0.516577599681943,
-9.69536727644782));
#59793=CARTESIAN_POINT('Ctrl Pts',(-0.693117255402863,0.405814416162977,
-9.69007174361635));
#59794=CARTESIAN_POINT('Ctrl Pts',(-0.739760880099864,0.283037403809672,
-9.68477621078488));
#59795=CARTESIAN_POINT('Ctrl Pts',(-0.77394532300293,0.193055894099291,
-9.68089519079781));
#59796=CARTESIAN_POINT('Ctrl Pts',(-0.790319746311059,0.0966215002284446,
-9.67701417081074));
#59797=CARTESIAN_POINT('Ctrl Pts',(-0.7897370361882,0.00012310453410933,
-9.67313315082366));
#59798=CARTESIAN_POINT('Origin',(0.,0.,-5.925));
#59799=CARTESIAN_POINT('',(-0.790129111244616,-0.000602373567983761,-9.44466684917629));
#59800=CARTESIAN_POINT('',(-0.791100127608287,-3.17057992569413E-5,-9.47313315082365));
#59801=CARTESIAN_POINT('',(-0.7911,-9.68818082805471E-17,-5.925));
#59802=CARTESIAN_POINT('Ctrl Pts',(-0.790129111244616,-0.00060237356798376,
-9.44466684917629));
#59803=CARTESIAN_POINT('Ctrl Pts',(-0.78877350216917,0.166988129555797,
-9.45140000234455));
#59804=CARTESIAN_POINT('Ctrl Pts',(-0.736146428833839,0.335184335378372,
-9.45813315551282));
#59805=CARTESIAN_POINT('Ctrl Pts',(-0.637699246421988,0.469636992975678,
-9.46486630868108));
#59806=CARTESIAN_POINT('Ctrl Pts',(-0.560271884590339,0.575382168347607,
-9.47016184151255));
#59807=CARTESIAN_POINT('Ctrl Pts',(-0.454502002845351,0.660254910048017,
-9.47545737434402));
#59808=CARTESIAN_POINT('Ctrl Pts',(-0.334816055928803,0.716130616615437,
-9.48075290717549));
#59809=CARTESIAN_POINT('Ctrl Pts',(-0.215130109012256,0.772006323182857,
-9.48604844000695));
#59810=CARTESIAN_POINT('Ctrl Pts',(-0.0815280969241502,0.798884994617287,
-9.49134397283841));
#59811=CARTESIAN_POINT('Ctrl Pts',(0.0493402593592206,0.790529462568899,
-9.49663950566987));
#59812=CARTESIAN_POINT('Ctrl Pts',(0.311076971925962,0.773818398472124,
-9.5072305713328));
#59813=CARTESIAN_POINT('Ctrl Pts',(0.561879061273764,0.616170520444079,
-9.51782163699574));
#59814=CARTESIAN_POINT('Ctrl Pts',(0.690879895303411,0.387351651535129,
-9.52841270265866));
#59815=CARTESIAN_POINT('Ctrl Pts',(0.755380312318234,0.272942217080654,
-9.53370823549013));
#59816=CARTESIAN_POINT('Ctrl Pts',(0.789430415503518,0.140740034905953,
-9.53900376832159));
#59817=CARTESIAN_POINT('Ctrl Pts',(0.7907447023627,0.00880726038284042,
-9.54429930115306));
#59818=CARTESIAN_POINT('Ctrl Pts',(0.792058989221882,-0.123125514140272,
-9.54959483398452));
#59819=CARTESIAN_POINT('Ctrl Pts',(0.760637459754962,-0.254788881011797,
-9.55489036681599));
#59820=CARTESIAN_POINT('Ctrl Pts',(0.699154343482463,-0.370660836291279,
-9.56018589964745));
#59821=CARTESIAN_POINT('Ctrl Pts',(0.637671227209964,-0.486532791570762,
-9.56548143247892));
#59822=CARTESIAN_POINT('Ctrl Pts',(0.546126524131887,-0.586613335258203,
-9.57077696531037));
#59823=CARTESIAN_POINT('Ctrl Pts',(0.43625198486056,-0.659564703765652,
-9.57607249814184));
#59824=CARTESIAN_POINT('Ctrl Pts',(0.326377445589232,-0.732516072273101,
-9.58136803097331));
#59825=CARTESIAN_POINT('Ctrl Pts',(0.198173070124655,-0.778338265600559,
-9.58666356380478));
#59826=CARTESIAN_POINT('Ctrl Pts',(0.0672927036574521,-0.789105015563541,
-9.59195909663625));
#59827=CARTESIAN_POINT('Ctrl Pts',(-0.194468029276953,-0.810638515489503,
-9.60255016229918));
#59828=CARTESIAN_POINT('Ctrl Pts',(-0.466932726221856,-0.691950241957559,
-9.61314122796209));
#59829=CARTESIAN_POINT('Ctrl Pts',(-0.626951517257354,-0.484751297419327,
-9.62373229362501));
#59830=CARTESIAN_POINT('Ctrl Pts',(-0.732383849778435,-0.348233155536065,
-9.63071047880877));
#59831=CARTESIAN_POINT('Ctrl Pts',(-0.78900163037992,-0.173291126981858,
-9.63768866399253));
#59832=CARTESIAN_POINT('Ctrl Pts',(-0.790332566743882,0.00078097778472147,
-9.6446668491763));
#59833=CARTESIAN_POINT('Ctrl Pts',(-0.7911,-5.95412608106471E-13,-9.67313315082367));
#59834=CARTESIAN_POINT('Ctrl Pts',(-0.791099999999834,-0.220167589667271,
-9.6642744072504));
#59835=CARTESIAN_POINT('Ctrl Pts',(-0.694214576672042,-0.438610418339204,
-9.65541566367713));
#59836=CARTESIAN_POINT('Ctrl Pts',(-0.531017389079889,-0.586395551223556,
-9.64655692010385));
#59837=CARTESIAN_POINT('Ctrl Pts',(-0.367820201487736,-0.734180684107907,
-9.63769817653058));
#59838=CARTESIAN_POINT('Ctrl Pts',(-0.140868175871139,-0.808992666571442,
-9.62883943295731));
#59839=CARTESIAN_POINT('Ctrl Pts',(0.0782205473253529,-0.787223447298238,
-9.61998068938404));
#59840=CARTESIAN_POINT('Ctrl Pts',(0.297309270521845,-0.765454228025035,
-9.61112194581076));
#59841=CARTESIAN_POINT('Ctrl Pts',(0.505102072676084,-0.647444880833849,
-9.60226320223749));
#59842=CARTESIAN_POINT('Ctrl Pts',(0.636026795762087,-0.470435038100494,
-9.59340445866422));
#59843=CARTESIAN_POINT('Ctrl Pts',(0.766951518848089,-0.293425195367138,
-9.58454571509095));
#59844=CARTESIAN_POINT('Ctrl Pts',(0.818956872247116,-0.0601881960093101,
-9.57568697151767));
#59845=CARTESIAN_POINT('Ctrl Pts',(0.775631781004092,0.15567450111184,-9.5668282279444));
#59846=CARTESIAN_POINT('Ctrl Pts',(0.732306689761068,0.37153719823299,-9.55796948437113));
#59847=CARTESIAN_POINT('Ctrl Pts',(0.594329958849784,0.566643518936949,
-9.54911074079786));
#59848=CARTESIAN_POINT('Ctrl Pts',(0.405242230243525,0.679424716085053,
-9.54025199722458));
#59849=CARTESIAN_POINT('Ctrl Pts',(0.216154501637265,0.792205913233156,
-9.53139325365131));
#59850=CARTESIAN_POINT('Ctrl Pts',(-0.0210816529306389,0.820894963712987,
-9.52253451007804));
#59851=CARTESIAN_POINT('Ctrl Pts',(-0.231602780753791,0.756438604215247,
-9.51367576650476));
#59852=CARTESIAN_POINT('Ctrl Pts',(-0.442123908576943,0.691982244717508,
-9.50481702293149));
#59853=CARTESIAN_POINT('Ctrl Pts',(-0.622631625634579,0.535390358803066,
-9.49595827935822));
#59854=CARTESIAN_POINT('Ctrl Pts',(-0.716163994722408,0.336077881841758,
-9.48709953578495));
#59855=CARTESIAN_POINT('Ctrl Pts',(-0.765317280859656,0.231334857513964,
-9.48244407413119));
#59856=CARTESIAN_POINT('Ctrl Pts',(-0.791100000000083,0.115702837835949,
-9.47778861247743));
#59857=CARTESIAN_POINT('Ctrl Pts',(-0.7911,-5.67157432129761E-13,-9.47313315082367));
#59858=CARTESIAN_POINT('Origin',(0.,0.,-5.925));
#59859=CARTESIAN_POINT('',(-0.791985506391904,-0.000137013821822907,-9.2446668491763));
#59860=CARTESIAN_POINT('',(-0.791291464171058,-0.000172660802811795,-9.27313315082367));
#59861=CARTESIAN_POINT('',(-0.7911,-9.68818082805471E-17,-5.925));
#59862=CARTESIAN_POINT('Ctrl Pts',(-0.791985506391904,-0.000137013821822907,
-9.2446668491763));
#59863=CARTESIAN_POINT('Ctrl Pts',(-0.791786526522987,0.112700469452395,
-9.24922474220219));
#59864=CARTESIAN_POINT('Ctrl Pts',(-0.766166379387017,0.225741947610222,
-9.25378263522809));
#59865=CARTESIAN_POINT('Ctrl Pts',(-0.718782612796448,0.329084194247059,
-9.25834052825398));
#59866=CARTESIAN_POINT('Ctrl Pts',(-0.663730357240334,0.449151132377018,
-9.26363606108544));
#59867=CARTESIAN_POINT('Ctrl Pts',(-0.579300103659578,0.556125395133812,
-9.2689315939169));
#59868=CARTESIAN_POINT('Ctrl Pts',(-0.474144470433553,0.634474832866043,
-9.27422712674836));
#59869=CARTESIAN_POINT('Ctrl Pts',(-0.263833203981505,0.791173708330505,
-9.28481819241128));
#59870=CARTESIAN_POINT('Ctrl Pts',(0.0293795810516175,0.833373283696715,
-9.29540925807423));
#59871=CARTESIAN_POINT('Ctrl Pts',(0.27582928125095,0.742478645676782,-9.30600032373715));
#59872=CARTESIAN_POINT('Ctrl Pts',(0.399054131350617,0.697031326666815,
-9.31129585656862));
#59873=CARTESIAN_POINT('Ctrl Pts',(0.510588210241836,0.618310454310313,
-9.31659138940007));
#59874=CARTESIAN_POINT('Ctrl Pts',(0.596996948867665,0.518603311976337,
-9.32188692223154));
#59875=CARTESIAN_POINT('Ctrl Pts',(0.683405687493494,0.41889616964236,-9.327182455063));
#59876=CARTESIAN_POINT('Ctrl Pts',(0.744689085853934,0.298202757330909,
-9.33247798789447));
#59877=CARTESIAN_POINT('Ctrl Pts',(0.772837210270715,0.170084972856288,
-9.33777352072594));
#59878=CARTESIAN_POINT('Ctrl Pts',(0.800985334687495,0.0419671883816674,
-9.34306905355741));
#59879=CARTESIAN_POINT('Ctrl Pts',(0.795998185160616,-0.0935749682561238,
-9.34836458638886));
#59880=CARTESIAN_POINT('Ctrl Pts',(0.759478065537175,-0.220305380588309,
-9.35366011922033));
#59881=CARTESIAN_POINT('Ctrl Pts',(0.722957945913735,-0.347035792920495,
-9.35895565205179));
#59882=CARTESIAN_POINT('Ctrl Pts',(0.654904856193732,-0.464954460947075,
-9.36425118488326));
#59883=CARTESIAN_POINT('Ctrl Pts',(0.562118924507943,-0.557886501237572,
-9.36954671771473));
#59884=CARTESIAN_POINT('Ctrl Pts',(0.376547061136364,-0.743750581818566,
-9.38013778337766));
#59885=CARTESIAN_POINT('Ctrl Pts',(0.0920438299016367,-0.82966815145523,
-9.39072884904058));
#59886=CARTESIAN_POINT('Ctrl Pts',(-0.164051761844405,-0.775331570862921,
-9.40131991470351));
#59887=CARTESIAN_POINT('Ctrl Pts',(-0.420147353590447,-0.720994990270612,
-9.41191098036644));
#59888=CARTESIAN_POINT('Ctrl Pts',(-0.647835305847804,-0.52640425944933,
-9.42250204602937));
#59889=CARTESIAN_POINT('Ctrl Pts',(-0.740936959971514,-0.281618851323722,
-9.4330931116923));
#59890=CARTESIAN_POINT('Ctrl Pts',(-0.774850264463147,-0.192453066257844,
-9.43695102418697));
#59891=CARTESIAN_POINT('Ctrl Pts',(-0.790905838144978,-0.0966271452954019,
-9.44080893668163));
#59892=CARTESIAN_POINT('Ctrl Pts',(-0.790129111244616,-0.00060237356798376,
-9.44466684917629));
#59893=CARTESIAN_POINT('Ctrl Pts',(-0.791100561757637,-0.000139575345601312,
-9.47313315082367));
#59894=CARTESIAN_POINT('Ctrl Pts',(-0.791433680411738,-0.0896913779101309,
-9.46954337783691));
#59895=CARTESIAN_POINT('Ctrl Pts',(-0.776842562758261,-0.17925244583268,
-9.46595360485014));
#59896=CARTESIAN_POINT('Ctrl Pts',(-0.747063898241547,-0.263157488256723,
-9.46236383186337));
#59897=CARTESIAN_POINT('Ctrl Pts',(-0.659206590157331,-0.510706237729051,
-9.45177276620044));
#59898=CARTESIAN_POINT('Ctrl Pts',(-0.439148817318704,-0.709021940791804,
-9.44118170053751));
#59899=CARTESIAN_POINT('Ctrl Pts',(-0.184153391517759,-0.770362785170478,
-9.43059063487458));
#59900=CARTESIAN_POINT('Ctrl Pts',(-0.0566556786172914,-0.801033207359814,
-9.42529510204312));
#59901=CARTESIAN_POINT('Ctrl Pts',(0.0795764475237638,-0.797459914878131,
-9.41999956921166));
#59902=CARTESIAN_POINT('Ctrl Pts',(0.20707040698932,-0.762932957677804,
-9.41470403638019));
#59903=CARTESIAN_POINT('Ctrl Pts',(0.334564366454881,-0.728406000477477,
-9.40940850354873));
#59904=CARTESIAN_POINT('Ctrl Pts',(0.453320159244951,-0.662925378558506,
-9.40411297071726));
#59905=CARTESIAN_POINT('Ctrl Pts',(0.547731929316479,-0.572021824466215,
-9.3988174378858));
#59906=CARTESIAN_POINT('Ctrl Pts',(0.736555469459537,-0.390214716281634,
-9.38822637222287));
#59907=CARTESIAN_POINT('Ctrl Pts',(0.828002918728424,-0.106715879403781,
-9.37763530655994));
#59908=CARTESIAN_POINT('Ctrl Pts',(0.778250780715013,0.150407707213407,
-9.36704424089701));
#59909=CARTESIAN_POINT('Ctrl Pts',(0.728498642701604,0.407531293830588,
-9.35645317523408));
#59910=CARTESIAN_POINT('Ctrl Pts',(0.537546917405906,0.638279630187101,
-9.34586210957115));
#59911=CARTESIAN_POINT('Ctrl Pts',(0.294560327079297,0.735721577128167,
-9.33527104390822));
#59912=CARTESIAN_POINT('Ctrl Pts',(0.051573736752682,0.833163524069235,
-9.32467997824529));
#59913=CARTESIAN_POINT('Ctrl Pts',(-0.243447718604854,0.797299081594843,
-9.31408891258236));
#59914=CARTESIAN_POINT('Ctrl Pts',(-0.458139645376263,0.646005494471663,
-9.30349784691943));
#59915=CARTESIAN_POINT('Ctrl Pts',(-0.565485608761967,0.570358700910073,
-9.29820231408797));
#59916=CARTESIAN_POINT('Ctrl Pts',(-0.65274919000114,0.465854621186288,
-9.29290678125651));
#59917=CARTESIAN_POINT('Ctrl Pts',(-0.710457625152268,0.347262660836506,
-9.28761124842504));
#59918=CARTESIAN_POINT('Ctrl Pts',(-0.763049648349371,0.239185026893182,
-9.28278521589125));
#59919=CARTESIAN_POINT('Ctrl Pts',(-0.791094906196155,0.119406828216415,
-9.27795918335746));
#59920=CARTESIAN_POINT('Ctrl Pts',(-0.791291464171058,-0.000172660802811794,
-9.27313315082367));
#59921=CARTESIAN_POINT('Origin',(0.,0.,-5.925));
#59922=CARTESIAN_POINT('',(-0.791150637177402,0.000157610601749369,-9.0446668491763));
#59923=CARTESIAN_POINT('',(-0.791456073972705,0.000283146808428445,-9.07313315082367));
#59924=CARTESIAN_POINT('',(-0.7911,-9.68818082805471E-17,-5.925));
#59925=CARTESIAN_POINT('Ctrl Pts',(-0.791308228660122,0.000648121520882616,
-9.0446668491763));
#59926=CARTESIAN_POINT('Ctrl Pts',(-0.791650333819295,0.0599578818431041,
-9.04704948205981));
#59927=CARTESIAN_POINT('Ctrl Pts',(-0.785358429788104,0.119155442284125,
-9.04943211494333));
#59928=CARTESIAN_POINT('Ctrl Pts',(-0.772117381331553,0.176652319058692,
-9.05181474782685));
#59929=CARTESIAN_POINT('Ctrl Pts',(-0.713259462170178,0.432232270777294,
-9.06240581348978));
#59930=CARTESIAN_POINT('Ctrl Pts',(-0.51709336754244,0.654208406401072,
-9.07299687915271));
#59931=CARTESIAN_POINT('Ctrl Pts',(-0.270410805205285,0.744469158602069,
-9.08358794481564));
#59932=CARTESIAN_POINT('Ctrl Pts',(-0.147069524036703,0.78959953470257,
-9.0888834776471));
#59933=CARTESIAN_POINT('Ctrl Pts',(-0.0110991259407661,0.801801064947372,
-9.09417901047857));
#59934=CARTESIAN_POINT('Ctrl Pts',(0.119306481265527,0.781742103048164,
-9.09947454331003));
#59935=CARTESIAN_POINT('Ctrl Pts',(0.249712088471816,0.761683141148956,
-9.1047700761415));
#59936=CARTESIAN_POINT('Ctrl Pts',(0.37455290478846,0.709363687105741,-9.11006560897296));
#59937=CARTESIAN_POINT('Ctrl Pts',(0.478944504916685,0.629935244910663,
-9.11536114180442));
#59938=CARTESIAN_POINT('Ctrl Pts',(0.583336105044909,0.550506802715584,
-9.12065667463589));
#59939=CARTESIAN_POINT('Ctrl Pts',(0.667278488984713,0.443969372368644,
-9.12595220746735));
#59940=CARTESIAN_POINT('Ctrl Pts',(0.72148242867828,0.323735228013172,-9.13124774029882));
#59941=CARTESIAN_POINT('Ctrl Pts',(0.775686368371847,0.2035010836577,-9.13654327313028));
#59942=CARTESIAN_POINT('Ctrl Pts',(0.800151863819177,0.0695702252936993,
-9.14183880596175));
#59943=CARTESIAN_POINT('Ctrl Pts',(0.789591060252161,-0.061326920050932,
-9.14713433879322));
#59944=CARTESIAN_POINT('Ctrl Pts',(0.768469453118131,-0.323121210740191,
-9.15772540445615));
#59945=CARTESIAN_POINT('Ctrl Pts',(0.60724264992672,-0.572780649351978,
-9.16831647011907));
#59946=CARTESIAN_POINT('Ctrl Pts',(0.376874024690652,-0.697149908451897,
-9.178907535782));
#59947=CARTESIAN_POINT('Ctrl Pts',(0.146505399454581,-0.821519167551817,
-9.18949860144492));
#59948=CARTESIAN_POINT('Ctrl Pts',(-0.153005047826149,-0.820598247139874,
-9.20008966710786));
#59949=CARTESIAN_POINT('Ctrl Pts',(-0.382428700634536,-0.694294638466769,
-9.21068073277079));
#59950=CARTESIAN_POINT('Ctrl Pts',(-0.611852353442922,-0.567991029793665,
-9.22127179843372));
#59951=CARTESIAN_POINT('Ctrl Pts',(-0.771189211778961,-0.316304732859401,
-9.23186286409664));
#59952=CARTESIAN_POINT('Ctrl Pts',(-0.790069154515677,-0.0548631492104814,
-9.24245392975957));
#59953=CARTESIAN_POINT('Ctrl Pts',(-0.791384092760116,-0.0366544320644326,
-9.24319156956515));
#59954=CARTESIAN_POINT('Ctrl Pts',(-0.792017708874715,-0.0183983944095057,
-9.24392920937072));
#59955=CARTESIAN_POINT('Ctrl Pts',(-0.791985506391904,-0.000137013821822907,
-9.2446668491763));
#59956=CARTESIAN_POINT('Ctrl Pts',(-0.791291464171058,-0.000172660802811794,
-9.27313315082367));
#59957=CARTESIAN_POINT('Ctrl Pts',(-0.79131058630235,-0.0118059445192655,
-9.27266365052599));
#59958=CARTESIAN_POINT('Ctrl Pts',(-0.791066138311347,-0.0234373475759765,
-9.27219415022832));
#59959=CARTESIAN_POINT('Ctrl Pts',(-0.790555079975775,-0.035055913838341,
-9.27172464993064));
#59960=CARTESIAN_POINT('Ctrl Pts',(-0.784790810585072,-0.166102687187628,
-9.26642911709918));
#59961=CARTESIAN_POINT('Ctrl Pts',(-0.745108982740585,-0.295516392910425,
-9.26113358426772));
#59962=CARTESIAN_POINT('Ctrl Pts',(-0.67707559581834,-0.408562589693877,
-9.25583805143626));
#59963=CARTESIAN_POINT('Ctrl Pts',(-0.609042208896096,-0.521608786477329,
-9.25054251860479));
#59964=CARTESIAN_POINT('Ctrl Pts',(-0.512657262896095,-0.618287474321436,
-9.24524698577332));
#59965=CARTESIAN_POINT('Ctrl Pts',(-0.399049604828334,-0.684189845414118,
-9.23995145294186));
#59966=CARTESIAN_POINT('Ctrl Pts',(-0.171834288692815,-0.815994587599481,
-9.22936038727893));
#59967=CARTESIAN_POINT('Ctrl Pts',(0.124271875713755,-0.824694062779146,
-9.21876932161601));
#59968=CARTESIAN_POINT('Ctrl Pts',(0.358336191702969,-0.706375584302658,
-9.20817825595308));
#59969=CARTESIAN_POINT('Ctrl Pts',(0.475368349697578,-0.647216345064414,
-9.20288272312161));
#59970=CARTESIAN_POINT('Ctrl Pts',(0.57689004558785,-0.55630261741213,-9.19758719029014));
#59971=CARTESIAN_POINT('Ctrl Pts',(0.651713661232107,-0.447452964148376,
-9.19229165745868));
#59972=CARTESIAN_POINT('Ctrl Pts',(0.726537276876364,-0.338603310884622,
-9.18699612462721));
#59973=CARTESIAN_POINT('Ctrl Pts',(0.774662812274606,-0.211817732009396,
-9.18170059179575));
#59974=CARTESIAN_POINT('Ctrl Pts',(0.787775960383391,-0.0814141897978206,
-9.17640505896428));
#59975=CARTESIAN_POINT('Ctrl Pts',(0.814002256600962,0.179392894625334,
-9.16581399330136));
#59976=CARTESIAN_POINT('Ctrl Pts',(0.700179003660705,0.454671832393888,
-9.15522292763843));
#59977=CARTESIAN_POINT('Ctrl Pts',(0.495808804183578,0.61844190169067,-9.1446318619755));
#59978=CARTESIAN_POINT('Ctrl Pts',(0.291438604706456,0.782211970987448,
-9.13404079631256));
#59979=CARTESIAN_POINT('Ctrl Pts',(-0.00347854130752701,0.83447317181246,
-9.12344973064964));
#59980=CARTESIAN_POINT('Ctrl Pts',(-0.251759969397478,0.751444570909924,
-9.11285866498671));
#59981=CARTESIAN_POINT('Ctrl Pts',(-0.500041397487433,0.668415970007387,
-9.10226759932378));
#59982=CARTESIAN_POINT('Ctrl Pts',(-0.701687107653353,0.450097567377298,
-9.09167653366085));
#59983=CARTESIAN_POINT('Ctrl Pts',(-0.767383052384056,0.195801645720345,
-9.08108546799792));
#59984=CARTESIAN_POINT('Ctrl Pts',(-0.783825684510273,0.132155490571162,
-9.07843469560651));
#59985=CARTESIAN_POINT('Ctrl Pts',(-0.791752152589477,0.0662556319819147,
-9.07578392321509));
#59986=CARTESIAN_POINT('Ctrl Pts',(-0.791456073972705,0.000283146808428445,
-9.07313315082367));
#59987=CARTESIAN_POINT('Origin',(0.,0.,-5.925));
#59988=CARTESIAN_POINT('',(-0.7911,-5.02375918642883E-14,-8.84466684917629));
#59989=CARTESIAN_POINT('',(-0.790337230870817,0.000108444134415879,-8.87313315082367));
#59990=CARTESIAN_POINT('',(-0.7911,-9.68818082805471E-17,-5.925));
#59991=CARTESIAN_POINT('Ctrl Pts',(-0.7911,-3.90243393155743E-14,-8.84466684917629));
#59992=CARTESIAN_POINT('Ctrl Pts',(-0.791100000000011,0.220167589666633,
-8.85352559274957));
#59993=CARTESIAN_POINT('Ctrl Pts',(-0.694214576672397,0.43861041833864,
-8.86238433632284));
#59994=CARTESIAN_POINT('Ctrl Pts',(-0.531017389080368,0.586395551223122,
-8.87124307989611));
#59995=CARTESIAN_POINT('Ctrl Pts',(-0.367820201488338,0.734180684107605,
-8.88010182346938));
#59996=CARTESIAN_POINT('Ctrl Pts',(-0.140868175871807,0.808992666571324,
-8.88896056704266));
#59997=CARTESIAN_POINT('Ctrl Pts',(0.0782205473246991,0.787223447298303,
-8.89781931061593));
#59998=CARTESIAN_POINT('Ctrl Pts',(0.297309270521205,0.765454228025282,
-8.9066780541892));
#59999=CARTESIAN_POINT('Ctrl Pts',(0.50510207267554,0.647444880834273,-8.91553679776247));
#60000=CARTESIAN_POINT('Ctrl Pts',(0.636026795761689,0.470435038101031,
-8.92439554133574));
#60001=CARTESIAN_POINT('Ctrl Pts',(0.766951518847839,0.293425195367788,
-8.93325428490902));
#60002=CARTESIAN_POINT('Ctrl Pts',(0.818956872247063,0.0601881960100098,
-8.94211302848229));
#60003=CARTESIAN_POINT('Ctrl Pts',(0.775631781004226,-0.155674501111174,
-8.95097177205556));
#60004=CARTESIAN_POINT('Ctrl Pts',(0.732306689761388,-0.371537198232358,
-8.95983051562884));
#60005=CARTESIAN_POINT('Ctrl Pts',(0.594329958850275,-0.566643518936432,
-8.96868925920211));
#60006=CARTESIAN_POINT('Ctrl Pts',(0.405242230244118,-0.679424716084699,
-8.97754800277538));
#60007=CARTESIAN_POINT('Ctrl Pts',(0.21615450163796,-0.792205913232966,
-8.98640674634865));
#60008=CARTESIAN_POINT('Ctrl Pts',(-0.0210816529299142,-0.820894963713004,
-8.99526548992193));
#60009=CARTESIAN_POINT('Ctrl Pts',(-0.23160278075312,-0.756438604215453,
-9.0041242334952));
#60010=CARTESIAN_POINT('Ctrl Pts',(-0.442123908576326,-0.691982244717901,
-9.01298297706847));
#60011=CARTESIAN_POINT('Ctrl Pts',(-0.622631625634097,-0.535390358803624,
-9.02184172064174));
#60012=CARTESIAN_POINT('Ctrl Pts',(-0.716163994722105,-0.336077881842404,
-9.03070046421501));
#60013=CARTESIAN_POINT('Ctrl Pts',(-0.765317280859466,-0.231334857514613,
-9.03535592586877));
#60014=CARTESIAN_POINT('Ctrl Pts',(-0.791099999999998,-0.115702837836572,
-9.04001138752253));
#60015=CARTESIAN_POINT('Ctrl Pts',(-0.7911,-1.11022302462516E-14,-9.04466684917629));
#60016=CARTESIAN_POINT('Ctrl Pts',(-0.791456073972705,0.000283146808428445,
-9.07313315082367));
#60017=CARTESIAN_POINT('Ctrl Pts',(-0.791160666862189,-0.0655397127790337,
-9.07048839038363));
#60018=CARTESIAN_POINT('Ctrl Pts',(-0.782679968229602,-0.131434869890149,
-9.06784362994358));
#60019=CARTESIAN_POINT('Ctrl Pts',(-0.766305602181184,-0.195236054083216,
-9.06519886950353));
#60020=CARTESIAN_POINT('Ctrl Pts',(-0.73351964860641,-0.322983452473125,
-9.05990333667207));
#60021=CARTESIAN_POINT('Ctrl Pts',(-0.669087210450313,-0.442335908667745,
-9.0546078038406));
#60022=CARTESIAN_POINT('Ctrl Pts',(-0.579860291012648,-0.538487042069976,
-9.04931227100913));
#60023=CARTESIAN_POINT('Ctrl Pts',(-0.490633371574989,-0.634638175472201,
-9.04401673817767));
#60024=CARTESIAN_POINT('Ctrl Pts',(-0.376611970855764,-0.707587986082038,
-9.0387212053462));
#60025=CARTESIAN_POINT('Ctrl Pts',(-0.251576818747605,-0.749709181228937,
-9.03342567251474));
#60026=CARTESIAN_POINT('Ctrl Pts',(-0.126541666639438,-0.791830376375839,
-9.02813013968327));
#60027=CARTESIAN_POINT('Ctrl Pts',(0.00950723685766419,-0.803122956059799,
-9.02283460685182));
#60028=CARTESIAN_POINT('Ctrl Pts',(0.138760010107436,-0.779808945368305,
-9.01753907402035));
#60029=CARTESIAN_POINT('Ctrl Pts',(0.397265556606972,-0.733180923985319,
-9.00694800835743));
#60030=CARTESIAN_POINT('Ctrl Pts',(0.628586582117184,-0.548126541100527,
-8.99635694269448));
#60031=CARTESIAN_POINT('Ctrl Pts',(0.730394500479292,-0.306423181323989,
-8.98576587703155));
#60032=CARTESIAN_POINT('Ctrl Pts',(0.781298459660345,-0.185571501435724,
-8.98047034420009));
#60033=CARTESIAN_POINT('Ctrl Pts',(0.799824142054372,-0.0505575773245239,
-8.97517481136864));
#60034=CARTESIAN_POINT('Ctrl Pts',(0.786389927968675,0.0808438776355248,
-8.96987927853717));
#60035=CARTESIAN_POINT('Ctrl Pts',(0.772955713882977,0.212245332595581,
-8.96458374570571));
#60036=CARTESIAN_POINT('Ctrl Pts',(0.727561603317545,0.340034318404495,
-8.95928821287423));
#60037=CARTESIAN_POINT('Ctrl Pts',(0.65313927536984,0.447915528897771,-8.95399268004277));
#60038=CARTESIAN_POINT('Ctrl Pts',(0.504294619474436,0.663677949884313,
-8.94340161437983));
#60039=CARTESIAN_POINT('Ctrl Pts',(0.239337094049943,0.799809269608347,
-8.93281054871691));
#60040=CARTESIAN_POINT('Ctrl Pts',(-0.0224489462895803,0.792333768612198,
-8.92221948305399));
#60041=CARTESIAN_POINT('Ctrl Pts',(-0.284234986629107,0.78485826761605,
-8.91162841739106));
#60042=CARTESIAN_POINT('Ctrl Pts',(-0.54284954188366,0.633775945899715,
-8.90103735172813));
#60043=CARTESIAN_POINT('Ctrl Pts',(-0.678338600276407,0.409766724754542,
-8.8904462860652));
#60044=CARTESIAN_POINT('Ctrl Pts',(-0.752166247916911,0.287704662746626,
-8.88467524098468));
#60045=CARTESIAN_POINT('Ctrl Pts',(-0.789436301294637,0.14398963633968,
-8.87890419590418));
#60046=CARTESIAN_POINT('Ctrl Pts',(-0.789536508750431,0.000222284108289859,
-8.87313315082367));
#60047=CARTESIAN_POINT('Origin',(0.,0.,-5.925));
#60048=CARTESIAN_POINT('',(-0.7911,-5.56776846849516E-14,-8.64466684917629));
#60049=CARTESIAN_POINT('',(-0.7911,-6.11399819661074E-13,-8.67313315082367));
#60050=CARTESIAN_POINT('',(-0.7911,-9.68818082805471E-17,-5.925));
#60051=CARTESIAN_POINT('Ctrl Pts',(-0.7911,-7.82152120848423E-14,-8.64466684917629));
#60052=CARTESIAN_POINT('Ctrl Pts',(-0.791100000000022,0.220167589666598,
-8.65352559274957));
#60053=CARTESIAN_POINT('Ctrl Pts',(-0.694214576672415,0.438610418338613,
-8.66238433632284));
#60054=CARTESIAN_POINT('Ctrl Pts',(-0.531017389080388,0.586395551223103,
-8.67124307989611));
#60055=CARTESIAN_POINT('Ctrl Pts',(-0.367820201488361,0.734180684107594,
-8.68010182346938));
#60056=CARTESIAN_POINT('Ctrl Pts',(-0.140868175871828,0.808992666571322,
-8.68896056704266));
#60057=CARTESIAN_POINT('Ctrl Pts',(0.0782205473246826,0.787223447298305,
-8.69781931061593));
#60058=CARTESIAN_POINT('Ctrl Pts',(0.297309270521193,0.765454228025288,
-8.7066780541892));
#60059=CARTESIAN_POINT('Ctrl Pts',(0.505102072675533,0.647444880834279,
-8.71553679776247));
#60060=CARTESIAN_POINT('Ctrl Pts',(0.636026795761686,0.470435038101035,
-8.72439554133575));
#60061=CARTESIAN_POINT('Ctrl Pts',(0.766951518847839,0.293425195367791,
-8.73325428490902));
#60062=CARTESIAN_POINT('Ctrl Pts',(0.818956872247065,0.0601881960100074,
-8.74211302848229));
#60063=CARTESIAN_POINT('Ctrl Pts',(0.775631781004225,-0.15567450111118,
-8.75097177205556));
#60064=CARTESIAN_POINT('Ctrl Pts',(0.732306689761385,-0.371537198232367,
-8.75983051562884));
#60065=CARTESIAN_POINT('Ctrl Pts',(0.594329958850266,-0.566643518936443,
-8.76868925920211));
#60066=CARTESIAN_POINT('Ctrl Pts',(0.405242230244103,-0.679424716084707,
-8.77754800277538));
#60067=CARTESIAN_POINT('Ctrl Pts',(0.21615450163794,-0.792205913232972,
-8.78640674634865));
#60068=CARTESIAN_POINT('Ctrl Pts',(-0.02108165292994,-0.820894963713005,
-8.79526548992193));
#60069=CARTESIAN_POINT('Ctrl Pts',(-0.231602780753147,-0.756438604215444,
-8.8041242334952));
#60070=CARTESIAN_POINT('Ctrl Pts',(-0.442123908576354,-0.691982244717884,
-8.81298297706847));
#60071=CARTESIAN_POINT('Ctrl Pts',(-0.622631625634123,-0.535390358803596,
-8.82184172064174));
#60072=CARTESIAN_POINT('Ctrl Pts',(-0.716163994722122,-0.336077881842368,
-8.83070046421502));
#60073=CARTESIAN_POINT('Ctrl Pts',(-0.765317280859468,-0.231334857514595,
-8.83535592586878));
#60074=CARTESIAN_POINT('Ctrl Pts',(-0.791099999999994,-0.115702837836577,
-8.84001138752253));
#60075=CARTESIAN_POINT('Ctrl Pts',(-0.7911,-3.90243393155743E-14,-8.84466684917629));
#60076=CARTESIAN_POINT('Ctrl Pts',(-0.7911,-6.05904215689179E-13,-8.87313315082367));
#60077=CARTESIAN_POINT('Ctrl Pts',(-0.791099999999831,-0.220167589667286,
-8.8642744072504));
#60078=CARTESIAN_POINT('Ctrl Pts',(-0.694214576672033,-0.438610418339221,
-8.85541566367713));
#60079=CARTESIAN_POINT('Ctrl Pts',(-0.531017389079873,-0.58639555122357,
-8.84655692010385));
#60080=CARTESIAN_POINT('Ctrl Pts',(-0.367820201487713,-0.73418068410792,
-8.83769817653058));
#60081=CARTESIAN_POINT('Ctrl Pts',(-0.140868175871109,-0.808992666571448,
-8.82883943295731));
#60082=CARTESIAN_POINT('Ctrl Pts',(0.0782205473253857,-0.787223447298235,
-8.81998068938404));
#60083=CARTESIAN_POINT('Ctrl Pts',(0.29730927052188,-0.765454228025022,
-8.81112194581076));
#60084=CARTESIAN_POINT('Ctrl Pts',(0.505102072676118,-0.647444880833824,
-8.80226320223749));
#60085=CARTESIAN_POINT('Ctrl Pts',(0.636026795762113,-0.470435038100458,
-8.79340445866422));
#60086=CARTESIAN_POINT('Ctrl Pts',(0.766951518848108,-0.293425195367092,
-8.78454571509094));
#60087=CARTESIAN_POINT('Ctrl Pts',(0.818956872247121,-0.0601881960092564,
-8.77568697151767));
#60088=CARTESIAN_POINT('Ctrl Pts',(0.775631781004081,0.155674501111895,
-8.7668282279444));
#60089=CARTESIAN_POINT('Ctrl Pts',(0.732306689761042,0.371537198233045,
-8.75796948437113));
#60090=CARTESIAN_POINT('Ctrl Pts',(0.594329958849739,0.566643518936997,
-8.74911074079785));
#60091=CARTESIAN_POINT('Ctrl Pts',(0.405242230243467,0.679424716085087,
-8.74025199722458));
#60092=CARTESIAN_POINT('Ctrl Pts',(0.216154501637195,0.792205913233177,
-8.73139325365131));
#60093=CARTESIAN_POINT('Ctrl Pts',(-0.0210816529307163,0.820894963712986,
-8.72253451007803));
#60094=CARTESIAN_POINT('Ctrl Pts',(-0.231602780753866,0.756438604215224,
-8.71367576650476));
#60095=CARTESIAN_POINT('Ctrl Pts',(-0.442123908577015,0.691982244717463,
-8.70481702293149));
#60096=CARTESIAN_POINT('Ctrl Pts',(-0.622631625634637,0.535390358802999,
-8.69595827935822));
#60097=CARTESIAN_POINT('Ctrl Pts',(-0.716163994722446,0.336077881841678,
-8.68709953578495));
#60098=CARTESIAN_POINT('Ctrl Pts',(-0.765317280859677,0.231334857513888,
-8.68244407413119));
#60099=CARTESIAN_POINT('Ctrl Pts',(-0.791100000000091,0.115702837835882,
-8.67778861247743));
#60100=CARTESIAN_POINT('Ctrl Pts',(-0.7911,-6.22557561058557E-13,-8.67313315082367));
#60101=CARTESIAN_POINT('Origin',(0.,0.,-5.925));
#60102=CARTESIAN_POINT('',(-0.7911,-6.11177775056149E-14,-8.44466684917629));
#60103=CARTESIAN_POINT('',(-0.791450958846291,0.000332134113033131,-8.47313315082367));
#60104=CARTESIAN_POINT('',(-0.7911,-9.68818082805471E-17,-5.925));
#60105=CARTESIAN_POINT('Ctrl Pts',(-0.7911,-6.11177775056149E-14,-8.44466684917629));
#60106=CARTESIAN_POINT('Ctrl Pts',(-0.791100000000017,0.220167589666615,
-8.45352559274957));
#60107=CARTESIAN_POINT('Ctrl Pts',(-0.694214576672406,0.438610418338628,
-8.46238433632284));
#60108=CARTESIAN_POINT('Ctrl Pts',(-0.531017389080376,0.586395551223115,
-8.47124307989611));
#60109=CARTESIAN_POINT('Ctrl Pts',(-0.367820201488346,0.734180684107602,
-8.48010182346938));
#60110=CARTESIAN_POINT('Ctrl Pts',(-0.14086817587181,0.808992666571325,
-8.48896056704266));
#60111=CARTESIAN_POINT('Ctrl Pts',(0.0782205473246995,0.787223447298303,
-8.49781931061593));
#60112=CARTESIAN_POINT('Ctrl Pts',(0.297309270521209,0.765454228025282,
-8.5066780541892));
#60113=CARTESIAN_POINT('Ctrl Pts',(0.505102072675547,0.647444880834269,
-8.51553679776247));
#60114=CARTESIAN_POINT('Ctrl Pts',(0.636026795761696,0.470435038101021,
-8.52439554133575));
#60115=CARTESIAN_POINT('Ctrl Pts',(0.766951518847846,0.293425195367774,
-8.53325428490902));
#60116=CARTESIAN_POINT('Ctrl Pts',(0.818956872247066,0.0601881960099898,
-8.54211302848229));
#60117=CARTESIAN_POINT('Ctrl Pts',(0.775631781004221,-0.155674501111196,
-8.55097177205556));
#60118=CARTESIAN_POINT('Ctrl Pts',(0.732306689761376,-0.371537198232383,
-8.55983051562884));
#60119=CARTESIAN_POINT('Ctrl Pts',(0.594329958850254,-0.566643518936455,
-8.56868925920211));
#60120=CARTESIAN_POINT('Ctrl Pts',(0.405242230244088,-0.679424716084716,
-8.57754800277538));
#60121=CARTESIAN_POINT('Ctrl Pts',(0.216154501637923,-0.792205913232977,
-8.58640674634865));
#60122=CARTESIAN_POINT('Ctrl Pts',(-0.0210816529299578,-0.820894963713004,
-8.59526548992193));
#60123=CARTESIAN_POINT('Ctrl Pts',(-0.231602780753163,-0.756438604215439,
-8.6041242334952));
#60124=CARTESIAN_POINT('Ctrl Pts',(-0.442123908576369,-0.691982244717875,
-8.61298297706847));
#60125=CARTESIAN_POINT('Ctrl Pts',(-0.622631625634134,-0.535390358803583,
-8.62184172064175));
#60126=CARTESIAN_POINT('Ctrl Pts',(-0.716163994722129,-0.336077881842353,
-8.63070046421502));
#60127=CARTESIAN_POINT('Ctrl Pts',(-0.765317280859465,-0.231334857514596,
-8.63535592586878));
#60128=CARTESIAN_POINT('Ctrl Pts',(-0.791099999999989,-0.115702837836598,
-8.64001138752253));
#60129=CARTESIAN_POINT('Ctrl Pts',(-0.7911,-7.82152120848423E-14,-8.64466684917629));
#60130=CARTESIAN_POINT('Ctrl Pts',(-0.7911,-6.22557561058557E-13,-8.67313315082367));
#60131=CARTESIAN_POINT('Ctrl Pts',(-0.791099999999827,-0.220167589667295,
-8.6642744072504));
#60132=CARTESIAN_POINT('Ctrl Pts',(-0.69421457667203,-0.438610418339221,
-8.65541566367713));
#60133=CARTESIAN_POINT('Ctrl Pts',(-0.531017389079877,-0.586395551223566,
-8.64655692010385));
#60134=CARTESIAN_POINT('Ctrl Pts',(-0.367820201487724,-0.734180684107912,
-8.63769817653058));
#60135=CARTESIAN_POINT('Ctrl Pts',(-0.14086817587113,-0.808992666571442,
-8.62883943295731));
#60136=CARTESIAN_POINT('Ctrl Pts',(0.0782205473253575,-0.787223447298238,
-8.61998068938404));
#60137=CARTESIAN_POINT('Ctrl Pts',(0.297309270521845,-0.765454228025034,
-8.61112194581076));
#60138=CARTESIAN_POINT('Ctrl Pts',(0.505102072676081,-0.647444880833851,
-8.60226320223749));
#60139=CARTESIAN_POINT('Ctrl Pts',(0.636026795762083,-0.470435038100499,
-8.59340445866422));
#60140=CARTESIAN_POINT('Ctrl Pts',(0.766951518848085,-0.293425195367147,
-8.58454571509095));
#60141=CARTESIAN_POINT('Ctrl Pts',(0.818956872247114,-0.0601881960093249,
-8.57568697151767));
#60142=CARTESIAN_POINT('Ctrl Pts',(0.775631781004096,0.155674501111823,
-8.5668282279444));
#60143=CARTESIAN_POINT('Ctrl Pts',(0.732306689761077,0.37153719823297,-8.55796948437113));
#60144=CARTESIAN_POINT('Ctrl Pts',(0.594329958849801,0.566643518936929,
-8.54911074079786));
#60145=CARTESIAN_POINT('Ctrl Pts',(0.40524223024355,0.679424716085038,-8.54025199722458));
#60146=CARTESIAN_POINT('Ctrl Pts',(0.216154501637298,0.792205913233147,
-8.53139325365131));
#60147=CARTESIAN_POINT('Ctrl Pts',(-0.0210816529306007,0.820894963712987,
-8.52253451007804));
#60148=CARTESIAN_POINT('Ctrl Pts',(-0.231602780753753,0.756438604215259,
-8.51367576650477));
#60149=CARTESIAN_POINT('Ctrl Pts',(-0.442123908576904,0.691982244717531,
-8.5048170229315));
#60150=CARTESIAN_POINT('Ctrl Pts',(-0.622631625634545,0.535390358803103,
-8.49595827935822));
#60151=CARTESIAN_POINT('Ctrl Pts',(-0.716163994722386,0.336077881841805,
-8.48709953578495));
#60152=CARTESIAN_POINT('Ctrl Pts',(-0.765317280859654,0.231334857513987,
-8.48244407413119));
#60153=CARTESIAN_POINT('Ctrl Pts',(-0.791100000000089,0.11570283783594,
-8.47778861247743));
#60154=CARTESIAN_POINT('Ctrl Pts',(-0.7911,-6.0551563763056E-13,-8.47313315082367));
#60155=CARTESIAN_POINT('Origin',(0.,0.,-5.925));
#60156=CARTESIAN_POINT('',(-0.7911,-6.65578703262781E-14,-8.24466684917629));
#60157=CARTESIAN_POINT('',(-0.789508070680606,0.000139428570836753,-8.27313315082367));
#60158=CARTESIAN_POINT('',(-0.7911,-9.68818082805471E-17,-5.925));
#60159=CARTESIAN_POINT('Ctrl Pts',(-0.7911,-4.40758540776187E-14,-8.24466684917629));
#60160=CARTESIAN_POINT('Ctrl Pts',(-0.791100000000012,0.220167589666636,
-8.25352559274957));
#60161=CARTESIAN_POINT('Ctrl Pts',(-0.694214576672393,0.43861041833865,
-8.26238433632284));
#60162=CARTESIAN_POINT('Ctrl Pts',(-0.531017389080355,0.586395551223134,
-8.27124307989611));
#60163=CARTESIAN_POINT('Ctrl Pts',(-0.367820201488317,0.734180684107618,
-8.28010182346939));
#60164=CARTESIAN_POINT('Ctrl Pts',(-0.140868175871773,0.808992666571332,
-8.28896056704266));
#60165=CARTESIAN_POINT('Ctrl Pts',(0.0782205473247389,0.787223447298299,
-8.29781931061593));
#60166=CARTESIAN_POINT('Ctrl Pts',(0.297309270521251,0.765454228025267,
-8.3066780541892));
#60167=CARTESIAN_POINT('Ctrl Pts',(0.505102072675586,0.647444880834239,
-8.31553679776248));
#60168=CARTESIAN_POINT('Ctrl Pts',(0.636026795761727,0.47043503810098,-8.32439554133575));
#60169=CARTESIAN_POINT('Ctrl Pts',(0.766951518847867,0.293425195367722,
-8.33325428490902));
#60170=CARTESIAN_POINT('Ctrl Pts',(0.818956872247071,0.0601881960099293,
-8.34211302848229));
#60171=CARTESIAN_POINT('Ctrl Pts',(0.775631781004209,-0.155674501111257,
-8.35097177205557));
#60172=CARTESIAN_POINT('Ctrl Pts',(0.732306689761347,-0.371537198232444,
-8.35983051562884));
#60173=CARTESIAN_POINT('Ctrl Pts',(0.594329958850205,-0.566643518936508,
-8.36868925920211));
#60174=CARTESIAN_POINT('Ctrl Pts',(0.405242230244025,-0.679424716084754,
-8.37754800277538));
#60175=CARTESIAN_POINT('Ctrl Pts',(0.216154501637846,-0.792205913232999,
-8.38640674634866));
#60176=CARTESIAN_POINT('Ctrl Pts',(-0.0210816529300418,-0.820894963713003,
-8.39526548992193));
#60177=CARTESIAN_POINT('Ctrl Pts',(-0.231602780753244,-0.756438604215415,
-8.4041242334952));
#60178=CARTESIAN_POINT('Ctrl Pts',(-0.442123908576446,-0.691982244717826,
-8.41298297706848));
#60179=CARTESIAN_POINT('Ctrl Pts',(-0.622631625634197,-0.535390358803511,
-8.42184172064175));
#60180=CARTESIAN_POINT('Ctrl Pts',(-0.71616399472217,-0.336077881842266,
-8.43070046421502));
#60181=CARTESIAN_POINT('Ctrl Pts',(-0.765317280859482,-0.231334857514527,
-8.43535592586878));
#60182=CARTESIAN_POINT('Ctrl Pts',(-0.791099999999991,-0.115702837836555,
-8.44001138752254));
#60183=CARTESIAN_POINT('Ctrl Pts',(-0.7911,-6.11177775056149E-14,-8.44466684917629));
#60184=CARTESIAN_POINT('Ctrl Pts',(-0.792046526175884,0.000895756401040832,
-8.47313315082367));
#60185=CARTESIAN_POINT('Ctrl Pts',(-0.79009966938662,-0.226486983166913,
-8.46396260995651));
#60186=CARTESIAN_POINT('Ctrl Pts',(-0.686581284676827,-0.455897606404604,
-8.45479206908934));
#60187=CARTESIAN_POINT('Ctrl Pts',(-0.514165232817067,-0.60306395904845,
-8.44562152822217));
#60188=CARTESIAN_POINT('Ctrl Pts',(-0.315041783825346,-0.773026508346413,
-8.43503046255924));
#60189=CARTESIAN_POINT('Ctrl Pts',(-0.0240228999910702,-0.833291976129561,
-8.42443939689631));
#60190=CARTESIAN_POINT('Ctrl Pts',(0.227752151920718,-0.758514331340251,
-8.41384833123338));
#60191=CARTESIAN_POINT('Ctrl Pts',(0.35363967787661,-0.721125508945596,
-8.40855279840192));
#60192=CARTESIAN_POINT('Ctrl Pts',(0.46971624585188,-0.649975908407827,
-8.40325726557046));
#60193=CARTESIAN_POINT('Ctrl Pts',(0.562287117707967,-0.55603470216158,
-8.397961732739));
#60194=CARTESIAN_POINT('Ctrl Pts',(0.654857989564054,-0.462093495915333,
-8.39266619990753));
#60195=CARTESIAN_POINT('Ctrl Pts',(0.723923165300961,-0.345360683960607,
-8.38737066707606));
#60196=CARTESIAN_POINT('Ctrl Pts',(0.760326468312458,-0.219339720876201,
-8.38207513424459));
#60197=CARTESIAN_POINT('Ctrl Pts',(0.796729771323954,-0.0933187577917998,
-8.37677960141313));
#60198=CARTESIAN_POINT('Ctrl Pts',(0.800471201610043,0.041990356422283,
-8.37148406858167));
#60199=CARTESIAN_POINT('Ctrl Pts',(0.772117869221663,0.170847148582369,
-8.3661885357502));
#60200=CARTESIAN_POINT('Ctrl Pts',(0.743764536833282,0.299703940742463,
-8.36089300291874));
#60201=CARTESIAN_POINT('Ctrl Pts',(0.683316441770433,0.422108410848553,
-8.35559747008728));
#60202=CARTESIAN_POINT('Ctrl Pts',(0.596716058659417,0.520851492288747,
-8.35030193725581));
#60203=CARTESIAN_POINT('Ctrl Pts',(0.423515292437392,0.718337655169128,
-8.33971087159288));
#60204=CARTESIAN_POINT('Ctrl Pts',(0.145705374022713,0.821178263385903,
-8.32911980592995));
#60205=CARTESIAN_POINT('Ctrl Pts',(-0.113892328640817,0.783836609160277,
-8.31852874026702));
#60206=CARTESIAN_POINT('Ctrl Pts',(-0.243691179972587,0.765165782047463,
-8.31323320743556));
#60207=CARTESIAN_POINT('Ctrl Pts',(-0.368936977366574,0.711449389324045,
-8.3079376746041));
#60208=CARTESIAN_POINT('Ctrl Pts',(-0.474613758660987,0.632207743903391,
-8.30264214177263));
#60209=CARTESIAN_POINT('Ctrl Pts',(-0.580290539955397,0.55296609848274,
-8.29734660894117));
#60210=CARTESIAN_POINT('Ctrl Pts',(-0.666398305150239,0.448199200364853,
-8.2920510761097));
#60211=CARTESIAN_POINT('Ctrl Pts',(-0.72048428825659,0.328818528118176,
-8.28675554327824));
#60212=CARTESIAN_POINT('Ctrl Pts',(-0.766861773558151,0.226452350147002,
-8.28221474579338));
#60213=CARTESIAN_POINT('Ctrl Pts',(-0.789694706689629,0.113341149727473,
-8.27767394830853));
#60214=CARTESIAN_POINT('Ctrl Pts',(-0.789508070680606,0.000139428570836753,
-8.27313315082367));
#60215=CARTESIAN_POINT('Origin',(0.,0.,-5.925));
#60216=CARTESIAN_POINT('',(-0.790047180336124,-0.000229621036622829,-8.04466684917629));
#60217=CARTESIAN_POINT('',(-0.791166926155794,-0.000598937135766913,-8.07313315082367));
#60218=CARTESIAN_POINT('',(-0.7911,-9.68818082805471E-17,-5.925));
#60219=CARTESIAN_POINT('Ctrl Pts',(-0.790047180336124,-0.000229621036622829,
-8.04466684917629));
#60220=CARTESIAN_POINT('Ctrl Pts',(-0.788717572232258,0.183736650574578,
-8.05205977984234));
#60221=CARTESIAN_POINT('Ctrl Pts',(-0.725318385967807,0.368133308188168,
-8.05945271050839));
#60222=CARTESIAN_POINT('Ctrl Pts',(-0.608036083416137,0.508275660055627,
-8.06684564117444));
#60223=CARTESIAN_POINT('Ctrl Pts',(-0.440018199367973,0.70904270601237,
-8.07743670683737));
#60224=CARTESIAN_POINT('Ctrl Pts',(-0.161414669232722,0.818985550804046,
-8.0880277725003));
#60225=CARTESIAN_POINT('Ctrl Pts',(0.0984571409497746,0.786513157848435,
-8.09861883816323));
#60226=CARTESIAN_POINT('Ctrl Pts',(0.358328951132271,0.754040764892825,
-8.10920990382615));
#60227=CARTESIAN_POINT('Ctrl Pts',(0.599469041362017,0.579153134189927,
-8.11980096948908));
#60228=CARTESIAN_POINT('Ctrl Pts',(0.713725172026125,0.343242789982087,
-8.13039203515201));
#60229=CARTESIAN_POINT('Ctrl Pts',(0.770853237358178,0.225287617878169,
-8.13568756798348));
#60230=CARTESIAN_POINT('Ctrl Pts',(0.796260312798822,0.0920767673980271,
-8.14098310081494));
#60231=CARTESIAN_POINT('Ctrl Pts',(0.7895301003907,-0.0398380714741007,
-8.14627863364641));
#60232=CARTESIAN_POINT('Ctrl Pts',(0.782799887982578,-0.17175291034624,
-8.15157416647787));
#60233=CARTESIAN_POINT('Ctrl Pts',(0.74393238772568,-0.302371737610357,
-8.15686969930934));
#60234=CARTESIAN_POINT('Ctrl Pts',(0.675220556067583,-0.414063392546229,
-8.1621652321408));
#60235=CARTESIAN_POINT('Ctrl Pts',(0.537796892751397,-0.637446702417962,
-8.17275629780373));
#60236=CARTESIAN_POINT('Ctrl Pts',(0.28099590383042,-0.785121322976735,
-8.18334736346666));
#60237=CARTESIAN_POINT('Ctrl Pts',(0.0184047961489411,-0.791844426109169,
-8.19393842912959));
#60238=CARTESIAN_POINT('Ctrl Pts',(-0.112890757691798,-0.795205977675386,
-8.19923396196105));
#60239=CARTESIAN_POINT('Ctrl Pts',(-0.245633841222665,-0.763329649885019,
-8.20452949479251));
#60240=CARTESIAN_POINT('Ctrl Pts',(-0.362797491579033,-0.70266117884375,
-8.20982502762398));
#60241=CARTESIAN_POINT('Ctrl Pts',(-0.479961141935401,-0.641992707802481,
-8.21512056045545));
#60242=CARTESIAN_POINT('Ctrl Pts',(-0.581545359117274,-0.55253209351031,
-8.22041609328692));
#60243=CARTESIAN_POINT('Ctrl Pts',(-0.655091465745599,-0.443916009035298,
-8.22571162611838));
#60244=CARTESIAN_POINT('Ctrl Pts',(-0.728637572373925,-0.335299924560287,
-8.23100715894985));
#60245=CARTESIAN_POINT('Ctrl Pts',(-0.774145568448705,-0.207528369902432,
-8.2363026917813));
#60246=CARTESIAN_POINT('Ctrl Pts',(-0.787097833118284,-0.076278396999101,
-8.24159822461277));
#60247=CARTESIAN_POINT('Ctrl Pts',(-0.789599667449425,-0.0509264067064596,
-8.24262109946728));
#60248=CARTESIAN_POINT('Ctrl Pts',(-0.790886846250653,-0.025444636501807,
-8.24364397432178));
#60249=CARTESIAN_POINT('Ctrl Pts',(-0.790961777408698,4.04858511152684E-5,
-8.24466684917629));
#60250=CARTESIAN_POINT('Ctrl Pts',(-0.789508070680606,0.000139428570836753,
-8.27313315082367));
#60251=CARTESIAN_POINT('Ctrl Pts',(-0.78925939235702,-0.150693277248314,
-8.2670828826456));
#60252=CARTESIAN_POINT('Ctrl Pts',(-0.748142827911767,-0.301686689427919,
-8.26103261446752));
#60253=CARTESIAN_POINT('Ctrl Pts',(-0.667400237636104,-0.427637321659363,
-8.25498234628945));
#60254=CARTESIAN_POINT('Ctrl Pts',(-0.52605938294417,-0.648115385935031,
-8.24439128062652));
#60255=CARTESIAN_POINT('Ctrl Pts',(-0.263292835701562,-0.791855073477848,
-8.23380021496359));
#60256=CARTESIAN_POINT('Ctrl Pts',(-0.00149710346494951,-0.79249592050826,
-8.22320914930066));
#60257=CARTESIAN_POINT('Ctrl Pts',(0.260298628771663,-0.793136767538672,
-8.21261808363773));
#60258=CARTESIAN_POINT('Ctrl Pts',(0.521123546002274,-0.65067877405668,
-8.2020270179748));
#60259=CARTESIAN_POINT('Ctrl Pts',(0.664616688819202,-0.430696750041217,
-8.19143595231187));
#60260=CARTESIAN_POINT('Ctrl Pts',(0.736363260227663,-0.320705738033488,
-8.18614041948041));
#60261=CARTESIAN_POINT('Ctrl Pts',(0.778776888032708,-0.191333718392383,
-8.18084488664894));
#60262=CARTESIAN_POINT('Ctrl Pts',(0.788520488945965,-0.0598066155259459,
-8.17554935381748));
#60263=CARTESIAN_POINT('Ctrl Pts',(0.798264089859222,0.071720487340495,
-8.17025382098602));
#60264=CARTESIAN_POINT('Ctrl Pts',(0.775337663880695,0.205402673432278,
-8.16495828815455));
#60265=CARTESIAN_POINT('Ctrl Pts',(0.721503951327807,0.325020460569648,
-8.15966275532308));
#60266=CARTESIAN_POINT('Ctrl Pts',(0.667670238774919,0.444638247707018,
-8.15436722249162));
#60267=CARTESIAN_POINT('Ctrl Pts',(0.582929239647671,0.550191635889973,
-8.14907168966016));
#60268=CARTESIAN_POINT('Ctrl Pts',(0.477902833472298,0.630050501078506,
-8.14377615682869));
#60269=CARTESIAN_POINT('Ctrl Pts',(0.372876427296924,0.709909366267039,
-8.13848062399723));
#60270=CARTESIAN_POINT('Ctrl Pts',(0.247564614073427,0.764073708461148,
-8.13318509116576));
#60271=CARTESIAN_POINT('Ctrl Pts',(0.117637024355971,0.783273810478888,
-8.1278895583343));
#60272=CARTESIAN_POINT('Ctrl Pts',(-0.14221815507894,0.821674014514368,
-8.11729849267136));
#60273=CARTESIAN_POINT('Ctrl Pts',(-0.420536440489676,0.72021725784437,
-8.10670742700844));
#60274=CARTESIAN_POINT('Ctrl Pts',(-0.59422621506534,0.523704590119495,
-8.09611636134551));
#60275=CARTESIAN_POINT('Ctrl Pts',(-0.681071102353172,0.425448256257057,
-8.09082082851405));
#60276=CARTESIAN_POINT('Ctrl Pts',(-0.741758861932236,0.303427944630902,
-8.08552529568258));
#60277=CARTESIAN_POINT('Ctrl Pts',(-0.771007462975747,0.174620569800434,
-8.08022976285112));
#60278=CARTESIAN_POINT('Ctrl Pts',(-0.784072939139481,0.117081760232854,
-8.07786422550864));
#60279=CARTESIAN_POINT('Ctrl Pts',(-0.790864896553931,0.0581886278955768,
-8.07549868816616));
#60280=CARTESIAN_POINT('Ctrl Pts',(-0.791166926155794,-0.000598937135766913,
-8.07313315082367));
#60281=CARTESIAN_POINT('Origin',(0.,0.,-5.925));
#60282=CARTESIAN_POINT('',(-0.792491847548892,-0.000436464152781535,-7.8446668491763));
#60283=CARTESIAN_POINT('',(-0.792077464554372,0.000352317614289522,-7.87313315082367));
#60284=CARTESIAN_POINT('',(-0.7911,-9.68818082805471E-17,-5.925));
#60285=CARTESIAN_POINT('Ctrl Pts',(-0.792491847548892,-0.000436464152781535,
-7.8446668491763));
#60286=CARTESIAN_POINT('Ctrl Pts',(-0.792298347834538,0.25945640178687,
-7.85518005253144));
#60287=CARTESIAN_POINT('Ctrl Pts',(-0.651590353855427,0.520785898705083,
-7.86569325588657));
#60288=CARTESIAN_POINT('Ctrl Pts',(-0.434108069765603,0.663209574596977,
-7.87620645924171));
#60289=CARTESIAN_POINT('Ctrl Pts',(-0.21501508035881,0.806688060874836,
-7.88679752490464));
#60290=CARTESIAN_POINT('Ctrl Pts',(0.0819936133437958,0.829492936536737,
-7.89738859056758));
#60291=CARTESIAN_POINT('Ctrl Pts',(0.321795719765056,0.723648221720539,
-7.9079796562305));
#60292=CARTESIAN_POINT('Ctrl Pts',(0.441696772975692,0.670725864312437,
-7.91327518906196));
#60293=CARTESIAN_POINT('Ctrl Pts',(0.547296179365993,0.585641109284806,
-7.91857072189342));
#60294=CARTESIAN_POINT('Ctrl Pts',(0.627561863841052,0.480740011247315,
-7.92386625472489));
#60295=CARTESIAN_POINT('Ctrl Pts',(0.707827548316103,0.375838913209837,
-7.92916178755636));
#60296=CARTESIAN_POINT('Ctrl Pts',(0.762759510875919,0.251121472162503,
-7.93445732038783));
#60297=CARTESIAN_POINT('Ctrl Pts',(0.782691847255788,0.121510347799813,
-7.9397528532193));
#60298=CARTESIAN_POINT('Ctrl Pts',(0.822556520015527,-0.137711900925585,
-7.95034391888223));
#60299=CARTESIAN_POINT('Ctrl Pts',(0.72242268805546,-0.416508882912403,
-7.96093498454514));
#60300=CARTESIAN_POINT('Ctrl Pts',(0.526630374428653,-0.591622160175378,
-7.97152605020807));
#60301=CARTESIAN_POINT('Ctrl Pts',(0.428734217615251,-0.679178798806863,
-7.97682158303954));
#60302=CARTESIAN_POINT('Ctrl Pts',(0.306923440385164,-0.740814511257387,
-7.98211711587101));
#60303=CARTESIAN_POINT('Ctrl Pts',(0.178348500349687,-0.770419732725704,
-7.98741264870248));
#60304=CARTESIAN_POINT('Ctrl Pts',(0.0497735603142099,-0.800024954194021,
-7.99270818153394));
#60305=CARTESIAN_POINT('Ctrl Pts',(-0.0855655425266594,-0.797599684680131,
-7.9980037143654));
#60306=CARTESIAN_POINT('Ctrl Pts',(-0.211934595031162,-0.762423752908789,
-8.00329924719686));
#60307=CARTESIAN_POINT('Ctrl Pts',(-0.338303647535658,-0.727247821137449,
-8.00859478002833));
#60308=CARTESIAN_POINT('Ctrl Pts',(-0.455702649703791,-0.659321227108661,
-8.01389031285979));
#60309=CARTESIAN_POINT('Ctrl Pts',(-0.550539734854605,-0.567668383032269,
-8.01918584569126));
#60310=CARTESIAN_POINT('Ctrl Pts',(-0.64537682000543,-0.476015538955867,
-8.02448137852272));
#60311=CARTESIAN_POINT('Ctrl Pts',(-0.717651988138931,-0.360636444831854,
-8.02977691135419));
#60312=CARTESIAN_POINT('Ctrl Pts',(-0.756263393901083,-0.235118507562208,
-8.03507244418565));
#60313=CARTESIAN_POINT('Ctrl Pts',(-0.779582008283564,-0.159314368357715,
-8.03827057918253));
#60314=CARTESIAN_POINT('Ctrl Pts',(-0.790622360383279,-0.0798122653305001,
-8.04146871417941));
#60315=CARTESIAN_POINT('Ctrl Pts',(-0.790047180336124,-0.000229621036622829,
-8.04466684917629));
#60316=CARTESIAN_POINT('Ctrl Pts',(-0.791166926155794,-0.000598937135766913,
-8.07313315082367));
#60317=CARTESIAN_POINT('Ctrl Pts',(-0.791541025247406,-0.0734142325262931,
-8.07020315533469));
#60318=CARTESIAN_POINT('Ctrl Pts',(-0.781958453425139,-0.146067569424397,
-8.0672731598457));
#60319=CARTESIAN_POINT('Ctrl Pts',(-0.762007978713805,-0.215784787311132,
-8.06434316435672));
#60320=CARTESIAN_POINT('Ctrl Pts',(-0.689892923086983,-0.467791875803772,
-8.05375209869379));
#60321=CARTESIAN_POINT('Ctrl Pts',(-0.482309986174684,-0.681435389142571,
-8.04316103303086));
#60322=CARTESIAN_POINT('Ctrl Pts',(-0.231854275641584,-0.757984400195306,
-8.03256996736793));
#60323=CARTESIAN_POINT('Ctrl Pts',(0.0186014348915136,-0.834533411248041,
-8.021978901705));
#60324=CARTESIAN_POINT('Ctrl Pts',(0.311929919045417,-0.77398792001471,
-8.01138783604208));
#60325=CARTESIAN_POINT('Ctrl Pts',(0.511883075792864,-0.605002266159273,
-8.00079677037915));
#60326=CARTESIAN_POINT('Ctrl Pts',(0.711836232540309,-0.43601661230384,
-7.99020570471622));
#60327=CARTESIAN_POINT('Ctrl Pts',(0.818414061881308,-0.158590795826307,
-7.97961463905329));
#60328=CARTESIAN_POINT('Ctrl Pts',(0.78537732129719,0.101968116316403,-7.96902357339036));
#60329=CARTESIAN_POINT('Ctrl Pts',(0.76885895100513,0.232247572387769,-7.9637280405589));
#60330=CARTESIAN_POINT('Ctrl Pts',(0.717436938231784,0.358310302375426,
-7.95843250772743));
#60331=CARTESIAN_POINT('Ctrl Pts',(0.63971903264416,0.464866595940244,-7.95313697489597));
#60332=CARTESIAN_POINT('Ctrl Pts',(0.562001127056541,0.571422889505055,
-7.9478414420645));
#60333=CARTESIAN_POINT('Ctrl Pts',(0.45798732865465,0.658472746647027,-7.94254590923304));
#60334=CARTESIAN_POINT('Ctrl Pts',(0.3395209030078,0.714794941218329,-7.93725037640157));
#60335=CARTESIAN_POINT('Ctrl Pts',(0.221054477360954,0.771117135789629,
-7.93195484357011));
#60336=CARTESIAN_POINT('Ctrl Pts',(0.0881354244691417,0.796711667790262,
-7.92665931073864));
#60337=CARTESIAN_POINT('Ctrl Pts',(-0.0436115676640736,0.789590262931357,
-7.92136377790718));
#60338=CARTESIAN_POINT('Ctrl Pts',(-0.175358559797293,0.782468858072452,
-7.91606824507571));
#60339=CARTESIAN_POINT('Ctrl Pts',(-0.305933491171922,0.74263151635401,
-7.91077271224425));
#60340=CARTESIAN_POINT('Ctrl Pts',(-0.417392339406398,0.673156717775511,
-7.90547717941278));
#60341=CARTESIAN_POINT('Ctrl Pts',(-0.640310035875351,0.534207120618512,
-7.89488611374986));
#60342=CARTESIAN_POINT('Ctrl Pts',(-0.786763399783684,0.27670769602129,
-7.88429504808694));
#60343=CARTESIAN_POINT('Ctrl Pts',(-0.791935199270052,0.0144890489754226,
-7.873703982424));
#60344=CARTESIAN_POINT('Ctrl Pts',(-0.792028114898857,0.00977807544695631,
-7.87351370522389));
#60345=CARTESIAN_POINT('Ctrl Pts',(-0.792075428969904,0.00506557869147931,
-7.87332342802378));
#60346=CARTESIAN_POINT('Ctrl Pts',(-0.792077464554372,0.000352317614289522,
-7.87313315082367));
#60347=CARTESIAN_POINT('Origin',(0.,0.,-5.925));
#60348=CARTESIAN_POINT('',(-0.790740166226785,0.000940778128334207,-7.64466684917629));
#60349=CARTESIAN_POINT('',(-0.790714182338634,7.12898943596447E-5,-7.67313315082367));
#60350=CARTESIAN_POINT('',(-0.7911,-9.68818082805471E-17,-5.925));
#60351=CARTESIAN_POINT('Ctrl Pts',(-0.790740166226785,0.000940778128334207,
-7.64466684917629));
#60352=CARTESIAN_POINT('Ctrl Pts',(-0.791434367191261,0.0767299662908557,
-7.6477092595576));
#60353=CARTESIAN_POINT('Ctrl Pts',(-0.781492355410326,0.152314472677872,
-7.6507516699389));
#60354=CARTESIAN_POINT('Ctrl Pts',(-0.760203509104705,0.224471336293998,
-7.6537940803202));
#60355=CARTESIAN_POINT('Ctrl Pts',(-0.686093990383465,0.475659698418317,
-7.66438514598313));
#60356=CARTESIAN_POINT('Ctrl Pts',(-0.474479483182523,0.685310662716084,
-7.67497621164606));
#60357=CARTESIAN_POINT('Ctrl Pts',(-0.223185687336729,0.759873267740378,
-7.68556727730899));
#60358=CARTESIAN_POINT('Ctrl Pts',(-0.0975387894138313,0.797154570252525,
-7.69086281014045));
#60359=CARTESIAN_POINT('Ctrl Pts',(0.0380279306702764,0.800663782946304,
-7.69615834297192));
#60360=CARTESIAN_POINT('Ctrl Pts',(0.167113678227793,0.772669314720665,
-7.70145387580338));
#60361=CARTESIAN_POINT('Ctrl Pts',(0.29619942578531,0.744674846495026,-7.70674940863485));
#60362=CARTESIAN_POINT('Ctrl Pts',(0.418804200816231,0.685176697349972,
-7.71204494146632));
#60363=CARTESIAN_POINT('Ctrl Pts',(0.517900519948477,0.599291534914524,
-7.71734047429778));
#60364=CARTESIAN_POINT('Ctrl Pts',(0.716093158212969,0.427521210043628,
-7.72793153996071));
#60365=CARTESIAN_POINT('Ctrl Pts',(0.820251972882747,0.150202832011168,
-7.73852260562363));
#60366=CARTESIAN_POINT('Ctrl Pts',(0.784380873848862,-0.110013528356924,
-7.74911367128656));
#60367=CARTESIAN_POINT('Ctrl Pts',(0.766445324331919,-0.24012170854097,
-7.75440920411803));
#60368=CARTESIAN_POINT('Ctrl Pts',(0.713502296389051,-0.365954384308944,
-7.7597047369495));
#60369=CARTESIAN_POINT('Ctrl Pts',(0.634668669730602,-0.471752511188351,
-7.76500026978096));
#60370=CARTESIAN_POINT('Ctrl Pts',(0.555835043072157,-0.577550638067753,
-7.77029580261242));
#60371=CARTESIAN_POINT('Ctrl Pts',(0.451110817698131,-0.663314216058609,
-7.77559133544388));
#60372=CARTESIAN_POINT('Ctrl Pts',(0.332022261747654,-0.718308756228488,
-7.78088686827535));
#60373=CARTESIAN_POINT('Ctrl Pts',(0.21293370579717,-0.77330329639837,-7.78618240110681));
#60374=CARTESIAN_POINT('Ctrl Pts',(0.0794808192702385,-0.797528798747268,
-7.79147793393828));
#60375=CARTESIAN_POINT('Ctrl Pts',(-0.0521348267623253,-0.789064859556369,
-7.79677346676974));
#60376=CARTESIAN_POINT('Ctrl Pts',(-0.183750472794889,-0.78060092036547,
-7.80206899960121));
#60377=CARTESIAN_POINT('Ctrl Pts',(-0.31352887833308,-0.739447539634773,
-7.80736453243267));
#60378=CARTESIAN_POINT('Ctrl Pts',(-0.424212478024202,-0.668774107633984,
-7.81266006526414));
#60379=CARTESIAN_POINT('Ctrl Pts',(-0.645579677406446,-0.527427243632406,
-7.82325113092707));
#60380=CARTESIAN_POINT('Ctrl Pts',(-0.790567653400404,-0.268000174550464,
-7.83384219659));
#60381=CARTESIAN_POINT('Ctrl Pts',(-0.792472998841892,-0.00621059156258216,
-7.84443326225293));
#60382=CARTESIAN_POINT('Ctrl Pts',(-0.792487006364641,-0.00428599381809321,
-7.84451112456072));
#60383=CARTESIAN_POINT('Ctrl Pts',(-0.792493280635821,-0.00236126838574793,
-7.84458898686851));
#60384=CARTESIAN_POINT('Ctrl Pts',(-0.792491847548892,-0.000436464152781535,
-7.8446668491763));
#60385=CARTESIAN_POINT('Ctrl Pts',(-0.792077464554372,0.000352317614289522,
-7.87313315082367));
#60386=CARTESIAN_POINT('Ctrl Pts',(-0.792132080551777,-0.126107408735287,
-7.86802789519232));
#60387=CARTESIAN_POINT('Ctrl Pts',(-0.759591516535767,-0.253117356739719,
-7.86292263956095));
#60388=CARTESIAN_POINT('Ctrl Pts',(-0.70069585656924,-0.366019354609049,
-7.8578173839296));
#60389=CARTESIAN_POINT('Ctrl Pts',(-0.639605105487552,-0.483129305535492,
-7.85252185109813));
#60390=CARTESIAN_POINT('Ctrl Pts',(-0.550158094686481,-0.585060078253289,
-7.84722631826667));
#60391=CARTESIAN_POINT('Ctrl Pts',(-0.441106678461014,-0.657756894510047,
-7.84193078543521));
#60392=CARTESIAN_POINT('Ctrl Pts',(-0.223003846010083,-0.803150527023559,
-7.83133971977229));
#60393=CARTESIAN_POINT('Ctrl Pts',(0.0735166081384336,-0.831608333692926,
-7.82074865410935));
#60394=CARTESIAN_POINT('Ctrl Pts',(0.313965838386481,-0.727820175866948,
-7.81015758844642));
#60395=CARTESIAN_POINT('Ctrl Pts',(0.554415068634545,-0.624032018040962,
-7.79956652278349));
#60396=CARTESIAN_POINT('Ctrl Pts',(0.738793074982127,-0.387997895719602,
-7.78897545712056));
#60397=CARTESIAN_POINT('Ctrl Pts',(0.781802262290506,-0.129758421763161,
-7.77838439145763));
#60398=CARTESIAN_POINT('Ctrl Pts',(0.824811449598881,0.128481052193258,
-7.76779332579471));
#60399=CARTESIAN_POINT('Ctrl Pts',(0.726451817868084,0.408925877784763,
-7.75720226013178));
#60400=CARTESIAN_POINT('Ctrl Pts',(0.532598074500645,0.58613507367438,-7.74661119446885));
#60401=CARTESIAN_POINT('Ctrl Pts',(0.435671202816917,0.674739671619196,
-7.74131566163738));
#60402=CARTESIAN_POINT('Ctrl Pts',(0.314870803224043,0.737535362138529,
-7.73602012880591));
#60403=CARTESIAN_POINT('Ctrl Pts',(0.186655454501568,0.768440716030238,
-7.73072459597445));
#60404=CARTESIAN_POINT('Ctrl Pts',(0.0584401057790991,0.799346069921944,
-7.72542906314298));
#60405=CARTESIAN_POINT('Ctrl Pts',(-0.0771901920729581,0.798361087186018,
-7.72013353031152));
#60406=CARTESIAN_POINT('Ctrl Pts',(-0.203944522867036,0.764599818966159,
-7.71483799748006));
#60407=CARTESIAN_POINT('Ctrl Pts',(-0.330698853661106,0.730838550746301,
-7.7095424646486));
#60408=CARTESIAN_POINT('Ctrl Pts',(-0.448577217397205,0.664300997042512,
-7.70424693181714));
#60409=CARTESIAN_POINT('Ctrl Pts',(-0.544383506192386,0.573586393088096,
-7.69895139898567));
#60410=CARTESIAN_POINT('Ctrl Pts',(-0.640189794987579,0.482871789133669,
-7.6936558661542));
#60411=CARTESIAN_POINT('Ctrl Pts',(-0.713924008841854,0.367980134928604,
-7.68836033332273));
#60412=CARTESIAN_POINT('Ctrl Pts',(-0.753902240174265,0.242873926022679,
-7.68306480049127));
#60413=CARTESIAN_POINT('Ctrl Pts',(-0.778894990388472,0.164662656408623,
-7.67975425060207));
#60414=CARTESIAN_POINT('Ctrl Pts',(-0.79069510103305,0.0824592962534152,
-7.67644370071287));
#60415=CARTESIAN_POINT('Ctrl Pts',(-0.790044269977258,0.000195073709034593,
-7.67313315082367));
#60416=CARTESIAN_POINT('Origin',(0.,0.,-5.925));
#60417=CARTESIAN_POINT('',(-0.789800442128824,-0.000456880331022314,-7.44466684917629));
#60418=CARTESIAN_POINT('',(-0.7911,-6.10178574333986E-13,-7.47313315082367));
#60419=CARTESIAN_POINT('',(-0.7911,-9.68818082805471E-17,-5.925));
#60420=CARTESIAN_POINT('Ctrl Pts',(-0.789800442128824,-0.000456880331022313,
-7.44466684917629));
#60421=CARTESIAN_POINT('Ctrl Pts',(-0.788892940225841,0.153073306983262,
-7.45082953224669));
#60422=CARTESIAN_POINT('Ctrl Pts',(-0.745378609669688,0.306963099682475,
-7.45699221531708));
#60423=CARTESIAN_POINT('Ctrl Pts',(-0.662015882221351,0.434688630798064,
-7.46315489838748));
#60424=CARTESIAN_POINT('Ctrl Pts',(-0.590383112033339,0.544441920998588,
-7.46845043121894));
#60425=CARTESIAN_POINT('Ctrl Pts',(-0.489327100322849,0.634876055401825,
-7.4737459640504));
#60426=CARTESIAN_POINT('Ctrl Pts',(-0.372816842178655,0.697102900259108,
-7.47904149688187));
#60427=CARTESIAN_POINT('Ctrl Pts',(-0.256306584034461,0.759329745116391,
-7.48433702971333));
#60428=CARTESIAN_POINT('Ctrl Pts',(-0.124342079456564,0.793349300427721,
-7.4896325625448));
#60429=CARTESIAN_POINT('Ctrl Pts',(0.0067861929163434,0.792038660652882,
-7.49492809537627));
#60430=CARTESIAN_POINT('Ctrl Pts',(0.269042737662159,0.789417381103205,
-7.5055191610392));
#60431=CARTESIAN_POINT('Ctrl Pts',(0.527954353588018,0.645475321208852,
-7.51611022670212));
#60432=CARTESIAN_POINT('Ctrl Pts',(0.669065422703021,0.423919558200222,
-7.52670129236505));
#60433=CARTESIAN_POINT('Ctrl Pts',(0.739620957260523,0.313141676695907,
-7.53199682519651));
#60434=CARTESIAN_POINT('Ctrl Pts',(0.78072635511531,0.182960369413022,-7.53729235802798));
#60435=CARTESIAN_POINT('Ctrl Pts',(0.789128762633997,0.0512888694929381,
-7.54258789085944));
#60436=CARTESIAN_POINT('Ctrl Pts',(0.797531170152684,-0.0803826304271457,
-7.54788342369091));
#60437=CARTESIAN_POINT('Ctrl Pts',(0.77323058733527,-0.213544322984428,
-7.55317895652238));
#60438=CARTESIAN_POINT('Ctrl Pts',(0.718063232484806,-0.33255292168919,
-7.55847448935384));
#60439=CARTESIAN_POINT('Ctrl Pts',(0.662895877634341,-0.451561520393951,
-7.5637700221853));
#60440=CARTESIAN_POINT('Ctrl Pts',(0.576861750750826,-0.556417025246192,
-7.56906555501677));
#60441=CARTESIAN_POINT('Ctrl Pts',(0.471066362514449,-0.635167595879746,
-7.57436108784823));
#60442=CARTESIAN_POINT('Ctrl Pts',(0.365270974278072,-0.7139181665133,-7.5796566206797));
#60443=CARTESIAN_POINT('Ctrl Pts',(0.239714324688833,-0.766563802928168,
-7.58495215351116));
#60444=CARTESIAN_POINT('Ctrl Pts',(0.109601684041382,-0.784348458536356,
-7.59024768634263));
#60445=CARTESIAN_POINT('Ctrl Pts',(-0.15062359725352,-0.819917769752734,
-7.60083875200556));
#60446=CARTESIAN_POINT('Ctrl Pts',(-0.42907284278127,-0.716043157742395,
-7.61142981766848));
#60447=CARTESIAN_POINT('Ctrl Pts',(-0.599995200424376,-0.517742971761791,
-7.62202088333141));
#60448=CARTESIAN_POINT('Ctrl Pts',(-0.721818064981508,-0.376406887755678,
-7.62956953861304));
#60449=CARTESIAN_POINT('Ctrl Pts',(-0.789017754349279,-0.187103037074619,
-7.63711819389467));
#60450=CARTESIAN_POINT('Ctrl Pts',(-0.790740166226785,0.000940778128334207,
-7.64466684917629));
#60451=CARTESIAN_POINT('Ctrl Pts',(-0.7911,-6.27220497761982E-13,-7.67313315082367));
#60452=CARTESIAN_POINT('Ctrl Pts',(-0.791099999999826,-0.220167589667307,
-7.6642744072504));
#60453=CARTESIAN_POINT('Ctrl Pts',(-0.694214576672021,-0.438610418339239,
-7.65541566367712));
#60454=CARTESIAN_POINT('Ctrl Pts',(-0.531017389079857,-0.586395551223585,
-7.64655692010385));
#60455=CARTESIAN_POINT('Ctrl Pts',(-0.367820201487694,-0.73418068410793,
-7.63769817653058));
#60456=CARTESIAN_POINT('Ctrl Pts',(-0.140868175871087,-0.808992666571452,
-7.62883943295731));
#60457=CARTESIAN_POINT('Ctrl Pts',(0.0782205473254069,-0.787223447298233,
-7.61998068938403));
#60458=CARTESIAN_POINT('Ctrl Pts',(0.297309270521901,-0.765454228025015,
-7.61112194581076));
#60459=CARTESIAN_POINT('Ctrl Pts',(0.505102072676136,-0.647444880833811,
-7.60226320223749));
#60460=CARTESIAN_POINT('Ctrl Pts',(0.636026795762126,-0.470435038100441,
-7.59340445866422));
#60461=CARTESIAN_POINT('Ctrl Pts',(0.766951518848116,-0.293425195367071,
-7.58454571509094));
#60462=CARTESIAN_POINT('Ctrl Pts',(0.818956872247122,-0.0601881960092344,
-7.57568697151767));
#60463=CARTESIAN_POINT('Ctrl Pts',(0.775631781004077,0.155674501111915,
-7.5668282279444));
#60464=CARTESIAN_POINT('Ctrl Pts',(0.732306689761032,0.371537198233065,
-7.55796948437113));
#60465=CARTESIAN_POINT('Ctrl Pts',(0.594329958849724,0.566643518937013,
-7.54911074079785));
#60466=CARTESIAN_POINT('Ctrl Pts',(0.405242230243449,0.679424716085098,
-7.54025199722458));
#60467=CARTESIAN_POINT('Ctrl Pts',(0.216154501637174,0.792205913233182,
-7.53139325365131));
#60468=CARTESIAN_POINT('Ctrl Pts',(-0.0210816529307384,0.820894963712985,
-7.52253451007803));
#60469=CARTESIAN_POINT('Ctrl Pts',(-0.231602780753886,0.756438604215218,
-7.51367576650476));
#60470=CARTESIAN_POINT('Ctrl Pts',(-0.442123908577034,0.691982244717451,
-7.50481702293149));
#60471=CARTESIAN_POINT('Ctrl Pts',(-0.622631625634652,0.535390358802983,
-7.49595827935822));
#60472=CARTESIAN_POINT('Ctrl Pts',(-0.716163994722455,0.336077881841658,
-7.48709953578494));
#60473=CARTESIAN_POINT('Ctrl Pts',(-0.765317280859679,0.231334857513877,
-7.48244407413119));
#60474=CARTESIAN_POINT('Ctrl Pts',(-0.791100000000089,0.115702837835883,
-7.47778861247743));
#60475=CARTESIAN_POINT('Ctrl Pts',(-0.7911,-6.10178574333986E-13,-7.47313315082367));
#60476=CARTESIAN_POINT('Origin',(0.,0.,-5.925));
#60477=CARTESIAN_POINT('',(-0.791849645310631,-0.000332508792182717,-7.2446668491763));
#60478=CARTESIAN_POINT('',(-0.79118714610156,-0.000297183305454875,-7.27313315082367));
#60479=CARTESIAN_POINT('',(-0.7911,-9.68818082805471E-17,-5.925));
#60480=CARTESIAN_POINT('Ctrl Pts',(-0.791849645310631,-0.000332508792182717,
-7.2446668491763));
#60481=CARTESIAN_POINT('Ctrl Pts',(-0.791466899765427,0.0984544020189313,
-7.24865427210432));
#60482=CARTESIAN_POINT('Ctrl Pts',(-0.771963610279708,0.197476669386961,
-7.25264169503234));
#60483=CARTESIAN_POINT('Ctrl Pts',(-0.735428824803906,0.289981542532058,
-7.25662911796036));
#60484=CARTESIAN_POINT('Ctrl Pts',(-0.686908474825973,0.412833470118636,
-7.26192465079182));
#60485=CARTESIAN_POINT('Ctrl Pts',(-0.608348982910782,0.524190404532698,
-7.26722018362329));
#60486=CARTESIAN_POINT('Ctrl Pts',(-0.507555772110868,0.608077651768299,
-7.27251571645475));
#60487=CARTESIAN_POINT('Ctrl Pts',(-0.305969350511039,0.775852146239502,
-7.28310678211768));
#60488=CARTESIAN_POINT('Ctrl Pts',(-0.0154480533723153,0.833747891996867,
-7.29369784778061));
#60489=CARTESIAN_POINT('Ctrl Pts',(0.235530167590292,0.756228716617091,
-7.30428891344354));
#60490=CARTESIAN_POINT('Ctrl Pts',(0.361019278071595,0.717469128927203,
-7.30958444627501));
#60491=CARTESIAN_POINT('Ctrl Pts',(0.47662261950887,0.64485581095303,-7.31487997910647));
#60492=CARTESIAN_POINT('Ctrl Pts',(0.568264721859209,0.549936321804992,
-7.32017551193793));
#60493=CARTESIAN_POINT('Ctrl Pts',(0.659906824209543,0.455016832656958,
-7.3254710447694));
#60494=CARTESIAN_POINT('Ctrl Pts',(0.727587687472945,0.337791172335062,
-7.33076657760086));
#60495=CARTESIAN_POINT('Ctrl Pts',(0.762580140965066,0.211371190506761,
-7.33606211043232));
#60496=CARTESIAN_POINT('Ctrl Pts',(0.79757259445719,0.0849512086784458,
-7.34135764326379));
#60497=CARTESIAN_POINT('Ctrl Pts',(0.799876638178026,-0.0506630946562756,
-7.34665317609526));
#60498=CARTESIAN_POINT('Ctrl Pts',(0.770219737559319,-0.179172957285143,
-7.35194870892672));
#60499=CARTESIAN_POINT('Ctrl Pts',(0.740562836940614,-0.307682819914002,
-7.35724424175819));
#60500=CARTESIAN_POINT('Ctrl Pts',(0.678944991982372,-0.429088241837008,
-7.36253977458965));
#60501=CARTESIAN_POINT('Ctrl Pts',(0.591287272089202,-0.526872276190706,
-7.36783530742111));
#60502=CARTESIAN_POINT('Ctrl Pts',(0.415971832302867,-0.722440344898095,
-7.37842637308404));
#60503=CARTESIAN_POINT('Ctrl Pts',(0.136496892776829,-0.823522863328255,
-7.38901743874697));
#60504=CARTESIAN_POINT('Ctrl Pts',(-0.122148664389583,-0.783027285047501,
-7.3996085044099));
#60505=CARTESIAN_POINT('Ctrl Pts',(-0.380794221556001,-0.742531706766746,
-7.41019957007283));
#60506=CARTESIAN_POINT('Ctrl Pts',(-0.618610396362793,-0.560458031775068,
-7.42079063573576));
#60507=CARTESIAN_POINT('Ctrl Pts',(-0.724732196623136,-0.321029592484128,
-7.43138170139869));
#60508=CARTESIAN_POINT('Ctrl Pts',(-0.769104306844893,-0.220918728624132,
-7.43581008399122));
#60509=CARTESIAN_POINT('Ctrl Pts',(-0.790452555110128,-0.110780646970491,
-7.44023846658376));
#60510=CARTESIAN_POINT('Ctrl Pts',(-0.789800442128824,-0.000456880331022313,
-7.44466684917629));
#60511=CARTESIAN_POINT('Ctrl Pts',(-0.790956389731621,2.47836052598815E-5,
-7.47313315082367));
#60512=CARTESIAN_POINT('Ctrl Pts',(-0.791255261516135,-0.103754980737926,
-7.46897290773903));
#60513=CARTESIAN_POINT('Ctrl Pts',(-0.771529051809008,-0.20768044077452,
-7.4648126646544));
#60514=CARTESIAN_POINT('Ctrl Pts',(-0.731842388362112,-0.302924165886258,
-7.46065242156976));
#60515=CARTESIAN_POINT('Ctrl Pts',(-0.630808854994587,-0.545393782713588,
-7.45006135590683));
#60516=CARTESIAN_POINT('Ctrl Pts',(-0.400411655188217,-0.731597090389257,
-7.4394702902439));
#60517=CARTESIAN_POINT('Ctrl Pts',(-0.142488267591274,-0.779145933687615,
-7.42887922458097));
#60518=CARTESIAN_POINT('Ctrl Pts',(-0.0135265737928139,-0.802920355336793,
-7.42358369174951));
#60519=CARTESIAN_POINT('Ctrl Pts',(0.122316666953292,-0.79203116089165,
-7.41828815891805));
#60520=CARTESIAN_POINT('Ctrl Pts',(0.247770929032774,-0.750702616278884,
-7.41299262608658));
#60521=CARTESIAN_POINT('Ctrl Pts',(0.373225191112264,-0.709374071666116,
-7.40769709325512));
#60522=CARTESIAN_POINT('Ctrl Pts',(0.488290474525134,-0.63760617688572,
-7.40240156042365));
#60523=CARTESIAN_POINT('Ctrl Pts',(0.577680693555855,-0.541760325560331,
-7.39710602759218));
#60524=CARTESIAN_POINT('Ctrl Pts',(0.756461131617302,-0.350068622909547,
-7.38651496192925));
#60525=CARTESIAN_POINT('Ctrl Pts',(0.832541312150155,-0.0620650940787978,
-7.37592389626633));
#60526=CARTESIAN_POINT('Ctrl Pts',(0.769043337874916,0.192013282204457,
-7.3653328306034));
#60527=CARTESIAN_POINT('Ctrl Pts',(0.705545363599678,0.446091658487705,
-7.35474176494047));
#60528=CARTESIAN_POINT('Ctrl Pts',(0.502469234516344,0.666244882223448,
-7.34415069927754));
#60529=CARTESIAN_POINT('Ctrl Pts',(0.254597269143168,0.750488011820216,
-7.33355963361461));
#60530=CARTESIAN_POINT('Ctrl Pts',(0.0067253037699912,0.834731141416984,
-7.32296856795168));
#60531=CARTESIAN_POINT('Ctrl Pts',(-0.285942497893035,0.783064176874781,
-7.31237750228875));
#60532=CARTESIAN_POINT('Ctrl Pts',(-0.492193727927431,0.620451744893963,
-7.30178643662582));
#60533=CARTESIAN_POINT('Ctrl Pts',(-0.595319342944629,0.539145528903554,
-7.29649090379436));
#60534=CARTESIAN_POINT('Ctrl Pts',(-0.676840815054672,0.43010294605349,
-7.29119537096289));
#60535=CARTESIAN_POINT('Ctrl Pts',(-0.728092771174107,0.308581122741266,
-7.28589983813143));
#60536=CARTESIAN_POINT('Ctrl Pts',(-0.769279542396317,0.210924527476826,
-7.28164427569551));
#60537=CARTESIAN_POINT('Ctrl Pts',(-0.790918414901856,0.105208902504377,
-7.27738871325959));
#60538=CARTESIAN_POINT('Ctrl Pts',(-0.79118714610156,-0.000297183305454875,
-7.27313315082367));
#60539=CARTESIAN_POINT('Origin',(0.,0.,-5.925));
#60540=CARTESIAN_POINT('',(-0.791588575322523,0.000669637297368075,-7.04466684917629));
#60541=CARTESIAN_POINT('',(-0.79166200567261,0.000301740142700173,-7.07313315082367));
#60542=CARTESIAN_POINT('',(-0.7911,-9.68818082805471E-17,-5.925));
#60543=CARTESIAN_POINT('Ctrl Pts',(-0.791588575322523,0.000669637297368075,
-7.04466684917629));
#60544=CARTESIAN_POINT('Ctrl Pts',(-0.791840267553662,0.0457204045308561,
-7.04647901196194));
#60545=CARTESIAN_POINT('Ctrl Pts',(-0.788201041072123,0.0906952463488291,
-7.04829117474759));
#60546=CARTESIAN_POINT('Ctrl Pts',(-0.78049488948999,0.134903742954435,
-7.05010333753324));
#60547=CARTESIAN_POINT('Ctrl Pts',(-0.735456795748511,0.393277380310535,
-7.06069440319616));
#60548=CARTESIAN_POINT('Ctrl Pts',(-0.551503082409662,0.62547465164853,
-7.0712854688591));
#60549=CARTESIAN_POINT('Ctrl Pts',(-0.310027561283053,0.728861607526646,
-7.08187653452203));
#60550=CARTESIAN_POINT('Ctrl Pts',(-0.189289800719745,0.780555085465705,
-7.08717206735349));
#60551=CARTESIAN_POINT('Ctrl Pts',(-0.0541715882094928,0.800045984539794,
-7.09246760018496));
#60552=CARTESIAN_POINT('Ctrl Pts',(0.0771235418761442,0.787023958617911,
-7.09776313301642));
#60553=CARTESIAN_POINT('Ctrl Pts',(0.208418671961781,0.774001932696027,
-7.10305866584788));
#60554=CARTESIAN_POINT('Ctrl Pts',(0.335890719622808,0.728466981778171,
-7.10835419867935));
#60555=CARTESIAN_POINT('Ctrl Pts',(0.44439992785956,0.654763282178348,-7.11364973151082));
#60556=CARTESIAN_POINT('Ctrl Pts',(0.552909136096312,0.581059582578525,
-7.11894526434228));
#60557=CARTESIAN_POINT('Ctrl Pts',(0.642455504908794,0.479187134296732,
-7.12424079717374));
#60558=CARTESIAN_POINT('Ctrl Pts',(0.703042458559388,0.362039630718822,
-7.12953633000521));
#60559=CARTESIAN_POINT('Ctrl Pts',(0.763629412209986,0.244892127140904,
-7.13483186283667));
#60560=CARTESIAN_POINT('Ctrl Pts',(0.795256950698695,0.112469568266862,
-7.14012739566814));
#60561=CARTESIAN_POINT('Ctrl Pts',(0.791745773177158,-0.0188059620644556,
-7.1454229284996));
#60562=CARTESIAN_POINT('Ctrl Pts',(0.784723418134085,-0.281357022727077,
-7.15601399416253));
#60563=CARTESIAN_POINT('Ctrl Pts',(0.637146199050064,-0.539319969218789,
-7.16660505982546));
#60564=CARTESIAN_POINT('Ctrl Pts',(0.413794019970774,-0.67588943946288,
-7.17719612548839));
#60565=CARTESIAN_POINT('Ctrl Pts',(0.190441840891483,-0.81245890970697,
-7.18778719115132));
#60566=CARTESIAN_POINT('Ctrl Pts',(-0.108685298183076,-0.82763490370342,
-7.19837825681425));
#60567=CARTESIAN_POINT('Ctrl Pts',(-0.344564940049599,-0.713842950628033,
-7.20896932247718));
#60568=CARTESIAN_POINT('Ctrl Pts',(-0.580444581916116,-0.600050997552649,
-7.21956038814011));
#60569=CARTESIAN_POINT('Ctrl Pts',(-0.753076726574608,-0.357291097405433,
-7.23015145380304));
#60570=CARTESIAN_POINT('Ctrl Pts',(-0.785979164073213,-0.0972419030109067,
-7.24074251946596));
#60571=CARTESIAN_POINT('Ctrl Pts',(-0.790042967066146,-0.0651230457215302,
-7.24205062936941));
#60572=CARTESIAN_POINT('Ctrl Pts',(-0.791975208424256,-0.0327404421103452,
-7.24335873927285));
#60573=CARTESIAN_POINT('Ctrl Pts',(-0.791849645310631,-0.000332508792182717,
-7.2446668491763));
#60574=CARTESIAN_POINT('Ctrl Pts',(-0.79118714610156,-0.000297183305454875,
-7.27313315082367));
#60575=CARTESIAN_POINT('Ctrl Pts',(-0.791252818382547,-0.026080662562157,
-7.27209318042813));
#60576=CARTESIAN_POINT('Ctrl Pts',(-0.790042241667021,-0.0518516279031952,
-7.27105321003258));
#60577=CARTESIAN_POINT('Ctrl Pts',(-0.787528821063515,-0.0774894029197258,
-7.27001323963704));
#60578=CARTESIAN_POINT('Ctrl Pts',(-0.774730474704658,-0.208037041494106,
-7.26471770680557));
#60579=CARTESIAN_POINT('Ctrl Pts',(-0.728151341858118,-0.335131254868476,
-7.25942217397411));
#60580=CARTESIAN_POINT('Ctrl Pts',(-0.65414120250197,-0.4443580080739,-7.25412664114264));
#60581=CARTESIAN_POINT('Ctrl Pts',(-0.580131063145823,-0.553584761279323,
-7.24883110831117));
#60582=CARTESIAN_POINT('Ctrl Pts',(-0.478689917280069,-0.644944054315796,
-7.24353557547971));
#60583=CARTESIAN_POINT('Ctrl Pts',(-0.361704854671847,-0.704645960598841,
-7.23824004264825));
#60584=CARTESIAN_POINT('Ctrl Pts',(-0.127734729455401,-0.824049773164929,
-7.22764897698532));
#60585=CARTESIAN_POINT('Ctrl Pts',(0.168411062730911,-0.816824038717297,
-7.21705791132239));
#60586=CARTESIAN_POINT('Ctrl Pts',(0.395778758995229,-0.686098000515455,
-7.20646684565946));
#60587=CARTESIAN_POINT('Ctrl Pts',(0.509462607127388,-0.620734981414534,
-7.201171312828));
#60588=CARTESIAN_POINT('Ctrl Pts',(0.605951931279045,-0.524496886375062,
-7.19587577999653));
#60589=CARTESIAN_POINT('Ctrl Pts',(0.674817884216283,-0.411783528693883,
-7.19058024716507));
#60590=CARTESIAN_POINT('Ctrl Pts',(0.743683837153516,-0.299070171012709,
-7.1852847143336));
#60591=CARTESIAN_POINT('Ctrl Pts',(0.784926418876335,-0.169881550689812,
-7.17998918150214));
#60592=CARTESIAN_POINT('Ctrl Pts',(0.7910127788093,-0.0389617481486627,
-7.17469364867067));
#60593=CARTESIAN_POINT('Ctrl Pts',(0.803185498675229,0.222877856933658,
-7.16410258300775));
#60594=CARTESIAN_POINT('Ctrl Pts',(0.674733331381749,0.491642190889068,
-7.15351151734481));
#60595=CARTESIAN_POINT('Ctrl Pts',(0.461857506030851,0.644192828426151,
-7.14292045168188));
#60596=CARTESIAN_POINT('Ctrl Pts',(0.248981680679959,0.796743465963228,
-7.13232938601895));
#60597=CARTESIAN_POINT('Ctrl Pts',(-0.0483178027283369,0.833080407081984,
-7.12173832035603));
#60598=CARTESIAN_POINT('Ctrl Pts',(-0.291778532425519,0.736829229439651,
-7.1111472546931));
#60599=CARTESIAN_POINT('Ctrl Pts',(-0.535239262122695,0.64057805179732,
-7.10055618903017));
#60600=CARTESIAN_POINT('Ctrl Pts',(-0.724861238108755,0.411738755393912,
-7.08996512336723));
#60601=CARTESIAN_POINT('Ctrl Pts',(-0.77679647965955,0.154279819618756,
-7.07937405770431));
#60602=CARTESIAN_POINT('Ctrl Pts',(-0.786997625186592,0.103709609629245,
-7.07729375541076));
#60603=CARTESIAN_POINT('Ctrl Pts',(-0.791886677657495,0.0520352250930769,
-7.07521345311722));
#60604=CARTESIAN_POINT('Ctrl Pts',(-0.79166200567261,0.000301740142700173,
-7.07313315082367));
#60605=CARTESIAN_POINT('Origin',(0.,0.,-5.925));
#60606=CARTESIAN_POINT('',(-0.790368242092622,-4.0643268100924E-5,-6.8446668491763));
#60607=CARTESIAN_POINT('',(-0.790586355510369,0.000136246675610042,-6.87313315082367));
#60608=CARTESIAN_POINT('',(-0.7911,-9.68818082805471E-17,-5.925));
#60609=CARTESIAN_POINT('Ctrl Pts',(-0.789428704647104,-9.28270190198588E-5,
-6.8446668491763));
#60610=CARTESIAN_POINT('Ctrl Pts',(-0.789627609852131,0.122617963089258,
-6.84959928465104));
#60611=CARTESIAN_POINT('Ctrl Pts',(-0.762676444066611,0.245335071236163,
-6.85453172012578));
#60612=CARTESIAN_POINT('Ctrl Pts',(-0.708130487639264,0.354834530672168,
-6.85946415560052));
#60613=CARTESIAN_POINT('Ctrl Pts',(-0.649569173545256,0.472394706662429,
-6.86475968843198));
#60614=CARTESIAN_POINT('Ctrl Pts',(-0.559200793589236,0.574719593190071,
-6.87005522126344));
#60615=CARTESIAN_POINT('Ctrl Pts',(-0.450699011174817,0.64978854520237,
-6.87535075409491));
#60616=CARTESIAN_POINT('Ctrl Pts',(-0.342197228760398,0.724857497214669,
-6.88064628692637));
#60617=CARTESIAN_POINT('Ctrl Pts',(-0.215562043887583,0.772670514711624,
-6.88594181975784));
#60618=CARTESIAN_POINT('Ctrl Pts',(-0.085145053365461,0.78673793060833,
-6.89123735258931));
#60619=CARTESIAN_POINT('Ctrl Pts',(0.0452719371566612,0.800805346505035,
-6.89653288542077));
#60620=CARTESIAN_POINT('Ctrl Pts',(0.179470733328086,0.781127160801492,
-6.90182841825223));
#60621=CARTESIAN_POINT('Ctrl Pts',(0.301485273272662,0.73105952066025,-6.9071239510837));
#60622=CARTESIAN_POINT('Ctrl Pts',(0.423499813217231,0.680991880519011,
-6.91241948391516));
#60623=CARTESIAN_POINT('Ctrl Pts',(0.533330096934947,0.60053478594008,-6.91771501674662));
#60624=CARTESIAN_POINT('Ctrl Pts',(0.61563544230515,0.498204813034557,-6.92301054957809));
#60625=CARTESIAN_POINT('Ctrl Pts',(0.780246133045565,0.293544867223497,
-6.93360161524102));
#60626=CARTESIAN_POINT('Ctrl Pts',(0.834757070395902,0.00139340810604574,
-6.94419268090395));
#60627=CARTESIAN_POINT('Ctrl Pts',(0.752928668151673,-0.247286162201554,
-6.95478374656688));
#60628=CARTESIAN_POINT('Ctrl Pts',(0.671100265907444,-0.495965732509153,
-6.96537481222981));
#60629=CARTESIAN_POINT('Ctrl Pts',(0.45293252406866,-0.701173414006912,
-6.97596587789274));
#60630=CARTESIAN_POINT('Ctrl Pts',(0.199483730741222,-0.76713949008136,
-6.98655694355566));
#60631=CARTESIAN_POINT('Ctrl Pts',(-0.0539650625862154,-0.833105566155808,
-6.99714800921859));
#60632=CARTESIAN_POINT('Ctrl Pts',(-0.342694907402299,-0.759830036806941,
-7.00773907488152));
#60633=CARTESIAN_POINT('Ctrl Pts',(-0.536116319172053,-0.582922401676084,
-7.01833014054445));
#60634=CARTESIAN_POINT('Ctrl Pts',(-0.632827025056924,-0.49446858411066,
-7.02362567337592));
#60635=CARTESIAN_POINT('Ctrl Pts',(-0.705710622680213,-0.380106740099744,
-7.02892120620738));
#60636=CARTESIAN_POINT('Ctrl Pts',(-0.748257350506165,-0.255060363002999,
-7.03421673903885));
#60637=CARTESIAN_POINT('Ctrl Pts',(-0.776244335380633,-0.172805598812202,
-7.03770010908466));
#60638=CARTESIAN_POINT('Ctrl Pts',(-0.791104768246437,-0.0859277116632267,
-7.04118347913048));
#60639=CARTESIAN_POINT('Ctrl Pts',(-0.791588575322523,0.000669637297368075,
-7.04466684917629));
#60640=CARTESIAN_POINT('Ctrl Pts',(-0.79166200567261,0.000301740142700173,
-7.07313315082367));
#60641=CARTESIAN_POINT('Ctrl Pts',(-0.79131476179894,-0.0796554281791444,
-7.06991792028576));
#60642=CARTESIAN_POINT('Ctrl Pts',(-0.778752090620685,-0.159753772823585,
-7.06670268974784));
#60643=CARTESIAN_POINT('Ctrl Pts',(-0.754706361115264,-0.236134921687598,
-7.06348745920992));
#60644=CARTESIAN_POINT('Ctrl Pts',(-0.715102684629,-0.361935817375853,-7.05819192637846));
#60645=CARTESIAN_POINT('Ctrl Pts',(-0.64434939448989,-0.477653231021849,
-7.05289639354698));
#60646=CARTESIAN_POINT('Ctrl Pts',(-0.550084282291531,-0.568870401714096,
-7.04760086071552));
#60647=CARTESIAN_POINT('Ctrl Pts',(-0.455819170093172,-0.660087572406342,
-7.04230532788405));
#60648=CARTESIAN_POINT('Ctrl Pts',(-0.338042235835557,-0.726804500144844,
-7.0370097950526));
#60649=CARTESIAN_POINT('Ctrl Pts',(-0.210924183965184,-0.762145485303659,
-7.03171426222113));
#60650=CARTESIAN_POINT('Ctrl Pts',(-0.0838061320948113,-0.797486470462474,
-7.02641872938967));
#60651=CARTESIAN_POINT('Ctrl Pts',(0.0526530373883043,-0.801451513041607,
-7.0211231965582));
#60652=CARTESIAN_POINT('Ctrl Pts',(0.180466151444074,-0.771225194002639,
-7.01582766372673));
#60653=CARTESIAN_POINT('Ctrl Pts',(0.436092379555614,-0.710772555924703,
-7.0052365980638));
#60654=CARTESIAN_POINT('Ctrl Pts',(0.657134385957696,-0.513554471374351,
-6.99464553240088));
#60655=CARTESIAN_POINT('Ctrl Pts',(0.74580613841404,-0.266729256526248,
-6.98405446673795));
#60656=CARTESIAN_POINT('Ctrl Pts',(0.790142014642215,-0.14331664910219,
-6.97875893390648));
#60657=CARTESIAN_POINT('Ctrl Pts',(0.801385327383953,-0.00750225910368728,
-6.97346340107502));
#60658=CARTESIAN_POINT('Ctrl Pts',(0.780909059079954,0.122987368492008,
-6.96816786824355));
#60659=CARTESIAN_POINT('Ctrl Pts',(0.760432790775956,0.253476996087696,
-6.96287233541209));
#60660=CARTESIAN_POINT('Ctrl Pts',(0.708236941426225,0.378641861280584,
-6.95757680258063));
#60661=CARTESIAN_POINT('Ctrl Pts',(0.62812465768728,0.482367752304858,-6.95228126974916));
#60662=CARTESIAN_POINT('Ctrl Pts',(0.467900090209389,0.689819534353405,
-6.94169020408624));
#60663=CARTESIAN_POINT('Ctrl Pts',(0.196009785174654,0.811515419727503,
-6.9310991384233));
#60664=CARTESIAN_POINT('Ctrl Pts',(-0.0649962387595744,0.789982433361549,
-6.92050807276037));
#60665=CARTESIAN_POINT('Ctrl Pts',(-0.326002262693803,0.768449446995596,
-6.90991700709744));
#60666=CARTESIAN_POINT('Ctrl Pts',(-0.57612400552752,0.603687588889572,
-6.89932594143451));
#60667=CARTESIAN_POINT('Ctrl Pts',(-0.699379104787005,0.372720931969687,
-6.88873487577159));
#60668=CARTESIAN_POINT('Ctrl Pts',(-0.759901568351269,0.259308414662271,
-6.88353430078895));
#60669=CARTESIAN_POINT('Ctrl Pts',(-0.789834639283667,0.129932957625574,
-6.87833372580631));
#60670=CARTESIAN_POINT('Ctrl Pts',(-0.789580398820022,0.000403081535511013,
-6.87313315082368));
#60671=CARTESIAN_POINT('Origin',(0.,0.,-5.925));
#60672=CARTESIAN_POINT('',(-0.7911,2.4980018054066E-14,-6.6446668491763));
#60673=CARTESIAN_POINT('',(-0.7911,-5.4195536947077E-13,-6.67313315082367));
#60674=CARTESIAN_POINT('',(-0.7911,-9.68818082805471E-17,-5.925));
#60675=CARTESIAN_POINT('Ctrl Pts',(-0.7911,2.4980018054066E-15,-6.6446668491763));
#60676=CARTESIAN_POINT('Ctrl Pts',(-0.791099999999999,0.220167589666675,
-6.65352559274957));
#60677=CARTESIAN_POINT('Ctrl Pts',(-0.694214576672374,0.438610418338676,
-6.66238433632284));
#60678=CARTESIAN_POINT('Ctrl Pts',(-0.531017389080337,0.58639555122315,
-6.67124307989611));
#60679=CARTESIAN_POINT('Ctrl Pts',(-0.3678202014883,0.734180684107624,-6.68010182346939));
#60680=CARTESIAN_POINT('Ctrl Pts',(-0.140868175871764,0.808992666571332,
-6.68896056704266));
#60681=CARTESIAN_POINT('Ctrl Pts',(0.0782205473247404,0.787223447298299,
-6.69781931061593));
#60682=CARTESIAN_POINT('Ctrl Pts',(0.297309270521245,0.765454228025267,
-6.7066780541892));
#60683=CARTESIAN_POINT('Ctrl Pts',(0.505102072675574,0.647444880834246,
-6.71553679776247));
#60684=CARTESIAN_POINT('Ctrl Pts',(0.636026795761714,0.470435038100997,
-6.72439554133575));
#60685=CARTESIAN_POINT('Ctrl Pts',(0.766951518847854,0.293425195367748,
-6.73325428490902));
#60686=CARTESIAN_POINT('Ctrl Pts',(0.818956872247066,0.0601881960099669,
-6.74211302848229));
#60687=CARTESIAN_POINT('Ctrl Pts',(0.775631781004217,-0.155674501111215,
-6.75097177205557));
#60688=CARTESIAN_POINT('Ctrl Pts',(0.732306689761369,-0.371537198232396,
-6.75983051562884));
#60689=CARTESIAN_POINT('Ctrl Pts',(0.594329958850246,-0.566643518936463,
-6.76868925920211));
#60690=CARTESIAN_POINT('Ctrl Pts',(0.405242230244082,-0.67942471608472,
-6.77754800277538));
#60691=CARTESIAN_POINT('Ctrl Pts',(0.216154501637919,-0.792205913232977,
-6.78640674634865));
#60692=CARTESIAN_POINT('Ctrl Pts',(-0.0210816529299573,-0.820894963713003,
-6.79526548992193));
#60693=CARTESIAN_POINT('Ctrl Pts',(-0.23160278075316,-0.756438604215441,
-6.8041242334952));
#60694=CARTESIAN_POINT('Ctrl Pts',(-0.442123908576362,-0.691982244717878,
-6.81298297706847));
#60695=CARTESIAN_POINT('Ctrl Pts',(-0.622631625634126,-0.535390358803591,
-6.82184172064174));
#60696=CARTESIAN_POINT('Ctrl Pts',(-0.716163994722123,-0.336077881842366,
-6.83070046421502));
#60697=CARTESIAN_POINT('Ctrl Pts',(-0.765317280859478,-0.231334857514573,
-6.83535592586878));
#60698=CARTESIAN_POINT('Ctrl Pts',(-0.791100000000004,-0.11570283783653,
-6.84001138752254));
#60699=CARTESIAN_POINT('Ctrl Pts',(-0.7911,3.0364599723498E-14,-6.8446668491763));
#60700=CARTESIAN_POINT('Ctrl Pts',(-0.7911,-5.58997292898766E-13,-6.87313315082367));
#60701=CARTESIAN_POINT('Ctrl Pts',(-0.791099999999845,-0.220167589667239,
-6.8642744072504));
#60702=CARTESIAN_POINT('Ctrl Pts',(-0.694214576672059,-0.438610418339179,
-6.85541566367713));
#60703=CARTESIAN_POINT('Ctrl Pts',(-0.531017389079908,-0.586395551223539,
-6.84655692010385));
#60704=CARTESIAN_POINT('Ctrl Pts',(-0.367820201487757,-0.734180684107898,
-6.83769817653058));
#60705=CARTESIAN_POINT('Ctrl Pts',(-0.140868175871157,-0.80899266657144,
-6.82883943295731));
#60706=CARTESIAN_POINT('Ctrl Pts',(0.078220547325339,-0.78722344729824,
-6.81998068938404));
#60707=CARTESIAN_POINT('Ctrl Pts',(0.297309270521835,-0.76545422802504,
-6.81112194581076));
#60708=CARTESIAN_POINT('Ctrl Pts',(0.50510207267608,-0.647444880833854,
-6.80226320223749));
#60709=CARTESIAN_POINT('Ctrl Pts',(0.636026795762085,-0.470435038100496,
-6.79340445866422));
#60710=CARTESIAN_POINT('Ctrl Pts',(0.766951518848091,-0.293425195367137,
-6.78454571509095));
#60711=CARTESIAN_POINT('Ctrl Pts',(0.818956872247117,-0.060188196009305,
-6.77568697151767));
#60712=CARTESIAN_POINT('Ctrl Pts',(0.77563178100409,0.155674501111848,-6.7668282279444));
#60713=CARTESIAN_POINT('Ctrl Pts',(0.732306689761064,0.371537198233002,
-6.75796948437113));
#60714=CARTESIAN_POINT('Ctrl Pts',(0.594329958849773,0.566643518936962,
-6.74911074079786));
#60715=CARTESIAN_POINT('Ctrl Pts',(0.405242230243508,0.679424716085063,
-6.74025199722458));
#60716=CARTESIAN_POINT('Ctrl Pts',(0.216154501637242,0.792205913233164,
-6.73139325365131));
#60717=CARTESIAN_POINT('Ctrl Pts',(-0.0210816529306676,0.820894963712987,
-6.72253451007804));
#60718=CARTESIAN_POINT('Ctrl Pts',(-0.231602780753821,0.756438604215238,
-6.71367576650476));
#60719=CARTESIAN_POINT('Ctrl Pts',(-0.442123908576974,0.691982244717489,
-6.70481702293149));
#60720=CARTESIAN_POINT('Ctrl Pts',(-0.622631625634606,0.535390358803036,
-6.69595827935822));
#60721=CARTESIAN_POINT('Ctrl Pts',(-0.716163994722426,0.33607788184172,
-6.68709953578495));
#60722=CARTESIAN_POINT('Ctrl Pts',(-0.765317280859659,0.231334857513943,
-6.68244407413119));
#60723=CARTESIAN_POINT('Ctrl Pts',(-0.791100000000079,0.115702837835951,
-6.67778861247743));
#60724=CARTESIAN_POINT('Ctrl Pts',(-0.7911,-5.4195536947077E-13,-6.67313315082367));
#60725=CARTESIAN_POINT('Origin',(0.,0.,-5.925));
#60726=CARTESIAN_POINT('',(-0.791106330306829,3.30307559588206E-6,-6.4446668491763));
#60727=CARTESIAN_POINT('',(-0.791564826434644,0.000250487832263192,-6.47313315082367));
#60728=CARTESIAN_POINT('',(-0.7911,-9.68818082805471E-17,-5.925));
#60729=CARTESIAN_POINT('Ctrl Pts',(-0.7911,4.20219414820622E-14,-6.4446668491763));
#60730=CARTESIAN_POINT('Ctrl Pts',(-0.791099999999988,0.220167589666714,
-6.45352559274957));
#60731=CARTESIAN_POINT('Ctrl Pts',(-0.694214576672352,0.438610418338711,
-6.46238433632284));
#60732=CARTESIAN_POINT('Ctrl Pts',(-0.531017389080308,0.586395551223177,
-6.47124307989611));
#60733=CARTESIAN_POINT('Ctrl Pts',(-0.367820201488263,0.734180684107642,
-6.48010182346939));
#60734=CARTESIAN_POINT('Ctrl Pts',(-0.140868175871724,0.808992666571339,
-6.48896056704266));
#60735=CARTESIAN_POINT('Ctrl Pts',(0.0782205473247798,0.787223447298295,
-6.49781931061593));
#60736=CARTESIAN_POINT('Ctrl Pts',(0.297309270521284,0.765454228025252,
-6.5066780541892));
#60737=CARTESIAN_POINT('Ctrl Pts',(0.505102072675606,0.647444880834221,
-6.51553679776248));
#60738=CARTESIAN_POINT('Ctrl Pts',(0.636026795761738,0.470435038100965,
-6.52439554133575));
#60739=CARTESIAN_POINT('Ctrl Pts',(0.766951518847869,0.29342519536771,-6.53325428490902));
#60740=CARTESIAN_POINT('Ctrl Pts',(0.818956872247069,0.0601881960099259,
-6.54211302848229));
#60741=CARTESIAN_POINT('Ctrl Pts',(0.77563178100421,-0.155674501111253,
-6.55097177205557));
#60742=CARTESIAN_POINT('Ctrl Pts',(0.73230668976135,-0.371537198232433,
-6.55983051562884));
#60743=CARTESIAN_POINT('Ctrl Pts',(0.594329958850217,-0.566643518936493,
-6.56868925920211));
#60744=CARTESIAN_POINT('Ctrl Pts',(0.405242230244048,-0.67942471608474,
-6.57754800277538));
#60745=CARTESIAN_POINT('Ctrl Pts',(0.216154501637879,-0.792205913232988,
-6.58640674634866));
#60746=CARTESIAN_POINT('Ctrl Pts',(-0.0210816529299984,-0.820894963713002,
-6.59526548992193));
#60747=CARTESIAN_POINT('Ctrl Pts',(-0.231602780753197,-0.756438604215429,
-6.6041242334952));
#60748=CARTESIAN_POINT('Ctrl Pts',(-0.442123908576397,-0.691982244717856,
-6.61298297706847));
#60749=CARTESIAN_POINT('Ctrl Pts',(-0.622631625634152,-0.53539035880356,
-6.62184172064175));
#60750=CARTESIAN_POINT('Ctrl Pts',(-0.716163994722139,-0.336077881842331,
-6.63070046421502));
#60751=CARTESIAN_POINT('Ctrl Pts',(-0.76531728085948,-0.231334857514555,
-6.63535592586878));
#60752=CARTESIAN_POINT('Ctrl Pts',(-0.7911,-0.115702837836536,-6.64001138752254));
#60753=CARTESIAN_POINT('Ctrl Pts',(-0.7911,2.4980018054066E-15,-6.6446668491763));
#60754=CARTESIAN_POINT('Ctrl Pts',(-0.7911,-5.4195536947077E-13,-6.67313315082367));
#60755=CARTESIAN_POINT('Ctrl Pts',(-0.791099999999849,-0.220167589667214,
-6.6642744072504));
#60756=CARTESIAN_POINT('Ctrl Pts',(-0.694214576672075,-0.43861041833915,
-6.65541566367713));
#60757=CARTESIAN_POINT('Ctrl Pts',(-0.531017389079937,-0.586395551223512,
-6.64655692010386));
#60758=CARTESIAN_POINT('Ctrl Pts',(-0.367820201487799,-0.734180684107875,
-6.63769817653058));
#60759=CARTESIAN_POINT('Ctrl Pts',(-0.140868175871213,-0.808992666571428,
-6.62883943295731));
#60760=CARTESIAN_POINT('Ctrl Pts',(0.0782205473252772,-0.787223447298246,
-6.61998068938404));
#60761=CARTESIAN_POINT('Ctrl Pts',(0.297309270521767,-0.765454228025064,
-6.61112194581077));
#60762=CARTESIAN_POINT('Ctrl Pts',(0.505102072676015,-0.647444880833902,
-6.60226320223749));
#60763=CARTESIAN_POINT('Ctrl Pts',(0.636026795762035,-0.470435038100564,
-6.59340445866422));
#60764=CARTESIAN_POINT('Ctrl Pts',(0.766951518848055,-0.293425195367225,
-6.58454571509095));
#60765=CARTESIAN_POINT('Ctrl Pts',(0.818956872247108,-0.0601881960094084,
-6.57568697151768));
#60766=CARTESIAN_POINT('Ctrl Pts',(0.775631781004111,0.155674501111744,
-6.5668282279444));
#60767=CARTESIAN_POINT('Ctrl Pts',(0.732306689761115,0.371537198232896,
-6.55796948437113));
#60768=CARTESIAN_POINT('Ctrl Pts',(0.594329958849859,0.566643518936868,
-6.54911074079786));
#60769=CARTESIAN_POINT('Ctrl Pts',(0.405242230243619,0.679424716084996,
-6.54025199722459));
#60770=CARTESIAN_POINT('Ctrl Pts',(0.216154501637378,0.792205913233125,
-6.53139325365132));
#60771=CARTESIAN_POINT('Ctrl Pts',(-0.021081652930517,0.820894963712989,
-6.52253451007804));
#60772=CARTESIAN_POINT('Ctrl Pts',(-0.231602780753675,0.756438604215283,
-6.51367576650477));
#60773=CARTESIAN_POINT('Ctrl Pts',(-0.442123908576834,0.691982244717576,
-6.5048170229315));
#60774=CARTESIAN_POINT('Ctrl Pts',(-0.622631625634491,0.535390358803167,
-6.49595827935823));
#60775=CARTESIAN_POINT('Ctrl Pts',(-0.716163994722352,0.336077881841878,
-6.48709953578495));
#60776=CARTESIAN_POINT('Ctrl Pts',(-0.76531728085963,0.231334857514065,
-6.48244407413119));
#60777=CARTESIAN_POINT('Ctrl Pts',(-0.791100000000077,0.115702837836021,
-6.47778861247743));
#60778=CARTESIAN_POINT('Ctrl Pts',(-0.7911,-5.24857934891543E-13,-6.47313315082367));
#60779=CARTESIAN_POINT('Origin',(0.,0.,-5.925));
#60780=CARTESIAN_POINT('',(-0.791105591446152,0.000150202279374845,-6.2446668491763));
#60781=CARTESIAN_POINT('',(-0.789646943890772,0.00034450190664909,-6.27313315082367));
#60782=CARTESIAN_POINT('',(-0.7911,-9.68818082805471E-17,-5.925));
#60783=CARTESIAN_POINT('Ctrl Pts',(-0.791105591446152,0.000150202279374845,
-6.2446668491763));
#60784=CARTESIAN_POINT('Ctrl Pts',(-0.79144237439907,0.0923771225581108,
-6.24836903705538));
#60785=CARTESIAN_POINT('Ctrl Pts',(-0.775893102399071,0.184576764100862,
-6.25207122493447));
#60786=CARTESIAN_POINT('Ctrl Pts',(-0.744247893335028,0.270759032458304,
-6.25577341281355));
#60787=CARTESIAN_POINT('Ctrl Pts',(-0.653718590646796,0.517305694314754,
-6.26636447847648));
#60788=CARTESIAN_POINT('Ctrl Pts',(-0.431461112281039,0.714606537868241,
-6.27695554413941));
#60789=CARTESIAN_POINT('Ctrl Pts',(-0.176182923218375,0.772665632828024,
-6.28754660980234));
#60790=CARTESIAN_POINT('Ctrl Pts',(0.0790952658442903,0.830724727787806,
-6.29813767546527));
#60791=CARTESIAN_POINT('Ctrl Pts',(0.367394165603863,0.749542074153883,
-6.3087287411282));
#60792=CARTESIAN_POINT('Ctrl Pts',(0.554559547305794,0.56635654910048,-6.31931980679113));
#60793=CARTESIAN_POINT('Ctrl Pts',(0.741724929007724,0.383171024047077,
-6.32991087245406));
#60794=CARTESIAN_POINT('Ctrl Pts',(0.827756792652013,0.0979826275741944,
-6.34050193811698));
#60795=CARTESIAN_POINT('Ctrl Pts',(0.775857090223025,-0.158950432914308,
-6.35109300377991));
#60796=CARTESIAN_POINT('Ctrl Pts',(0.749907239008532,-0.287416963158559,
-6.35638853661138));
#60797=CARTESIAN_POINT('Ctrl Pts',(0.689474496275719,-0.408819659406715,
-6.36168406944284));
#60798=CARTESIAN_POINT('Ctrl Pts',(0.604249241889583,-0.509732962576653,
-6.36697960227431));
#60799=CARTESIAN_POINT('Ctrl Pts',(0.519023987503447,-0.61064626574659,
-6.37227513510577));
#60800=CARTESIAN_POINT('Ctrl Pts',(0.409006221463986,-0.691070175838309,
-6.37757066793724));
#60801=CARTESIAN_POINT('Ctrl Pts',(0.286695534736869,-0.738360975552133,
-6.3828662007687));
#60802=CARTESIAN_POINT('Ctrl Pts',(0.0420741612826401,-0.832942574979778,
-6.39345726643163));
#60803=CARTESIAN_POINT('Ctrl Pts',(-0.251718894922216,-0.794991732895852,
-6.40404833209456));
#60804=CARTESIAN_POINT('Ctrl Pts',(-0.464779911730617,-0.641354845576358,
-6.41463939775749));
#60805=CARTESIAN_POINT('Ctrl Pts',(-0.57131042013482,-0.564536401916609,
-6.41993493058895));
#60806=CARTESIAN_POINT('Ctrl Pts',(-0.657657918689909,-0.458796446947966,
-6.42523046342042));
#60807=CARTESIAN_POINT('Ctrl Pts',(-0.714173715474753,-0.339574174989383,
-6.43052599625189));
#60808=CARTESIAN_POINT('Ctrl Pts',(-0.764479107816768,-0.233452992807072,
-6.43523961389336));
#60809=CARTESIAN_POINT('Ctrl Pts',(-0.791148858337168,-0.116649777874704,
-6.43995323153483));
#60810=CARTESIAN_POINT('Ctrl Pts',(-0.791304868704775,0.000106897948089511,
-6.4446668491763));
#60811=CARTESIAN_POINT('Ctrl Pts',(-0.792405686160893,0.000703614237492454,
-6.47313315082367));
#60812=CARTESIAN_POINT('Ctrl Pts',(-0.790931820918324,-0.240478805143301,
-6.46339213985864));
#60813=CARTESIAN_POINT('Ctrl Pts',(-0.672291318622103,-0.48357032053066,
-6.4536511288936));
#60814=CARTESIAN_POINT('Ctrl Pts',(-0.481013815618491,-0.629823575980568,
-6.44391011792856));
#60815=CARTESIAN_POINT('Ctrl Pts',(-0.273044375749921,-0.788839702483944,
-6.43331905226563));
#60816=CARTESIAN_POINT('Ctrl Pts',(0.0207926315836592,-0.833378830523809,
-6.4227279866027));
#60817=CARTESIAN_POINT('Ctrl Pts',(0.268185334101307,-0.745178944639886,
-6.41213692093977));
#60818=CARTESIAN_POINT('Ctrl Pts',(0.39188168536012,-0.701079001697929,
-6.40684138810831));
#60819=CARTESIAN_POINT('Ctrl Pts',(0.50396696041495,-0.623794305275027,
-6.40154585527685));
#60820=CARTESIAN_POINT('Ctrl Pts',(0.591355703565141,-0.525014117087408,
-6.39625032244538));
#60821=CARTESIAN_POINT('Ctrl Pts',(0.678744446715342,-0.426233928899778,
-6.39095478961392));
#60822=CARTESIAN_POINT('Ctrl Pts',(0.741436657960902,-0.305958248947421,
-6.38565925678245));
#60823=CARTESIAN_POINT('Ctrl Pts',(0.771015028956397,-0.178163093565044,
-6.38036372395099));
#60824=CARTESIAN_POINT('Ctrl Pts',(0.800593399951893,-0.0503679381826663,
-6.37506819111952));
#60825=CARTESIAN_POINT('Ctrl Pts',(0.797057930697324,0.084946692629738,
-6.36977265828806));
#60826=CARTESIAN_POINT('Ctrl Pts',(0.761820860783038,0.212093593185943,
-6.36447712545659));
#60827=CARTESIAN_POINT('Ctrl Pts',(0.726583790868755,0.339240493742134,
-6.35918159262512));
#60828=CARTESIAN_POINT('Ctrl Pts',(0.659645120294761,0.458219664042133,
-6.35388605979366));
#60829=CARTESIAN_POINT('Ctrl Pts',(0.567863458218445,0.552166186136732,
-6.3485905269622));
#60830=CARTESIAN_POINT('Ctrl Pts',(0.384300134065797,0.740059230325945,
-6.33799946129927));
#60831=CARTESIAN_POINT('Ctrl Pts',(0.101364843903861,0.827821681693549,
-6.32740839563635));
#60832=CARTESIAN_POINT('Ctrl Pts',(-0.155850887918912,0.776583389335134,
-6.31681732997342));
#60833=CARTESIAN_POINT('Ctrl Pts',(-0.284458753830295,0.750964243155928,
-6.31152179714195));
#60834=CARTESIAN_POINT('Ctrl Pts',(-0.406636730156887,0.690594911045214,
-6.30622626431048));
#60835=CARTESIAN_POINT('Ctrl Pts',(-0.50790244458249,0.60578869768958,-6.30093073147902));
#60836=CARTESIAN_POINT('Ctrl Pts',(-0.609168159008086,0.520982484333951,
-6.29563519864755));
#60837=CARTESIAN_POINT('Ctrl Pts',(-0.689521611532702,0.411739389733399,
-6.29033966581609));
#60838=CARTESIAN_POINT('Ctrl Pts',(-0.737113985579674,0.289624648184222,
-6.28504413298462));
#60839=CARTESIAN_POINT('Ctrl Pts',(-0.77279638281976,0.198069082737379,
-6.28107380559764));
#60840=CARTESIAN_POINT('Ctrl Pts',(-0.790062941498036,0.0992780359435954,
-6.27710347821066));
#60841=CARTESIAN_POINT('Ctrl Pts',(-0.789646943890772,0.00034450190664909,
-6.27313315082367));
#60842=CARTESIAN_POINT('Origin',(0.,0.,-5.925));
#60843=CARTESIAN_POINT('',(-0.790663869694179,-0.000319622920649363,-6.0446668491763));
#60844=CARTESIAN_POINT('',(-0.790931871961626,-0.000575333837205039,-6.07313315082367));
#60845=CARTESIAN_POINT('',(-0.7911,-9.68818082805471E-17,-5.925));
#60846=CARTESIAN_POINT('Ctrl Pts',(-0.79027278667866,-0.00060623243642971,
-6.0446668491763));
#60847=CARTESIAN_POINT('Ctrl Pts',(-0.789239692543626,0.169353443234173,
-6.05148930974447));
#60848=CARTESIAN_POINT('Ctrl Pts',(-0.735523539619875,0.339963444333918,
-6.05831177031265));
#60849=CARTESIAN_POINT('Ctrl Pts',(-0.634255164638182,0.475084083996859,
-6.06513423088083));
#60850=CARTESIAN_POINT('Ctrl Pts',(-0.477047952036308,0.684842946329087,
-6.07572529654376));
#60851=CARTESIAN_POINT('Ctrl Pts',(-0.205245106273596,0.809076344901306,
-6.08631636220669));
#60852=CARTESIAN_POINT('Ctrl Pts',(0.0559109762185824,0.790524027970827,
-6.09690742786962));
#60853=CARTESIAN_POINT('Ctrl Pts',(0.317067058710761,0.771971711040347,
-6.10749849353255));
#60854=CARTESIAN_POINT('Ctrl Pts',(0.567576377932405,0.610633678607169,
-6.11808955919547));
#60855=CARTESIAN_POINT('Ctrl Pts',(0.694329353803112,0.381187901319921,
-6.1286806248584));
#60856=CARTESIAN_POINT('Ctrl Pts',(0.757705841738466,0.266465012676297,
-6.13397615768987));
#60857=CARTESIAN_POINT('Ctrl Pts',(0.790143243836085,0.134715187819156,
-6.13927169052133));
#60858=CARTESIAN_POINT('Ctrl Pts',(0.790491482816431,0.0026078004279992,
-6.14456722335279));
#60859=CARTESIAN_POINT('Ctrl Pts',(0.790839721796777,-0.129499586963158,
-6.14986275618426));
#60860=CARTESIAN_POINT('Ctrl Pts',(0.759098797659849,-0.261964536888331,
-6.15515828901573));
#60861=CARTESIAN_POINT('Ctrl Pts',(0.696510600452876,-0.377164033684325,
-6.1604538218472));
#60862=CARTESIAN_POINT('Ctrl Pts',(0.57133420603893,-0.607563027276312,
-6.17104488751013));
#60863=CARTESIAN_POINT('Ctrl Pts',(0.322768719344804,-0.76890020835158,
-6.18163595317304));
#60864=CARTESIAN_POINT('Ctrl Pts',(0.0609180238672261,-0.789725501077674,
-6.19222701883598));
#60865=CARTESIAN_POINT('Ctrl Pts',(-0.0700073238715702,-0.800138147440722,
-6.19752255166744));
#60866=CARTESIAN_POINT('Ctrl Pts',(-0.20425397380623,-0.775422821716471,
-6.20281808449891));
#60867=CARTESIAN_POINT('Ctrl Pts',(-0.324505308412596,-0.721134851061482,
-6.20811361733038));
#60868=CARTESIAN_POINT('Ctrl Pts',(-0.444756643018949,-0.666846880406498,
-6.21340915016184));
#60869=CARTESIAN_POINT('Ctrl Pts',(-0.551012662297012,-0.582986264820781,
-6.2187046829933));
#60870=CARTESIAN_POINT('Ctrl Pts',(-0.630292184928299,-0.478482327068392,
-6.22400021582476));
#60871=CARTESIAN_POINT('Ctrl Pts',(-0.70957170755959,-0.373978389315996,
-6.22929574865623));
#60872=CARTESIAN_POINT('Ctrl Pts',(-0.761874733544102,-0.248831129396924,
-6.23459128148769));
#60873=CARTESIAN_POINT('Ctrl Pts',(-0.78185994282399,-0.118465106685406,
-6.23988681431916));
#60874=CARTESIAN_POINT('Ctrl Pts',(-0.78787318707,-0.079239961480945,-6.24148015927154));
#60875=CARTESIAN_POINT('Ctrl Pts',(-0.79096064704149,-0.0395423532307859,
-6.24307350422392));
#60876=CARTESIAN_POINT('Ctrl Pts',(-0.791105591446152,0.000150202279374845,
-6.2446668491763));
#60877=CARTESIAN_POINT('Ctrl Pts',(-0.789646943890772,0.00034450190664909,
-6.27313315082367));
#60878=CARTESIAN_POINT('Ctrl Pts',(-0.7889532451066,-0.164632582280567,
-6.26651241254773));
#60879=CARTESIAN_POINT('Ctrl Pts',(-0.739088975450182,-0.330005886277594,
-6.25989167427178));
#60880=CARTESIAN_POINT('Ctrl Pts',(-0.643454389938275,-0.462884953618257,
-6.25327093599584));
#60881=CARTESIAN_POINT('Ctrl Pts',(-0.490469612019563,-0.67544900142945,
-6.24267987033291));
#60882=CARTESIAN_POINT('Ctrl Pts',(-0.220359621998779,-0.804861026158961,
-6.23208880466998));
#60883=CARTESIAN_POINT('Ctrl Pts',(0.0410929792480928,-0.791431595050273,
-6.22149773900705));
#60884=CARTESIAN_POINT('Ctrl Pts',(0.30254558049498,-0.778002163941584,
-6.21090667334412));
#60885=CARTESIAN_POINT('Ctrl Pts',(0.555340792967953,-0.621731276994677,
-6.20031560768119));
#60886=CARTESIAN_POINT('Ctrl Pts',(0.68680223501153,-0.394357794869774,
-6.18972454201826));
#60887=CARTESIAN_POINT('Ctrl Pts',(0.752532956033317,-0.280671053807326,
-6.1844290091868));
#60888=CARTESIAN_POINT('Ctrl Pts',(0.787930234447756,-0.14920866395038,
-6.17913347635533));
#60889=CARTESIAN_POINT('Ctrl Pts',(0.790593478787117,-0.0173465556812871,
-6.17383794352387));
#60890=CARTESIAN_POINT('Ctrl Pts',(0.793256723126477,0.114515552587806,
-6.1685424106924));
#60891=CARTESIAN_POINT('Ctrl Pts',(0.763185933390757,0.246777379269046,
-6.16324687786094));
#60892=CARTESIAN_POINT('Ctrl Pts',(0.702998643332439,0.363326964552898,
-6.15795134502948));
#60893=CARTESIAN_POINT('Ctrl Pts',(0.642811353274121,0.47987654983675,-6.15265581219801));
#60894=CARTESIAN_POINT('Ctrl Pts',(0.552507562893205,0.580713893723215,
-6.14736027936654));
#60895=CARTESIAN_POINT('Ctrl Pts',(0.443345199926037,0.654816159166802,
-6.14206474653508));
#60896=CARTESIAN_POINT('Ctrl Pts',(0.33418283695887,0.728918424610389,-6.13676921370361));
#60897=CARTESIAN_POINT('Ctrl Pts',(0.206161901405452,0.776285611611098,
-6.13147368087215));
#60898=CARTESIAN_POINT('Ctrl Pts',(0.0753900581244591,0.788475561967689,
-6.12617814804069));
#60899=CARTESIAN_POINT('Ctrl Pts',(-0.186153628437527,0.81285546268087,
-6.11558708237776));
#60900=CARTESIAN_POINT('Ctrl Pts',(-0.458700945909811,0.696526416817579,
-6.10499601671483));
#60901=CARTESIAN_POINT('Ctrl Pts',(-0.621527725141712,0.49100204859901,
-6.0944049510519));
#60902=CARTESIAN_POINT('Ctrl Pts',(-0.702941114757658,0.388239864489732,
-6.08910941822044));
#60903=CARTESIAN_POINT('Ctrl Pts',(-0.756924369813512,0.263178849791636,
-6.08381388538897));
#60904=CARTESIAN_POINT('Ctrl Pts',(-0.77923235736188,0.132968109968668,
-6.0785183525575));
#60905=CARTESIAN_POINT('Ctrl Pts',(-0.786794266430465,0.0888295801187872,
-6.07672328531289));
#60906=CARTESIAN_POINT('Ctrl Pts',(-0.790716502172883,0.044099316760431,
-6.07492821806828));
#60907=CARTESIAN_POINT('Ctrl Pts',(-0.790931871961626,-0.000575333837205039,
-6.07313315082367));
#60908=CARTESIAN_POINT('Origin',(0.,0.,-5.925));
#60909=CARTESIAN_POINT('',(-0.7911,9.31477117660506E-14,-5.8446668491763));
#60910=CARTESIAN_POINT('',(-0.792458596363369,-0.000371319283420802,-5.87313315082368));
#60911=CARTESIAN_POINT('',(-0.7911,-9.68818082805471E-17,-5.925));
#60912=CARTESIAN_POINT('Ctrl Pts',(-0.7911,9.31477117660506E-14,-5.8446668491763));
#60913=CARTESIAN_POINT('Ctrl Pts',(-0.791099999999974,0.220167589666758,
-5.85352559274957));
#60914=CARTESIAN_POINT('Ctrl Pts',(-0.694214576672331,0.438610418338741,
-5.86238433632284));
#60915=CARTESIAN_POINT('Ctrl Pts',(-0.531017389080286,0.586395551223196,
-5.87124307989612));
#60916=CARTESIAN_POINT('Ctrl Pts',(-0.367820201488242,0.734180684107651,
-5.88010182346939));
#60917=CARTESIAN_POINT('Ctrl Pts',(-0.14086817587171,0.808992666571339,
-5.88896056704266));
#60918=CARTESIAN_POINT('Ctrl Pts',(0.0782205473247859,0.787223447298295,
-5.89781931061593));
#60919=CARTESIAN_POINT('Ctrl Pts',(0.297309270521282,0.76545422802525,-5.9066780541892));
#60920=CARTESIAN_POINT('Ctrl Pts',(0.505102072675597,0.647444880834226,
-5.91553679776248));
#60921=CARTESIAN_POINT('Ctrl Pts',(0.636026795761728,0.470435038100979,
-5.92439554133575));
#60922=CARTESIAN_POINT('Ctrl Pts',(0.766951518847859,0.293425195367732,
-5.93325428490902));
#60923=CARTESIAN_POINT('Ctrl Pts',(0.818956872247065,0.0601881960099587,
-5.94211302848229));
#60924=CARTESIAN_POINT('Ctrl Pts',(0.775631781004217,-0.155674501111215,
-5.95097177205556));
#60925=CARTESIAN_POINT('Ctrl Pts',(0.73230668976137,-0.37153719823239,-5.95983051562884));
#60926=CARTESIAN_POINT('Ctrl Pts',(0.594329958850255,-0.56664351893645,
-5.96868925920211));
#60927=CARTESIAN_POINT('Ctrl Pts',(0.405242230244101,-0.679424716084709,
-5.97754800277538));
#60928=CARTESIAN_POINT('Ctrl Pts',(0.216154501637947,-0.792205913232967,
-5.98640674634865));
#60929=CARTESIAN_POINT('Ctrl Pts',(-0.0210816529299185,-0.820894963713002,
-5.99526548992193));
#60930=CARTESIAN_POINT('Ctrl Pts',(-0.231602780753117,-0.756438604215453,
-6.0041242334952));
#60931=CARTESIAN_POINT('Ctrl Pts',(-0.442123908576316,-0.691982244717905,
-6.01298297706847));
#60932=CARTESIAN_POINT('Ctrl Pts',(-0.622631625634084,-0.535390358803637,
-6.02184172064174));
#60933=CARTESIAN_POINT('Ctrl Pts',(-0.716163994722094,-0.336077881842427,
-6.03070046421501));
#60934=CARTESIAN_POINT('Ctrl Pts',(-0.765317280859475,-0.231334857514603,
-6.03535592586878));
#60935=CARTESIAN_POINT('Ctrl Pts',(-0.791100000000011,-0.115702837836522,
-6.04001138752254));
#60936=CARTESIAN_POINT('Ctrl Pts',(-0.7911,7.60502771868232E-14,-6.0446668491763));
#60937=CARTESIAN_POINT('Ctrl Pts',(-0.790931871961626,-0.000575333837205039,
-6.07313315082367));
#60938=CARTESIAN_POINT('Ctrl Pts',(-0.791351853183058,-0.0876930044934924,
-6.06963268523682));
#60939=CARTESIAN_POINT('Ctrl Pts',(-0.777675796400345,-0.174599197422119,
-6.06613221964997));
#60940=CARTESIAN_POINT('Ctrl Pts',(-0.749405440614064,-0.256493573493322,
-6.06263175406311));
#60941=CARTESIAN_POINT('Ctrl Pts',(-0.663870191939938,-0.504274530875614,
-6.05204068840018));
#60942=CARTESIAN_POINT('Ctrl Pts',(-0.444733565754056,-0.706175543231099,
-6.04144962273725));
#60943=CARTESIAN_POINT('Ctrl Pts',(-0.190625871903937,-0.769230819079553,
-6.03085855707432));
#60944=CARTESIAN_POINT('Ctrl Pts',(0.063481821946182,-0.832286094928007,
-6.02026749141139));
#60945=CARTESIAN_POINT('Ctrl Pts',(0.352560583460537,-0.75649563426943,
-6.00967642574847));
#60946=CARTESIAN_POINT('Ctrl Pts',(0.543404894746757,-0.576797729800151,
-5.99908536008554));
#60947=CARTESIAN_POINT('Ctrl Pts',(0.734249206032977,-0.397099825330873,
-5.98849429442261));
#60948=CARTESIAN_POINT('Ctrl Pts',(0.826859067091062,-0.113494477050894,
-5.97790322875968));
#60949=CARTESIAN_POINT('Ctrl Pts',(0.779142391420507,0.144110508626454,
-5.96731216309675));
#60950=CARTESIAN_POINT('Ctrl Pts',(0.731425715749952,0.401715494303803,
-5.95672109743382));
#60951=CARTESIAN_POINT('Ctrl Pts',(0.543382503350756,0.633320117378521,
-5.94613003177089));
#60952=CARTESIAN_POINT('Ctrl Pts',(0.301070755401524,0.732930491279356,
-5.93553896610796));
#60953=CARTESIAN_POINT('Ctrl Pts',(0.0587590074522929,0.83254086518019,
-5.92494790044503));
#60954=CARTESIAN_POINT('Ctrl Pts',(-0.237821276046974,0.800156989907141,
-5.9143568347821));
#60955=CARTESIAN_POINT('Ctrl Pts',(-0.452886511529511,0.650290941357769,
-5.90376576911917));
#60956=CARTESIAN_POINT('Ctrl Pts',(-0.660231440322552,0.50580471095775,
-5.89355489635401));
#60957=CARTESIAN_POINT('Ctrl Pts',(-0.791808652946734,0.252119551325989,
-5.88334402358884));
#60958=CARTESIAN_POINT('Ctrl Pts',(-0.792458596363369,-0.000371319283420802,
-5.87313315082368));
#60959=CARTESIAN_POINT('Origin',(0.,0.,-5.925));
#60960=CARTESIAN_POINT('',(-0.7911,1.10300657496509E-13,-5.6446668491763));
#60961=CARTESIAN_POINT('',(-0.790982034689833,0.00049980459233876,-5.67313315082368));
#60962=CARTESIAN_POINT('',(-0.7911,-9.68818082805471E-17,-5.925));
#60963=CARTESIAN_POINT('Ctrl Pts',(-0.7911,1.10300657496509E-13,-5.6446668491763));
#60964=CARTESIAN_POINT('Ctrl Pts',(-0.791099999999969,0.22016758966679,
-5.65352559274957));
#60965=CARTESIAN_POINT('Ctrl Pts',(-0.694214576672307,0.438610418338786,
-5.66238433632285));
#60966=CARTESIAN_POINT('Ctrl Pts',(-0.53101738908024,0.586395551223237,
-5.67124307989612));
#60967=CARTESIAN_POINT('Ctrl Pts',(-0.367820201488173,0.734180684107689,
-5.68010182346939));
#60968=CARTESIAN_POINT('Ctrl Pts',(-0.140868175871616,0.808992666571359,
-5.68896056704266));
#60969=CARTESIAN_POINT('Ctrl Pts',(0.0782205473248925,0.787223447298284,
-5.69781931061594));
#60970=CARTESIAN_POINT('Ctrl Pts',(0.297309270521401,0.765454228025208,
-5.70667805418921));
#60971=CARTESIAN_POINT('Ctrl Pts',(0.505102072675713,0.647444880834141,
-5.71553679776248));
#60972=CARTESIAN_POINT('Ctrl Pts',(0.636026795761818,0.470435038100856,
-5.72439554133575));
#60973=CARTESIAN_POINT('Ctrl Pts',(0.766951518847924,0.293425195367572,
-5.73325428490903));
#60974=CARTESIAN_POINT('Ctrl Pts',(0.818956872247083,0.0601881960097696,
-5.7421130284823));
#60975=CARTESIAN_POINT('Ctrl Pts',(0.775631781004179,-0.155674501111408,
-5.75097177205557));
#60976=CARTESIAN_POINT('Ctrl Pts',(0.732306689761274,-0.371537198232586,
-5.75983051562884));
#60977=CARTESIAN_POINT('Ctrl Pts',(0.594329958850094,-0.566643518936625,
-5.76868925920212));
#60978=CARTESIAN_POINT('Ctrl Pts',(0.405242230243893,-0.679424716084833,
-5.77754800277539));
#60979=CARTESIAN_POINT('Ctrl Pts',(0.216154501637692,-0.792205913233041,
-5.78640674634866));
#60980=CARTESIAN_POINT('Ctrl Pts',(-0.0210816529302019,-0.820894963712999,
-5.79526548992194));
#60981=CARTESIAN_POINT('Ctrl Pts',(-0.231602780753392,-0.756438604215369,
-5.80412423349521));
#60982=CARTESIAN_POINT('Ctrl Pts',(-0.442123908576581,-0.69198224471774,
-5.81298297706848));
#60983=CARTESIAN_POINT('Ctrl Pts',(-0.622631625634302,-0.535390358803389,
-5.82184172064175));
#60984=CARTESIAN_POINT('Ctrl Pts',(-0.716163994722235,-0.336077881842126,
-5.83070046421503));
#60985=CARTESIAN_POINT('Ctrl Pts',(-0.765317280859527,-0.231334857514377,
-5.83535592586878));
#60986=CARTESIAN_POINT('Ctrl Pts',(-0.791100000000014,-0.1157028378364,
-5.84001138752254));
#60987=CARTESIAN_POINT('Ctrl Pts',(-0.7911,9.31477117660506E-14,-5.8446668491763));
#60988=CARTESIAN_POINT('Ctrl Pts',(-0.792458596363369,-0.000371319283420802,
-5.87313315082368));
#60989=CARTESIAN_POINT('Ctrl Pts',(-0.792482796436823,-0.00977259554683975,
-5.87275295792591));
#60990=CARTESIAN_POINT('Ctrl Pts',(-0.792325481568797,-0.0191722160718984,
-5.87237276502815));
#60991=CARTESIAN_POINT('Ctrl Pts',(-0.791983804387725,-0.0285644822897483,
-5.87199257213039));
#60992=CARTESIAN_POINT('Ctrl Pts',(-0.782465674297599,-0.290205635562192,
-5.86140150646746));
#60993=CARTESIAN_POINT('Ctrl Pts',(-0.629879226651533,-0.546139720281407,
-5.85081044080453));
#60994=CARTESIAN_POINT('Ctrl Pts',(-0.404949836955553,-0.680744516845347,
-5.8402193751416));
#60995=CARTESIAN_POINT('Ctrl Pts',(-0.292485142107553,-0.748046915127322,
-5.83492384231014));
#60996=CARTESIAN_POINT('Ctrl Pts',(-0.161934711747093,-0.785016991370474,
-5.82962830947867));
#60997=CARTESIAN_POINT('Ctrl Pts',(-0.0299182311690132,-0.789929417398865,
-5.82433277664721));
#60998=CARTESIAN_POINT('Ctrl Pts',(0.102098249409059,-0.794841843427256,
-5.81903724381574));
#60999=CARTESIAN_POINT('Ctrl Pts',(0.235580780204725,-0.767696619240881,
-5.81374171098428));
#61000=CARTESIAN_POINT('Ctrl Pts',(0.352873959307637,-0.709126006920355,
-5.80844617815281));
#61001=CARTESIAN_POINT('Ctrl Pts',(0.587460317513463,-0.591984782279301,
-5.79785511248988));
#61002=CARTESIAN_POINT('Ctrl Pts',(0.757289268948261,-0.349142005101648,
-5.78726404682695));
#61003=CARTESIAN_POINT('Ctrl Pts',(0.787149237372238,-0.0881671752330585,
-5.77667298116402));
#61004=CARTESIAN_POINT('Ctrl Pts',(0.802079221584226,0.0423202397012362,
-5.77137744833256));
#61005=CARTESIAN_POINT('Ctrl Pts',(0.782016960043503,0.177340667808283,
-5.7660819155011));
#61006=CARTESIAN_POINT('Ctrl Pts',(0.731916162847515,0.29939589036256,-5.76078638266963));
#61007=CARTESIAN_POINT('Ctrl Pts',(0.68181536565153,0.42145111291683,-5.75549084983817));
#61008=CARTESIAN_POINT('Ctrl Pts',(0.601676032800284,0.530541129918351,
-5.7501953170067));
#61009=CARTESIAN_POINT('Ctrl Pts',(0.499973647650632,0.613383996655761,
-5.74489978417524));
#61010=CARTESIAN_POINT('Ctrl Pts',(0.398271262500969,0.69622686339318,-5.73960425134377));
#61011=CARTESIAN_POINT('Ctrl Pts',(0.2750058250529,0.752822579866479,-5.73430871851231));
#61012=CARTESIAN_POINT('Ctrl Pts',(0.145408139388317,0.777300086642441,
-5.72901318568084));
#61013=CARTESIAN_POINT('Ctrl Pts',(0.0158104537237486,0.8017775934184,-5.72371765284938));
#61014=CARTESIAN_POINT('Ctrl Pts',(-0.120119480157327,0.794136890497028,
-5.71842212001791));
#61015=CARTESIAN_POINT('Ctrl Pts',(-0.244883133276068,0.753158437135428,
-5.71312658718645));
#61016=CARTESIAN_POINT('Ctrl Pts',(-0.49441043951357,0.67120153041222,-5.70253552152352));
#61017=CARTESIAN_POINT('Ctrl Pts',(-0.699272622701712,0.455893621928078,
-5.69194445586059));
#61018=CARTESIAN_POINT('Ctrl Pts',(-0.766117078544422,0.202773826096619,
-5.68135339019766));
#61019=CARTESIAN_POINT('Ctrl Pts',(-0.783410819178852,0.137287645629397,
-5.67861331040633));
#61020=CARTESIAN_POINT('Ctrl Pts',(-0.791466474469695,0.0692705624365982,
-5.67587323061501));
#61021=CARTESIAN_POINT('Ctrl Pts',(-0.79084825614368,0.00106660793215366,
-5.67313315082368));
#61022=CARTESIAN_POINT('Origin',(0.,0.,-5.925));
#61023=CARTESIAN_POINT('',(-0.790955350306868,1.92250298529111E-5,-5.4446668491763));
#61024=CARTESIAN_POINT('',(-0.79043867098578,-0.000255047988537571,-5.47313315082368));
#61025=CARTESIAN_POINT('',(-0.7911,-9.68818082805471E-17,-5.925));
#61026=CARTESIAN_POINT('Ctrl Pts',(-0.7911,1.27342580924505E-13,-5.4446668491763));
#61027=CARTESIAN_POINT('Ctrl Pts',(-0.791099999999964,0.220167589666792,
-5.45352559274957));
#61028=CARTESIAN_POINT('Ctrl Pts',(-0.694214576672312,0.438610418338771,
-5.46238433632285));
#61029=CARTESIAN_POINT('Ctrl Pts',(-0.531017389080261,0.586395551223219,
-5.47124307989612));
#61030=CARTESIAN_POINT('Ctrl Pts',(-0.36782020148821,0.734180684107666,
-5.48010182346939));
#61031=CARTESIAN_POINT('Ctrl Pts',(-0.140868175871675,0.808992666571345,
-5.48896056704266));
#61032=CARTESIAN_POINT('Ctrl Pts',(0.0782205473248199,0.787223447298291,
-5.49781931061593));
#61033=CARTESIAN_POINT('Ctrl Pts',(0.297309270521315,0.765454228025237,
-5.50667805418921));
#61034=CARTESIAN_POINT('Ctrl Pts',(0.505102072675625,0.647444880834204,
-5.51553679776248));
#61035=CARTESIAN_POINT('Ctrl Pts',(0.636026795761748,0.470435038100951,
-5.52439554133575));
#61036=CARTESIAN_POINT('Ctrl Pts',(0.766951518847871,0.293425195367699,
-5.53325428490902));
#61037=CARTESIAN_POINT('Ctrl Pts',(0.818956872247068,0.0601881960099234,
-5.54211302848229));
#61038=CARTESIAN_POINT('Ctrl Pts',(0.775631781004211,-0.155674501111249,
-5.55097177205557));
#61039=CARTESIAN_POINT('Ctrl Pts',(0.732306689761354,-0.371537198232421,
-5.55983051562884));
#61040=CARTESIAN_POINT('Ctrl Pts',(0.59432995885023,-0.566643518936476,
-5.56868925920211));
#61041=CARTESIAN_POINT('Ctrl Pts',(0.405242230244071,-0.679424716084726,
-5.57754800277538));
#61042=CARTESIAN_POINT('Ctrl Pts',(0.216154501637913,-0.792205913232977,
-5.58640674634866));
#61043=CARTESIAN_POINT('Ctrl Pts',(-0.021081652929954,-0.820894963713001,
-5.59526548992193));
#61044=CARTESIAN_POINT('Ctrl Pts',(-0.23160278075315,-0.756438604215443,
-5.6041242334952));
#61045=CARTESIAN_POINT('Ctrl Pts',(-0.442123908576346,-0.691982244717885,
-5.61298297706847));
#61046=CARTESIAN_POINT('Ctrl Pts',(-0.622631625634107,-0.53539035880361,
-5.62184172064174));
#61047=CARTESIAN_POINT('Ctrl Pts',(-0.716163994722109,-0.336077881842396,
-5.63070046421501));
#61048=CARTESIAN_POINT('Ctrl Pts',(-0.765317280859485,-0.23133485751457,
-5.63535592586878));
#61049=CARTESIAN_POINT('Ctrl Pts',(-0.791100000000016,-0.115702837836488,
-5.64001138752254));
#61050=CARTESIAN_POINT('Ctrl Pts',(-0.7911,1.10300657496509E-13,-5.6446668491763));
#61051=CARTESIAN_POINT('Ctrl Pts',(-0.7911,-4.56634730028327E-13,-5.67313315082368));
#61052=CARTESIAN_POINT('Ctrl Pts',(-0.791099999999873,-0.220167589667121,
-5.6642744072504));
#61053=CARTESIAN_POINT('Ctrl Pts',(-0.694214576672129,-0.43861041833906,
-5.65541566367713));
#61054=CARTESIAN_POINT('Ctrl Pts',(-0.531017389080017,-0.58639555122344,
-5.64655692010386));
#61055=CARTESIAN_POINT('Ctrl Pts',(-0.367820201487905,-0.73418068410782,
-5.63769817653059));
#61056=CARTESIAN_POINT('Ctrl Pts',(-0.140868175871339,-0.808992666571404,
-5.62883943295732));
#61057=CARTESIAN_POINT('Ctrl Pts',(0.0782205473251476,-0.787223447298259,
-5.61998068938404));
#61058=CARTESIAN_POINT('Ctrl Pts',(0.297309270521634,-0.765454228025114,
-5.61112194581077));
#61059=CARTESIAN_POINT('Ctrl Pts',(0.505102072675895,-0.647444880833994,
-5.6022632022375));
#61060=CARTESIAN_POINT('Ctrl Pts',(0.636026795761944,-0.470435038100687,
-5.59340445866423));
#61061=CARTESIAN_POINT('Ctrl Pts',(0.766951518847994,-0.293425195367379,
-5.58454571509096));
#61062=CARTESIAN_POINT('Ctrl Pts',(0.818956872247093,-0.0601881960095824,
-5.57568697151768));
#61063=CARTESIAN_POINT('Ctrl Pts',(0.775631781004146,0.155674501111572,
-5.56682822794441));
#61064=CARTESIAN_POINT('Ctrl Pts',(0.732306689761199,0.371537198232726,
-5.55796948437114));
#61065=CARTESIAN_POINT('Ctrl Pts',(0.594329958849994,0.566643518936724,
-5.54911074079787));
#61066=CARTESIAN_POINT('Ctrl Pts',(0.405242230243789,0.679424716084895,
-5.5402519972246));
#61067=CARTESIAN_POINT('Ctrl Pts',(0.216154501637583,0.792205913233067,
-5.53139325365132));
#61068=CARTESIAN_POINT('Ctrl Pts',(-0.0210816529302957,0.820894963712993,
-5.52253451007805));
#61069=CARTESIAN_POINT('Ctrl Pts',(-0.231602780753465,0.756438604215347,
-5.51367576650478));
#61070=CARTESIAN_POINT('Ctrl Pts',(-0.442123908576634,0.691982244717702,
-5.50481702293151));
#61071=CARTESIAN_POINT('Ctrl Pts',(-0.62263162563433,0.535390358803351,
-5.49595827935824));
#61072=CARTESIAN_POINT('Ctrl Pts',(-0.716163994722249,0.336077881842098,
-5.48709953578496));
#61073=CARTESIAN_POINT('Ctrl Pts',(-0.765317280859578,0.231334857514259,
-5.4824440741312));
#61074=CARTESIAN_POINT('Ctrl Pts',(-0.791100000000061,0.115702837836174,
-5.47778861247744));
#61075=CARTESIAN_POINT('Ctrl Pts',(-0.7911,-4.17166301502903E-13,-5.47313315082368));
#61076=CARTESIAN_POINT('Origin',(0.,0.,-5.925));
#61077=CARTESIAN_POINT('',(-0.790920704737585,-0.000653246164056709,-5.2446668491763));
#61078=CARTESIAN_POINT('',(-0.79181808259713,-0.000281894939852955,-5.27313315082368));
#61079=CARTESIAN_POINT('',(-0.7911,-9.68818082805471E-17,-5.925));
#61080=CARTESIAN_POINT('Ctrl Pts',(-0.790920704737585,-0.000653246164056709,
-5.2446668491763));
#61081=CARTESIAN_POINT('Ctrl Pts',(-0.788945460378493,0.215598739194996,
-5.25337933483792));
#61082=CARTESIAN_POINT('Ctrl Pts',(-0.697988167637598,0.433127810576575,
-5.26209182049953));
#61083=CARTESIAN_POINT('Ctrl Pts',(-0.540326790654243,0.579951476740454,
-5.27080430616114));
#61084=CARTESIAN_POINT('Ctrl Pts',(-0.348670578983709,0.758433158043535,
-5.28139537182407));
#61085=CARTESIAN_POINT('Ctrl Pts',(-0.0584437231446916,0.832431322067987,
-5.291986437487));
#61086=CARTESIAN_POINT('Ctrl Pts',(0.195313604932554,0.768052485885201,
-5.30257750314993));
#61087=CARTESIAN_POINT('Ctrl Pts',(0.449070933009777,0.703673649702421,
-5.31316856881286));
#61088=CARTESIAN_POINT('Ctrl Pts',(0.666358733325236,0.50091781331243,-5.32375963447579));
#61089=CARTESIAN_POINT('Ctrl Pts',(0.750740772904286,0.252196997301994,
-5.33435070013872));
#61090=CARTESIAN_POINT('Ctrl Pts',(0.792931792693813,0.127836589296773,
-5.33964623297019));
#61091=CARTESIAN_POINT('Ctrl Pts',(0.801896372299235,-0.00801506361356036,
-5.34494176580165));
#61092=CARTESIAN_POINT('Ctrl Pts',(0.778678837782813,-0.13784288282515,
-5.35023729863311));
#61093=CARTESIAN_POINT('Ctrl Pts',(0.755461303266393,-0.267670702036732,
-5.35553283146458));
#61094=CARTESIAN_POINT('Ctrl Pts',(0.700061654628132,-0.391474687549571,
-5.36082836429603));
#61095=CARTESIAN_POINT('Ctrl Pts',(0.618214469457432,-0.49398089165876,
-5.3661238971275));
#61096=CARTESIAN_POINT('Ctrl Pts',(0.536367284286727,-0.596487095767956,
-5.37141942995896));
#61097=CARTESIAN_POINT('Ctrl Pts',(0.428072562583579,-0.677695518473499,
-5.37671496279044));
#61098=CARTESIAN_POINT('Ctrl Pts',(0.306507155037109,-0.72897744547975,
-5.3820104956219));
#61099=CARTESIAN_POINT('Ctrl Pts',(0.184941747490638,-0.780259372486002,
-5.38730602845337));
#61100=CARTESIAN_POINT('Ctrl Pts',(0.0501056541008438,-0.80161480379296,
-5.39260156128483));
#61101=CARTESIAN_POINT('Ctrl Pts',(-0.0805206321447689,-0.787954795419253,
-5.39789709411629));
#61102=CARTESIAN_POINT('Ctrl Pts',(-0.341773204635994,-0.760634778671838,
-5.40848815977922));
#61103=CARTESIAN_POINT('Ctrl Pts',(-0.586186548550494,-0.59325300320176,
-5.41907922544215));
#61104=CARTESIAN_POINT('Ctrl Pts',(-0.70564674271158,-0.359769324320271,
-5.42967029110508));
#61105=CARTESIAN_POINT('Ctrl Pts',(-0.762030484629915,-0.249567900451454,
-5.43466914379549));
#61106=CARTESIAN_POINT('Ctrl Pts',(-0.790578115231393,-0.124640797836264,
-5.43966799648589));
#61107=CARTESIAN_POINT('Ctrl Pts',(-0.790531284472335,7.55865616196768E-5,
-5.4446668491763));
#61108=CARTESIAN_POINT('Ctrl Pts',(-0.789707734786939,-0.000536940665675214,
-5.47313315082368));
#61109=CARTESIAN_POINT('Ctrl Pts',(-0.79018851931201,-0.118315462065016,
-5.46840243764117));
#61110=CARTESIAN_POINT('Ctrl Pts',(-0.765626792726158,-0.235892771010167,
-5.46367172445866));
#61111=CARTESIAN_POINT('Ctrl Pts',(-0.715193436764779,-0.341394750524073,
-5.45894101127615));
#61112=CARTESIAN_POINT('Ctrl Pts',(-0.602283825891805,-0.57759135545288,
-5.44834994561322));
#61113=CARTESIAN_POINT('Ctrl Pts',(-0.359701123138071,-0.753264315732189,
-5.43775887995029));
#61114=CARTESIAN_POINT('Ctrl Pts',(-0.0999042190561839,-0.786330656795897,
-5.42716781428736));
#61115=CARTESIAN_POINT('Ctrl Pts',(0.159892685025703,-0.819396997859606,
-5.41657674862443));
#61116=CARTESIAN_POINT('Ctrl Pts',(0.436903790435752,-0.709856719707715,
-5.40598568296151));
#61117=CARTESIAN_POINT('Ctrl Pts',(0.606154956204237,-0.509701287988473,
-5.39539461729858));
#61118=CARTESIAN_POINT('Ctrl Pts',(0.690780539088484,-0.409623572128847,
-5.39009908446711));
#61119=CARTESIAN_POINT('Ctrl Pts',(0.74846613706234,-0.286892067877377,
-5.38480355163564));
#61120=CARTESIAN_POINT('Ctrl Pts',(0.774698971576816,-0.157436828890488,
-5.37950801880418));
#61121=CARTESIAN_POINT('Ctrl Pts',(0.800931806091292,-0.0279815899036063,
-5.37421248597271));
#61122=CARTESIAN_POINT('Ctrl Pts',(0.795711877146396,0.108197383818677,
-5.36891695314125));
#61123=CARTESIAN_POINT('Ctrl Pts',(0.756882813203795,0.233451706564843,
-5.36362142030979));
#61124=CARTESIAN_POINT('Ctrl Pts',(0.679224685318594,0.483960352057175,
-5.35303035464686));
#61125=CARTESIAN_POINT('Ctrl Pts',(0.467130017442567,0.690770393644964,
-5.34243928898393));
#61126=CARTESIAN_POINT('Ctrl Pts',(0.214430568118855,0.762480074022537,
-5.331848223321));
#61127=CARTESIAN_POINT('Ctrl Pts',(0.0880808434569991,0.798334914211325,
-5.32655269048953));
#61128=CARTESIAN_POINT('Ctrl Pts',(-0.0484200765667811,0.800414664097558,
-5.32125715765807));
#61129=CARTESIAN_POINT('Ctrl Pts',(-0.176978016792099,0.770735709357923,
-5.31596162482661));
#61130=CARTESIAN_POINT('Ctrl Pts',(-0.305535957017418,0.741056754618287,
-5.31066609199514));
#61131=CARTESIAN_POINT('Ctrl Pts',(-0.426150917444278,0.679619095252781,
-5.30537055916368));
#61132=CARTESIAN_POINT('Ctrl Pts',(-0.52436170595682,0.592664367831045,
-5.30007502633221));
#61133=CARTESIAN_POINT('Ctrl Pts',(-0.62257249446936,0.505709640409309,
-5.29477949350075));
#61134=CARTESIAN_POINT('Ctrl Pts',(-0.698379111067585,0.39323784493134,
-5.28948396066928));
#61135=CARTESIAN_POINT('Ctrl Pts',(-0.743513036798558,0.26931349180263,
-5.28418842783782));
#61136=CARTESIAN_POINT('Ctrl Pts',(-0.774921147972737,0.18307614822532,
-5.28050333549977));
#61137=CARTESIAN_POINT('Ctrl Pts',(-0.791475742174448,0.0912928041298384,
-5.27681824316172));
#61138=CARTESIAN_POINT('Ctrl Pts',(-0.79181808259713,-0.000281894939852955,
-5.27313315082368));
#61139=CARTESIAN_POINT('Origin',(0.,0.,-5.925));
#61140=CARTESIAN_POINT('',(-0.792204594358573,0.000315518470781081,-5.0446668491763));
#61141=CARTESIAN_POINT('',(-0.791078014336539,0.000374052597120995,-5.07313315082368));
#61142=CARTESIAN_POINT('',(-0.7911,-9.68818082805471E-17,-5.925));
#61143=CARTESIAN_POINT('Ctrl Pts',(-0.792204594358573,0.000315518470781081,
-5.0446668491763));
#61144=CARTESIAN_POINT('Ctrl Pts',(-0.79246329697991,0.0310447806827188,
-5.04590854186408));
#61145=CARTESIAN_POINT('Ctrl Pts',(-0.790845381848934,0.0617570747404931,
-5.04715023455185));
#61146=CARTESIAN_POINT('Ctrl Pts',(-0.787265111314072,0.0922518323957158,
-5.04839192723963));
#61147=CARTESIAN_POINT('Ctrl Pts',(-0.756727055723453,0.352358043764337,
-5.05898299290256));
#61148=CARTESIAN_POINT('Ctrl Pts',(-0.583421702319185,0.596637823128375,
-5.06957405856549));
#61149=CARTESIAN_POINT('Ctrl Pts',(-0.348334401689638,0.711839286595329,
-5.08016512422842));
#61150=CARTESIAN_POINT('Ctrl Pts',(-0.113247101060097,0.827040750062279,
-5.09075618989135));
#61151=CARTESIAN_POINT('Ctrl Pts',(0.183622146794714,0.813163897632151,
-5.10134725555427));
#61152=CARTESIAN_POINT('Ctrl Pts',(0.408947385305092,0.678216093590518,
-5.1119383212172));
#61153=CARTESIAN_POINT('Ctrl Pts',(0.521610004560291,0.610742191569696,
-5.11723385404867));
#61154=CARTESIAN_POINT('Ctrl Pts',(0.616386621479376,0.513000551645993,
-5.12252938688014));
#61155=CARTESIAN_POINT('Ctrl Pts',(0.682734783222974,0.399017052926018,
-5.1278249197116));
#61156=CARTESIAN_POINT('Ctrl Pts',(0.749082944966569,0.285033554206049,
-5.13312045254307));
#61157=CARTESIAN_POINT('Ctrl Pts',(0.787002651534682,0.154808196689791,
-5.13841598537453));
#61158=CARTESIAN_POINT('Ctrl Pts',(0.790977118250049,0.0236949356473377,
-5.14371151820599));
#61159=CARTESIAN_POINT('Ctrl Pts',(0.794951584965415,-0.107418325395108,
-5.14900705103746));
#61160=CARTESIAN_POINT('Ctrl Pts',(0.764980811828053,-0.239419489963747,
-5.15430258386892));
#61161=CARTESIAN_POINT('Ctrl Pts',(0.705522254309981,-0.357201764866207,
-5.15959811670039));
#61162=CARTESIAN_POINT('Ctrl Pts',(0.646063696791902,-0.47498403976868,
-5.16489364953185));
#61163=CARTESIAN_POINT('Ctrl Pts',(0.557117354893093,-0.578547425004965,
-5.17018918236332));
#61164=CARTESIAN_POINT('Ctrl Pts',(0.448712359625208,-0.652697134972368,
-5.17548471519478));
#61165=CARTESIAN_POINT('Ctrl Pts',(0.231902369089455,-0.800996554907163,
-5.18607578085771));
#61166=CARTESIAN_POINT('Ctrl Pts',(-0.062742234922631,-0.831641273766528,
-5.19666684652064));
#61167=CARTESIAN_POINT('Ctrl Pts',(-0.304939923081079,-0.7310150037407,
-5.20725791218357));
#61168=CARTESIAN_POINT('Ctrl Pts',(-0.426038767160313,-0.680701868727781,
-5.21255344501503));
#61169=CARTESIAN_POINT('Ctrl Pts',(-0.534025882276133,-0.597570986493561,
-5.2178489778465));
#61170=CARTESIAN_POINT('Ctrl Pts',(-0.616719234357281,-0.494572782648415,
-5.22314451067796));
#61171=CARTESIAN_POINT('Ctrl Pts',(-0.69941258643842,-0.391574578803282,
-5.22844004350943));
#61172=CARTESIAN_POINT('Ctrl Pts',(-0.756812175484892,-0.268709053347231,
-5.23373557634089));
#61173=CARTESIAN_POINT('Ctrl Pts',(-0.779564306932199,-0.139637836612918,
-5.23903110917236));
#61174=CARTESIAN_POINT('Ctrl Pts',(-0.787635581435542,-0.0938500728090807,
-5.24090968917367));
#61175=CARTESIAN_POINT('Ctrl Pts',(-0.791346605530403,-0.0472813464236894,
-5.24278826917499));
#61176=CARTESIAN_POINT('Ctrl Pts',(-0.790920704737585,-0.000653246164056709,
-5.2446668491763));
#61177=CARTESIAN_POINT('Ctrl Pts',(-0.79181808259713,-0.000281894939852955,
-5.27313315082368));
#61178=CARTESIAN_POINT('Ctrl Pts',(-0.791967690484436,-0.0403014087066727,
-5.27152271033026));
#61179=CARTESIAN_POINT('Ctrl Pts',(-0.789021048451441,-0.0802810750128665,
-5.26991226983684));
#61180=CARTESIAN_POINT('Ctrl Pts',(-0.782864753571529,-0.119740599482619,
-5.26830182934342));
#61181=CARTESIAN_POINT('Ctrl Pts',(-0.742377865928075,-0.379246254236745,
-5.25771076368049));
#61182=CARTESIAN_POINT('Ctrl Pts',(-0.563072263542853,-0.616255575381294,
-5.24711969801757));
#61183=CARTESIAN_POINT('Ctrl Pts',(-0.324111150269872,-0.72319014623882,
-5.23652863235464));
#61184=CARTESIAN_POINT('Ctrl Pts',(-0.0851500369968912,-0.830124717096347,
-5.22593756669171));
#61185=CARTESIAN_POINT('Ctrl Pts',(0.213466587163831,-0.806984537666828,
-5.21534650102878));
#61186=CARTESIAN_POINT('Ctrl Pts',(0.43288697747365,-0.664007244543216,
-5.20475543536585));
#61187=CARTESIAN_POINT('Ctrl Pts',(0.652307367783463,-0.52102995141961,
-5.19416436970292));
#61188=CARTESIAN_POINT('Ctrl Pts',(0.792531524242369,-0.25821554460192,
-5.18357330403999));
#61189=CARTESIAN_POINT('Ctrl Pts',(0.791962104743775,0.00390623942245968,
-5.17298223837706));
#61190=CARTESIAN_POINT('Ctrl Pts',(0.791677394994479,0.134967131434653,
-5.1676867055456));
#61191=CARTESIAN_POINT('Ctrl Pts',(0.756194291255797,0.26585486774854,-5.16239117271413));
#61192=CARTESIAN_POINT('Ctrl Pts',(0.692385554167272,0.381506350855799,
-5.15709563988267));
#61193=CARTESIAN_POINT('Ctrl Pts',(0.628576817078747,0.497157833963058,
-5.1518001070512));
#61194=CARTESIAN_POINT('Ctrl Pts',(0.536442446640378,0.597573063863706,
-5.14650457421974));
#61195=CARTESIAN_POINT('Ctrl Pts',(0.425763601408166,0.667904669918289,
-5.14120904138828));
#61196=CARTESIAN_POINT('Ctrl Pts',(0.204405910943742,0.808567882027454,
-5.13061797572535));
#61197=CARTESIAN_POINT('Ctrl Pts',(-0.0911296786960406,0.828896598752346,
-5.12002691006241));
#61198=CARTESIAN_POINT('Ctrl Pts',(-0.330156313607016,0.719967457783326,
-5.10943584439948));
#61199=CARTESIAN_POINT('Ctrl Pts',(-0.449669631062504,0.665502887298816,
-5.10414031156802));
#61200=CARTESIAN_POINT('Ctrl Pts',(-0.555055709835787,0.578723852390829,
-5.09884477873656));
#61201=CARTESIAN_POINT('Ctrl Pts',(-0.633828647979511,0.47288053158344,
-5.0935492459051));
#61202=CARTESIAN_POINT('Ctrl Pts',(-0.712601586123234,0.36703721077605,
-5.08825371307363));
#61203=CARTESIAN_POINT('Ctrl Pts',(-0.764761383637394,0.242129604069261,
-5.08295818024217));
#61204=CARTESIAN_POINT('Ctrl Pts',(-0.783326391228992,0.112276517467586,
-5.0776626474107));
#61205=CARTESIAN_POINT('Ctrl Pts',(-0.788619540580868,0.075253544124127,
-5.07615281521503));
#61206=CARTESIAN_POINT('Ctrl Pts',(-0.791181763733698,0.0378285518770546,
-5.07464298301935));
#61207=CARTESIAN_POINT('Ctrl Pts',(-0.791078014336539,0.000374052597120995,
-5.07313315082368));
#61208=CARTESIAN_POINT('Origin',(0.,0.,-5.925));
#61209=CARTESIAN_POINT('',(-0.790607229746229,0.000210778082028613,-4.8446668491763));
#61210=CARTESIAN_POINT('',(-0.7911,-3.88467036316342E-13,-4.87313315082368));
#61211=CARTESIAN_POINT('',(-0.7911,-9.68818082805471E-17,-5.925));
#61212=CARTESIAN_POINT('Ctrl Pts',(-0.789880781196105,0.000521509970750122,
-4.8446668491763));
#61213=CARTESIAN_POINT('Ctrl Pts',(-0.790311297832213,0.109477148114268,
-4.84902881455317));
#61214=CARTESIAN_POINT('Ctrl Pts',(-0.769390262863306,0.218221643359569,
-4.85339077993004));
#61215=CARTESIAN_POINT('Ctrl Pts',(-0.72630816890144,0.317062248033498,
-4.8577527453069));
#61216=CARTESIAN_POINT('Ctrl Pts',(-0.621702733822472,0.557052079180901,
-4.86834381096983));
#61217=CARTESIAN_POINT('Ctrl Pts',(-0.386448505408363,0.738654296591801,
-4.87893487663277));
#61218=CARTESIAN_POINT('Ctrl Pts',(-0.127348890008807,0.781663158762513,
-4.88952594229569));
#61219=CARTESIAN_POINT('Ctrl Pts',(0.00220091769097169,0.803167589847869,
-4.89482147512716));
#61220=CARTESIAN_POINT('Ctrl Pts',(0.137712072137115,0.790023682123179,
-4.90011700795862));
#61221=CARTESIAN_POINT('Ctrl Pts',(0.262069525770256,0.746097149445568,
-4.90541254079008));
#61222=CARTESIAN_POINT('Ctrl Pts',(0.386426979403397,0.702170616767958,
-4.91070807362155));
#61223=CARTESIAN_POINT('Ctrl Pts',(0.499630732223539,0.627461459137427,
-4.91600360645302));
#61224=CARTESIAN_POINT('Ctrl Pts',(0.587536521468257,0.530101016327572,
-4.92129913928448));
#61225=CARTESIAN_POINT('Ctrl Pts',(0.675442310712974,0.432740573517717,
-4.92659467211595));
#61226=CARTESIAN_POINT('Ctrl Pts',(0.738050136382271,0.312728845528534,
-4.93189020494741));
#61227=CARTESIAN_POINT('Ctrl Pts',(0.768978010925335,0.184465635996092,
-4.93718573777887));
#61228=CARTESIAN_POINT('Ctrl Pts',(0.7999058854684,0.0562024264636513,-4.94248127061034));
#61229=CARTESIAN_POINT('Ctrl Pts',(0.799153808885237,-0.0803122646120308,
-4.9477768034418));
#61230=CARTESIAN_POINT('Ctrl Pts',(0.76452951145305,-0.207004728928604,
-4.95307233627327));
#61231=CARTESIAN_POINT('Ctrl Pts',(0.695280916588675,-0.460389657561749,
-4.9636634019362));
#61232=CARTESIAN_POINT('Ctrl Pts',(0.49054343832819,-0.674485679158382,
-4.97425446759912));
#61233=CARTESIAN_POINT('Ctrl Pts',(0.240801924961463,-0.754576520518603,
-4.98484553326205));
#61234=CARTESIAN_POINT('Ctrl Pts',(0.115931168278092,-0.794621941198716,
-4.99014106609352));
#61235=CARTESIAN_POINT('Ctrl Pts',(-0.020190597181845,-0.801166066819722,
-4.99543659892498));
#61236=CARTESIAN_POINT('Ctrl Pts',(-0.149894847527861,-0.776193523579221,
-5.00073213175645));
#61237=CARTESIAN_POINT('Ctrl Pts',(-0.27959909787387,-0.751220980338721,
-5.00602766458791));
#61238=CARTESIAN_POINT('Ctrl Pts',(-0.402885833105963,-0.694731768236716,
-5.01132319741938));
#61239=CARTESIAN_POINT('Ctrl Pts',(-0.503781863631195,-0.611083519606513,
-5.01661873025085));
#61240=CARTESIAN_POINT('Ctrl Pts',(-0.681915896808727,-0.463400802861689,
-5.025968103226));
#61241=CARTESIAN_POINT('Ctrl Pts',(-0.790256682995049,-0.231061646345439,
-5.03531747620115));
#61242=CARTESIAN_POINT('Ctrl Pts',(-0.792204594358573,0.000315518470781081,
-5.0446668491763));
#61243=CARTESIAN_POINT('Ctrl Pts',(-0.791078014336539,0.000374052597120995,
-5.07313315082368));
#61244=CARTESIAN_POINT('Ctrl Pts',(-0.790817876713358,-0.0935380537572494,
-5.06934745018789));
#61245=CARTESIAN_POINT('Ctrl Pts',(-0.773797089544038,-0.187635667286825,
-5.0655617495521));
#61246=CARTESIAN_POINT('Ctrl Pts',(-0.741039549927412,-0.276046695672426,
-5.0617760489163));
#61247=CARTESIAN_POINT('Ctrl Pts',(-0.695217483365202,-0.399718255714205,
-5.05648051608484));
#61248=CARTESIAN_POINT('Ctrl Pts',(-0.618603132571746,-0.512262809301205,
-5.05118498325337));
#61249=CARTESIAN_POINT('Ctrl Pts',(-0.519177958415979,-0.5980545803253,
-5.04588945042191));
#61250=CARTESIAN_POINT('Ctrl Pts',(-0.320327610104445,-0.769638122373489,
-5.03529838475898));
#61251=CARTESIAN_POINT('Ctrl Pts',(-0.030233968343667,-0.834210534170057,
-5.02470731909606));
#61252=CARTESIAN_POINT('Ctrl Pts',(0.221124351197595,-0.761023026358905,
-5.01411625343313));
#61253=CARTESIAN_POINT('Ctrl Pts',(0.472482670738857,-0.687835518547754,
-5.0035251877702));
#61254=CARTESIAN_POINT('Ctrl Pts',(0.685105668060603,-0.476888091128884,
-4.99293412210727));
#61255=CARTESIAN_POINT('Ctrl Pts',(0.759789177345915,-0.225869790057779,
-4.98234305644434));
#61256=CARTESIAN_POINT('Ctrl Pts',(0.834472686631226,0.025148511013326,
-4.97175199078141));
#61257=CARTESIAN_POINT('Ctrl Pts',(0.771216707880102,0.316237685736666,
-4.96116092511847));
#61258=CARTESIAN_POINT('Ctrl Pts',(0.601097529576061,0.515655887192186,
-4.95056985945555));
#61259=CARTESIAN_POINT('Ctrl Pts',(0.51603794042404,0.615364987919945,-4.94527432662408));
#61260=CARTESIAN_POINT('Ctrl Pts',(0.404262551383771,0.692156345330761,
-4.93997879379262));
#61261=CARTESIAN_POINT('Ctrl Pts',(0.280760850166947,0.738998103093141,
-4.93468326096116));
#61262=CARTESIAN_POINT('Ctrl Pts',(0.157259148950123,0.785839860855522,
-4.92938772812969));
#61263=CARTESIAN_POINT('Ctrl Pts',(0.0220311355567532,0.802732018969479,
-4.92409219529823));
#61264=CARTESIAN_POINT('Ctrl Pts',(-0.107856599431224,0.784689904575202,
-4.91879666246676));
#61265=CARTESIAN_POINT('Ctrl Pts',(-0.367632069407185,0.748605675786647,
-4.90820559680383));
#61266=CARTESIAN_POINT('Ctrl Pts',(-0.606046425761481,0.572784356965126,
-4.89761453114091));
#61267=CARTESIAN_POINT('Ctrl Pts',(-0.717714788418723,0.335025094830986,
-4.88702346547798));
#61268=CARTESIAN_POINT('Ctrl Pts',(-0.766532938345096,0.231083682697319,
-4.88239336059321));
#61269=CARTESIAN_POINT('Ctrl Pts',(-0.791127605893187,0.115304794406683,
-4.87776325570845));
#61270=CARTESIAN_POINT('Ctrl Pts',(-0.790871083339374,-0.000158561846635865,
-4.87313315082368));
#61271=CARTESIAN_POINT('Origin',(0.,0.,-5.925));
#61272=CARTESIAN_POINT('',(-0.790948977202054,-0.000261541659524338,-4.6446668491763));
#61273=CARTESIAN_POINT('',(-0.7911,-3.71369601737115E-13,-4.67313315082368));
#61274=CARTESIAN_POINT('',(-0.7911,-9.68818082805471E-17,-5.925));
#61275=CARTESIAN_POINT('Ctrl Pts',(-0.7911,1.95454763485259E-13,-4.6446668491763));
#61276=CARTESIAN_POINT('Ctrl Pts',(-0.791099999999946,0.220167589666875,
-4.65352559274958));
#61277=CARTESIAN_POINT('Ctrl Pts',(-0.69421457667226,0.43861041833886,-4.66238433632285));
#61278=CARTESIAN_POINT('Ctrl Pts',(-0.531017389080177,0.586395551223295,
-4.67124307989612));
#61279=CARTESIAN_POINT('Ctrl Pts',(-0.367820201488094,0.734180684107729,
-4.68010182346939));
#61280=CARTESIAN_POINT('Ctrl Pts',(-0.140868175871529,0.808992666571375,
-4.68896056704267));
#61281=CARTESIAN_POINT('Ctrl Pts',(0.0782205473249772,0.787223447298276,
-4.69781931061594));
#61282=CARTESIAN_POINT('Ctrl Pts',(0.297309270521483,0.765454228025177,
-4.70667805418921));
#61283=CARTESIAN_POINT('Ctrl Pts',(0.505102072675782,0.647444880834086,
-4.71553679776249));
#61284=CARTESIAN_POINT('Ctrl Pts',(0.636026795761869,0.470435038100788,
-4.72439554133576));
#61285=CARTESIAN_POINT('Ctrl Pts',(0.766951518847956,0.29342519536749,-4.73325428490903));
#61286=CARTESIAN_POINT('Ctrl Pts',(0.818956872247089,0.0601881960096812,
-4.7421130284823));
#61287=CARTESIAN_POINT('Ctrl Pts',(0.775631781004162,-0.155674501111492,
-4.75097177205558));
#61288=CARTESIAN_POINT('Ctrl Pts',(0.732306689761234,-0.371537198232665,
-4.75983051562885));
#61289=CARTESIAN_POINT('Ctrl Pts',(0.594329958850033,-0.566643518936689,
-4.76868925920212));
#61290=CARTESIAN_POINT('Ctrl Pts',(0.40524223024382,-0.679424716084876,
-4.77754800277539));
#61291=CARTESIAN_POINT('Ctrl Pts',(0.216154501637606,-0.792205913233064,
-4.78640674634867));
#61292=CARTESIAN_POINT('Ctrl Pts',(-0.0210816529302905,-0.820894963712997,
-4.79526548992194));
#61293=CARTESIAN_POINT('Ctrl Pts',(-0.231602780753473,-0.756438604215344,
-4.80412423349521));
#61294=CARTESIAN_POINT('Ctrl Pts',(-0.442123908576656,-0.691982244717692,
-4.81298297706848));
#61295=CARTESIAN_POINT('Ctrl Pts',(-0.62263162563436,-0.535390358803322,
-4.82184172064176));
#61296=CARTESIAN_POINT('Ctrl Pts',(-0.716163994722272,-0.336077881842049,
-4.83070046421503));
#61297=CARTESIAN_POINT('Ctrl Pts',(-0.765317280859552,-0.231334857514295,
-4.83535592586879));
#61298=CARTESIAN_POINT('Ctrl Pts',(-0.791100000000026,-0.115702837836315,
-4.84001138752255));
#61299=CARTESIAN_POINT('Ctrl Pts',(-0.7911,1.78468351208494E-13,-4.8446668491763));
#61300=CARTESIAN_POINT('Ctrl Pts',(-0.7911,-3.88467036316342E-13,-4.87313315082368));
#61301=CARTESIAN_POINT('Ctrl Pts',(-0.791099999999892,-0.220167589667068,
-4.86427440725041));
#61302=CARTESIAN_POINT('Ctrl Pts',(-0.694214576672153,-0.43861041833903,
-4.85541566367713));
#61303=CARTESIAN_POINT('Ctrl Pts',(-0.531017389080034,-0.586395551223424,
-4.84655692010386));
#61304=CARTESIAN_POINT('Ctrl Pts',(-0.367820201487915,-0.734180684107819,
-4.83769817653059));
#61305=CARTESIAN_POINT('Ctrl Pts',(-0.140868175871331,-0.808992666571409,
-4.82883943295732));
#61306=CARTESIAN_POINT('Ctrl Pts',(0.0782205473251693,-0.787223447298257,
-4.81998068938404));
#61307=CARTESIAN_POINT('Ctrl Pts',(0.29730927052167,-0.765454228025104,
-4.81112194581077));
#61308=CARTESIAN_POINT('Ctrl Pts',(0.50510207267594,-0.647444880833963,
-4.8022632022375));
#61309=CARTESIAN_POINT('Ctrl Pts',(0.636026795761984,-0.470435038100633,
-4.79340445866423));
#61310=CARTESIAN_POINT('Ctrl Pts',(0.766951518848027,-0.293425195367303,
-4.78454571509095));
#61311=CARTESIAN_POINT('Ctrl Pts',(0.818956872247104,-0.0601881960094816,
-4.77568697151768));
#61312=CARTESIAN_POINT('Ctrl Pts',(0.775631781004124,0.155674501111681,
-4.76682822794441));
#61313=CARTESIAN_POINT('Ctrl Pts',(0.732306689761144,0.371537198232844,
-4.75796948437114));
#61314=CARTESIAN_POINT('Ctrl Pts',(0.594329958849895,0.566643518936834,
-4.74911074079786));
#61315=CARTESIAN_POINT('Ctrl Pts',(0.405242230243654,0.679424716084975,
-4.74025199722459));
#61316=CARTESIAN_POINT('Ctrl Pts',(0.216154501637413,0.792205913233117,
-4.73139325365132));
#61317=CARTESIAN_POINT('Ctrl Pts',(-0.0210816529304906,0.820894963712992,
-4.72253451007804));
#61318=CARTESIAN_POINT('Ctrl Pts',(-0.231602780753658,0.756438604215288,
-4.71367576650477));
#61319=CARTESIAN_POINT('Ctrl Pts',(-0.442123908576825,0.691982244717585,
-4.7048170229315));
#61320=CARTESIAN_POINT('Ctrl Pts',(-0.62263162563449,0.535390358803171,
-4.69595827935823));
#61321=CARTESIAN_POINT('Ctrl Pts',(-0.716163994722354,0.336077881841874,
-4.68709953578495));
#61322=CARTESIAN_POINT('Ctrl Pts',(-0.765317280859606,0.231334857514115,
-4.6824440741312));
#61323=CARTESIAN_POINT('Ctrl Pts',(-0.791100000000051,0.115702837836137,
-4.67778861247744));
#61324=CARTESIAN_POINT('Ctrl Pts',(-0.7911,-3.48887585488455E-13,-4.67313315082368));
#61325=CARTESIAN_POINT('Origin',(0.,0.,-5.925));
#61326=CARTESIAN_POINT('',(-0.791966503588212,6.66945195454318E-6,-4.4446668491763));
#61327=CARTESIAN_POINT('',(-0.791525477886921,-8.44546748736536E-5,-4.47313315082368));
#61328=CARTESIAN_POINT('',(-0.7911,-9.68818082805471E-17,-5.925));
#61329=CARTESIAN_POINT('Ctrl Pts',(-0.791966503588212,6.66945195454318E-6,
-4.4446668491763));
#61330=CARTESIAN_POINT('Ctrl Pts',(-0.792369950221889,0.131611474342429,
-4.44997382709989));
#61331=CARTESIAN_POINT('Ctrl Pts',(-0.757450744888324,0.263526968080427,
-4.45528080502347));
#61332=CARTESIAN_POINT('Ctrl Pts',(-0.693836616678797,0.379383898055742,
-4.46058778294706));
#61333=CARTESIAN_POINT('Ctrl Pts',(-0.630359679459704,0.494990969588929,
-4.46588331577853));
#61334=CARTESIAN_POINT('Ctrl Pts',(-0.538311520124503,0.59460866003309,
-4.47117884860999));
#61335=CARTESIAN_POINT('Ctrl Pts',(-0.428005770805877,0.665595456510494,
-4.47647438144146));
#61336=CARTESIAN_POINT('Ctrl Pts',(-0.317700021487244,0.736582252987901,
-4.48176991427292));
#61337=CARTESIAN_POINT('Ctrl Pts',(-0.189136682185182,0.778938155498549,
-4.48706544710439));
#61338=CARTESIAN_POINT('Ctrl Pts',(-0.0575587042796079,0.78869623285,-4.49236097993585));
#61339=CARTESIAN_POINT('Ctrl Pts',(0.0740192736259514,0.798454310201449,
-4.49765651276731));
#61340=CARTESIAN_POINT('Ctrl Pts',(0.208611890135023,0.77561456239371,-4.50295204559878));
#61341=CARTESIAN_POINT('Ctrl Pts',(0.328028928417781,0.720939216440974,
-4.50824757843024));
#61342=CARTESIAN_POINT('Ctrl Pts',(0.566863004983317,0.611588524535494,
-4.51883864409317));
#61343=CARTESIAN_POINT('Ctrl Pts',(0.744994768643586,0.374895440050002,
-4.5294297097561));
#61344=CARTESIAN_POINT('Ctrl Pts',(0.783603804359831,0.115483203003332,
-4.54002077541903));
#61345=CARTESIAN_POINT('Ctrl Pts',(0.802908322217952,-0.0142229155199985,
-4.54531630825049));
#61346=CARTESIAN_POINT('Ctrl Pts',(0.78733215809007,-0.149608822183623,
-4.55061184108196));
#61347=CARTESIAN_POINT('Ctrl Pts',(0.741693763534813,-0.273560253866108,
-4.55590737391342));
#61348=CARTESIAN_POINT('Ctrl Pts',(0.696055368979556,-0.397511685548593,
-4.56120290674489));
#61349=CARTESIAN_POINT('Ctrl Pts',(0.620354743996924,-0.510028642249938,
-4.56649843957635));
#61350=CARTESIAN_POINT('Ctrl Pts',(0.521477628194601,-0.596053955066941,
-4.57179397240782));
#61351=CARTESIAN_POINT('Ctrl Pts',(0.323723396589961,-0.76810458070094,
-4.58238503807075));
#61352=CARTESIAN_POINT('Ctrl Pts',(0.0332632017065634,-0.834188630797575,
-4.59297610373368));
#61353=CARTESIAN_POINT('Ctrl Pts',(-0.21846958092695,-0.761949997232314,
-4.6035671693966));
#61354=CARTESIAN_POINT('Ctrl Pts',(-0.470202363560477,-0.68971136366705,
-4.61415823505953));
#61355=CARTESIAN_POINT('Ctrl Pts',(-0.683207733944114,-0.47915004643987,
-4.62474930072247));
#61356=CARTESIAN_POINT('Ctrl Pts',(-0.758836430659324,-0.228515419272388,
-4.63534036638539));
#61357=CARTESIAN_POINT('Ctrl Pts',(-0.781035951175385,-0.154945877689627,
-4.63844919398236));
#61358=CARTESIAN_POINT('Ctrl Pts',(-0.791398872216265,-0.0779235540097163,
-4.64155802157933));
#61359=CARTESIAN_POINT('Ctrl Pts',(-0.790670861719162,-0.000743182749338822,
-4.64466684917631));
#61360=CARTESIAN_POINT('Ctrl Pts',(-0.7911,-3.48887585488455E-13,-4.67313315082368));
#61361=CARTESIAN_POINT('Ctrl Pts',(-0.791099999999903,-0.220167589667021,
-4.66427440725041));
#61362=CARTESIAN_POINT('Ctrl Pts',(-0.694214576672182,-0.43861041833898,
-4.65541566367714));
#61363=CARTESIAN_POINT('Ctrl Pts',(-0.53101738908008,-0.586395551223383,
-4.64655692010386));
#61364=CARTESIAN_POINT('Ctrl Pts',(-0.367820201487978,-0.734180684107785,
-4.63769817653059));
#61365=CARTESIAN_POINT('Ctrl Pts',(-0.14086817587141,-0.808992666571393,
-4.62883943295732));
#61366=CARTESIAN_POINT('Ctrl Pts',(0.0782205473250852,-0.787223447298265,
-4.61998068938405));
#61367=CARTESIAN_POINT('Ctrl Pts',(0.297309270521581,-0.765454228025137,
-4.61112194581077));
#61368=CARTESIAN_POINT('Ctrl Pts',(0.505102072675857,-0.647444880834025,
-4.6022632022375));
#61369=CARTESIAN_POINT('Ctrl Pts',(0.63602679576192,-0.470435038100719,
-4.59340445866423));
#61370=CARTESIAN_POINT('Ctrl Pts',(0.766951518847983,-0.293425195367412,
-4.58454571509096));
#61371=CARTESIAN_POINT('Ctrl Pts',(0.818956872247093,-0.0601881960096083,
-4.57568697151769));
#61372=CARTESIAN_POINT('Ctrl Pts',(0.77563178100415,0.155674501111554,-4.56682822794441));
#61373=CARTESIAN_POINT('Ctrl Pts',(0.732306689761206,0.371537198232717,
-4.55796948437114));
#61374=CARTESIAN_POINT('Ctrl Pts',(0.594329958849998,0.566643518936723,
-4.54911074079787));
#61375=CARTESIAN_POINT('Ctrl Pts',(0.405242230243785,0.679424716084898,
-4.5402519972246));
#61376=CARTESIAN_POINT('Ctrl Pts',(0.216154501637572,0.792205913233072,
-4.53139325365132));
#61377=CARTESIAN_POINT('Ctrl Pts',(-0.0210816529303167,0.820894963712994,
-4.52253451007805));
#61378=CARTESIAN_POINT('Ctrl Pts',(-0.231602780753491,0.756438604215339,
-4.51367576650478));
#61379=CARTESIAN_POINT('Ctrl Pts',(-0.442123908576665,0.691982244717684,
-4.50481702293151));
#61380=CARTESIAN_POINT('Ctrl Pts',(-0.62263162563436,0.535390358803319,
-4.49595827935823));
#61381=CARTESIAN_POINT('Ctrl Pts',(-0.71616399472227,0.336077881842053,
-4.48709953578496));
#61382=CARTESIAN_POINT('Ctrl Pts',(-0.765317280859574,0.231334857514251,
-4.4824440741312));
#61383=CARTESIAN_POINT('Ctrl Pts',(-0.791100000000049,0.115702837836214,
-4.47778861247744));
#61384=CARTESIAN_POINT('Ctrl Pts',(-0.7911,-3.31845662060459E-13,-4.47313315082368));
#61385=CARTESIAN_POINT('Origin',(0.,0.,-5.925));
#61386=CARTESIAN_POINT('',(-0.791036741154233,7.90254580421569E-5,-4.24466684917631));
#61387=CARTESIAN_POINT('',(-0.790970110322915,0.00058332005030696,-4.27313315082368));
#61388=CARTESIAN_POINT('',(-0.7911,-9.68818082805471E-17,-5.925));
#61389=CARTESIAN_POINT('Ctrl Pts',(-0.790748515183379,0.000439088762327566,
-4.24466684917631));
#61390=CARTESIAN_POINT('Ctrl Pts',(-0.790835927644234,0.0782887347139587,
-4.24779856695752));
#61391=CARTESIAN_POINT('Ctrl Pts',(-0.779640960872226,0.156013699302697,
-4.25093028473873));
#61392=CARTESIAN_POINT('Ctrl Pts',(-0.75709689931653,0.230240171594448,
-4.25406200251995));
#61393=CARTESIAN_POINT('Ctrl Pts',(-0.718976344891441,0.355752350036183,
-4.25935753535141));
#61394=CARTESIAN_POINT('Ctrl Pts',(-0.648405744472263,0.471261419145324,
-4.26465306818287));
#61395=CARTESIAN_POINT('Ctrl Pts',(-0.554435133095759,0.563876258889497,
-4.26994860101434));
#61396=CARTESIAN_POINT('Ctrl Pts',(-0.460464521719244,0.65649109863368,
-4.2752441338458));
#61397=CARTESIAN_POINT('Ctrl Pts',(-0.343093899385398,0.726211709012889,
-4.28053966667727));
#61398=CARTESIAN_POINT('Ctrl Pts',(-0.216681111813741,0.761843571518856,
-4.28583519950874));
#61399=CARTESIAN_POINT('Ctrl Pts',(0.0361444633295574,0.833107296530785,
-4.29642626517167));
#61400=CARTESIAN_POINT('Ctrl Pts',(0.325138699424094,0.768016030049762,
-4.30701733083458));
#61401=CARTESIAN_POINT('Ctrl Pts',(0.522497292065463,0.59528805814275,-4.31760839649752));
#61402=CARTESIAN_POINT('Ctrl Pts',(0.621176588386148,0.508924072189243,
-4.32290392932898));
#61403=CARTESIAN_POINT('Ctrl Pts',(0.696946973843541,0.395650909879239,
-4.32819946216045));
#61404=CARTESIAN_POINT('Ctrl Pts',(0.742402068266281,0.271632141683701,
-4.33349499499192));
#61405=CARTESIAN_POINT('Ctrl Pts',(0.787857162689021,0.147613373488162,
-4.33879052782338));
#61406=CARTESIAN_POINT('Ctrl Pts',(0.802996966077109,0.0128489994070881,
-4.34408606065484));
#61407=CARTESIAN_POINT('Ctrl Pts',(0.783322431151289,-0.116727044482598,
-4.34938159348631));
#61408=CARTESIAN_POINT('Ctrl Pts',(0.743973361299652,-0.375879132261963,
-4.35997265914923));
#61409=CARTESIAN_POINT('Ctrl Pts',(0.565366938192395,-0.614277899275778,
-4.37056372481216));
#61410=CARTESIAN_POINT('Ctrl Pts',(0.326734668627864,-0.722178102956162,
-4.38115479047509));
#61411=CARTESIAN_POINT('Ctrl Pts',(0.0881023990633191,-0.830078306636553,
-4.39174585613802));
#61412=CARTESIAN_POINT('Ctrl Pts',(-0.210555716958507,-0.807479946983497,
-4.40233692180096));
#61413=CARTESIAN_POINT('Ctrl Pts',(-0.430448148214726,-0.665406955959684,
-4.41292798746388));
#61414=CARTESIAN_POINT('Ctrl Pts',(-0.650102955683813,-0.523487494195533,
-4.42350760803469));
#61415=CARTESIAN_POINT('Ctrl Pts',(-0.791162220554377,-0.262351478835906,
-4.43408722860549));
#61416=CARTESIAN_POINT('Ctrl Pts',(-0.791966503588212,6.66945195454318E-6,
-4.4446668491763));
#61417=CARTESIAN_POINT('Ctrl Pts',(-0.792015954376217,-0.000181811160338708,
-4.47313315082368));
#61418=CARTESIAN_POINT('Ctrl Pts',(-0.79106198746347,-0.255451043576872,
-4.46282166976077));
#61419=CARTESIAN_POINT('Ctrl Pts',(-0.657614632699196,-0.509262474217293,
-4.45251018869786));
#61420=CARTESIAN_POINT('Ctrl Pts',(-0.446783095806645,-0.654019263464673,
-4.44219870763495));
#61421=CARTESIAN_POINT('Ctrl Pts',(-0.338509093390211,-0.728360119580303,
-4.43690317480349));
#61422=CARTESIAN_POINT('Ctrl Pts',(-0.209825728930858,-0.773938823051294,
-4.43160764197202));
#61423=CARTESIAN_POINT('Ctrl Pts',(-0.0785231522652674,-0.786885548671759,
-4.42631210914056));
#61424=CARTESIAN_POINT('Ctrl Pts',(0.0527794244003236,-0.799832274292223,
-4.42101657630909));
#61425=CARTESIAN_POINT('Ctrl Pts',(0.186701213272174,-0.780147022062139,
-4.41572104347763));
#61426=CARTESIAN_POINT('Ctrl Pts',(0.307544825190331,-0.729124428385988,
-4.41042551064616));
#61427=CARTESIAN_POINT('Ctrl Pts',(0.428388437108489,-0.678101834709837,
-4.4051299778147));
#61428=CARTESIAN_POINT('Ctrl Pts',(0.536153872072984,-0.595741899587628,
-4.39983444498324));
#61429=CARTESIAN_POINT('Ctrl Pts',(0.618512723066843,-0.492730559385846,
-4.39453891215177));
#61430=CARTESIAN_POINT('Ctrl Pts',(0.700871574060708,-0.389719219184058,
-4.38924337932031));
#61431=CARTESIAN_POINT('Ctrl Pts',(0.757823841083915,-0.266056473902705,
-4.38394784648884));
#61432=CARTESIAN_POINT('Ctrl Pts',(0.780093353519537,-0.136635988479275,
-4.37865231365737));
#61433=CARTESIAN_POINT('Ctrl Pts',(0.824632378390776,0.12220498236757,-4.36806124799444));
#61434=CARTESIAN_POINT('Ctrl Pts',(0.730440384911687,0.40407691378272,-4.35747018233152));
#61435=CARTESIAN_POINT('Ctrl Pts',(0.53816407146517,0.581748620561365,-4.34687911666859));
#61436=CARTESIAN_POINT('Ctrl Pts',(0.345887758018658,0.759420327340004,
-4.33628805100566));
#61437=CARTESIAN_POINT('Ctrl Pts',(0.0555271246047256,0.832891809482146,
-4.32569698534273));
#61438=CARTESIAN_POINT('Ctrl Pts',(-0.198071796498553,0.767505256988222,
-4.3151059196798));
#61439=CARTESIAN_POINT('Ctrl Pts',(-0.451670717601839,0.702118704494297,
-4.30451485401687));
#61440=CARTESIAN_POINT('Ctrl Pts',(-0.668507926394469,0.497874117364298,
-4.29392378835394));
#61441=CARTESIAN_POINT('Ctrl Pts',(-0.751708375512725,0.249306542718858,
-4.28333272269101));
#61442=CARTESIAN_POINT('Ctrl Pts',(-0.778416703304708,0.169513412604227,
-4.2799328654019));
#61443=CARTESIAN_POINT('Ctrl Pts',(-0.791353951428056,0.0851528611175555,
-4.27653300811279));
#61444=CARTESIAN_POINT('Ctrl Pts',(-0.790970110322915,0.00058332005030696,
-4.27313315082368));
#61445=CARTESIAN_POINT('Origin',(0.,0.,-5.925));
#61446=CARTESIAN_POINT('',(-0.791030670713791,-9.38883850568749E-5,-4.04466684917631));
#61447=CARTESIAN_POINT('',(-0.789613844031706,-0.000310489881695122,-4.07313315082369));
#61448=CARTESIAN_POINT('',(-0.7911,-9.68818082805471E-17,-5.925));
#61449=CARTESIAN_POINT('Ctrl Pts',(-0.7911,2.69173572320369E-13,-4.04466684917631));
#61450=CARTESIAN_POINT('Ctrl Pts',(-0.791099999999925,0.220167589666956,
-4.05352559274958));
#61451=CARTESIAN_POINT('Ctrl Pts',(-0.694214576672213,0.43861041833894,
-4.06238433632285));
#61452=CARTESIAN_POINT('Ctrl Pts',(-0.531017389080106,0.586395551223359,
-4.07124307989613));
#61453=CARTESIAN_POINT('Ctrl Pts',(-0.367820201487999,0.734180684107779,
-4.0801018234694));
#61454=CARTESIAN_POINT('Ctrl Pts',(-0.140868175871415,0.808992666571397,
-4.08896056704267));
#61455=CARTESIAN_POINT('Ctrl Pts',(0.0782205473250954,0.787223447298264,
-4.09781931061594));
#61456=CARTESIAN_POINT('Ctrl Pts',(0.297309270521605,0.765454228025131,
-4.10667805418922));
#61457=CARTESIAN_POINT('Ctrl Pts',(0.505102072675893,0.647444880834002,
-4.11553679776249));
#61458=CARTESIAN_POINT('Ctrl Pts',(0.636026795761953,0.470435038100674,
-4.12439554133576));
#61459=CARTESIAN_POINT('Ctrl Pts',(0.766951518848012,0.293425195367347,
-4.13325428490904));
#61460=CARTESIAN_POINT('Ctrl Pts',(0.818956872247103,0.0601881960095193,
-4.14211302848231));
#61461=CARTESIAN_POINT('Ctrl Pts',(0.77563178100413,-0.155674501111652,
-4.15097177205558));
#61462=CARTESIAN_POINT('Ctrl Pts',(0.732306689761156,-0.371537198232824,
-4.15983051562886));
#61463=CARTESIAN_POINT('Ctrl Pts',(0.594329958849906,-0.566643518936825,
-4.16868925920213));
#61464=CARTESIAN_POINT('Ctrl Pts',(0.40524223024366,-0.679424716084972,
-4.1775480027754));
#61465=CARTESIAN_POINT('Ctrl Pts',(0.216154501637414,-0.792205913233119,
-4.18640674634868));
#61466=CARTESIAN_POINT('Ctrl Pts',(-0.0210816529304995,-0.820894963712993,
-4.19526548992195));
#61467=CARTESIAN_POINT('Ctrl Pts',(-0.231602780753673,-0.756438604215284,
-4.20412423349522));
#61468=CARTESIAN_POINT('Ctrl Pts',(-0.442123908576845,-0.691982244717574,
-4.21298297706849));
#61469=CARTESIAN_POINT('Ctrl Pts',(-0.622631625634513,-0.535390358803147,
-4.22184172064177));
#61470=CARTESIAN_POINT('Ctrl Pts',(-0.71616399472237,-0.33607788184184,
-4.23070046421504));
#61471=CARTESIAN_POINT('Ctrl Pts',(-0.765317280859594,-0.231334857514126,
-4.23535592586879));
#61472=CARTESIAN_POINT('Ctrl Pts',(-0.791100000000033,-0.115702837836204,
-4.24001138752255));
#61473=CARTESIAN_POINT('Ctrl Pts',(-0.7911,2.29594121492482E-13,-4.2446668491763));
#61474=CARTESIAN_POINT('Ctrl Pts',(-0.790970110322915,0.00058332005030696,
-4.27313315082368));
#61475=CARTESIAN_POINT('Ctrl Pts',(-0.790756090105803,-0.0465705446553784,
-4.27123747528133));
#61476=CARTESIAN_POINT('Ctrl Pts',(-0.786400677548894,-0.0937893821146618,
-4.26934179973898));
#61477=CARTESIAN_POINT('Ctrl Pts',(-0.777981876000496,-0.140317682337169,
-4.26744612419662));
#61478=CARTESIAN_POINT('Ctrl Pts',(-0.754464117288605,-0.270293585868894,
-4.26215059136516));
#61479=CARTESIAN_POINT('Ctrl Pts',(-0.699237565224288,-0.394880858730763,
-4.25685505853369));
#61480=CARTESIAN_POINT('Ctrl Pts',(-0.616827522050246,-0.496885399689367,
-4.25155952570223));
#61481=CARTESIAN_POINT('Ctrl Pts',(-0.452007435702166,-0.700894481606568,
-4.24096846003929));
#61482=CARTESIAN_POINT('Ctrl Pts',(-0.178453384915186,-0.814572635910709,
-4.23037739437637));
#61483=CARTESIAN_POINT('Ctrl Pts',(0.0828469823253125,-0.787713595922422,
-4.21978632871344));
#61484=CARTESIAN_POINT('Ctrl Pts',(0.213497165945573,-0.774284075928278,
-4.21449079588198));
#61485=CARTESIAN_POINT('Ctrl Pts',(0.341083928679213,-0.725720257361019,
-4.20919526305051));
#61486=CARTESIAN_POINT('Ctrl Pts',(0.449542640975874,-0.650589091588972,
-4.20389973021904));
#61487=CARTESIAN_POINT('Ctrl Pts',(0.558001353272529,-0.57545792581693,
-4.19860419738758));
#61488=CARTESIAN_POINT('Ctrl Pts',(0.647332015132223,-0.473759412840084,
-4.19330866455611));
#61489=CARTESIAN_POINT('Ctrl Pts',(0.706408306709897,-0.35664205554281,
-4.18801313172465));
#61490=CARTESIAN_POINT('Ctrl Pts',(0.765484598287572,-0.239524698245536,
-4.18271759889319));
#61491=CARTESIAN_POINT('Ctrl Pts',(0.794306519583243,-0.106988496627837,
-4.17742206606172));
#61492=CARTESIAN_POINT('Ctrl Pts',(0.790395038786528,0.0248410025943516,
-4.17212653323026));
#61493=CARTESIAN_POINT('Ctrl Pts',(0.786483557989814,0.156670501816548,
-4.16683100039879));
#61494=CARTESIAN_POINT('Ctrl Pts',(0.749838675100704,0.287793298643213,
-4.16153546756733));
#61495=CARTESIAN_POINT('Ctrl Pts',(0.683031628147731,0.400852626912842,
-4.15623993473586));
#61496=CARTESIAN_POINT('Ctrl Pts',(0.549417534241792,0.626971283452087,
-4.14564886907293));
#61497=CARTESIAN_POINT('Ctrl Pts',(0.295154784080413,0.780836065763196,
-4.13505780341001));
#61498=CARTESIAN_POINT('Ctrl Pts',(0.0335873339007514,0.791785271612486,
-4.12446673774708));
#61499=CARTESIAN_POINT('Ctrl Pts',(-0.227980116278903,0.802734477461776,
-4.11387567208415));
#61500=CARTESIAN_POINT('Ctrl Pts',(-0.49685226647684,0.670768106849258,
-4.10328460642122));
#61501=CARTESIAN_POINT('Ctrl Pts',(-0.647814891993137,0.456763200996579,
-4.09269354075829));
#61502=CARTESIAN_POINT('Ctrl Pts',(-0.740751332153453,0.325016326173946,
-4.08617341078009));
#61503=CARTESIAN_POINT('Ctrl Pts',(-0.789000682338518,0.162177277791855,
-4.07965328080189));
#61504=CARTESIAN_POINT('Ctrl Pts',(-0.789613844031706,-0.000310489881695122,
-4.07313315082369));
#61505=CARTESIAN_POINT('Origin',(0.,0.,-5.925));
#61506=CARTESIAN_POINT('',(-0.791171331530249,-5.58023572299298E-6,-3.84466684917632));
#61507=CARTESIAN_POINT('',(-0.791632884276151,-0.000316525830029703,-3.87313315082368));
#61508=CARTESIAN_POINT('',(-0.7911,-9.68818082805471E-17,-5.925));
#61509=CARTESIAN_POINT('Ctrl Pts',(-0.791516496870447,-3.25823843516648E-5,
-3.84466684917631));
#61510=CARTESIAN_POINT('Ctrl Pts',(-0.789509283147655,0.232306133060974,
-3.8540391123357));
#61511=CARTESIAN_POINT('Ctrl Pts',(-0.681965996973624,0.464363987367173,
-3.86341137549509));
#61512=CARTESIAN_POINT('Ctrl Pts',(-0.502861014580263,0.611965760805632,
-3.87278363865449));
#61513=CARTESIAN_POINT('Ctrl Pts',(-0.401662798267677,0.695363977856574,
-3.87807917148596));
#61514=CARTESIAN_POINT('Ctrl Pts',(-0.277618538052244,0.75179962368152,
-3.88337470431743));
#61515=CARTESIAN_POINT('Ctrl Pts',(-0.147877509951437,0.776580384385472,
-3.88867023714889));
#61516=CARTESIAN_POINT('Ctrl Pts',(-0.0181364818506448,0.801361145089422,
-3.89396576998036));
#61517=CARTESIAN_POINT('Ctrl Pts',(0.117301314135521,0.794487020672385,
-3.89926130281182));
#61518=CARTESIAN_POINT('Ctrl Pts',(0.24198381704612,0.754097517796073,-3.90455683564328));
#61519=CARTESIAN_POINT('Ctrl Pts',(0.491348822867332,0.673318512043445,
-3.91514790130621));
#61520=CARTESIAN_POINT('Ctrl Pts',(0.697692656386272,0.458477992453703,
-3.92573896696914));
#61521=CARTESIAN_POINT('Ctrl Pts',(0.765542558291149,0.205526999486113,
-3.93633003263207));
#61522=CARTESIAN_POINT('Ctrl Pts',(0.833392460196026,-0.0474239934814776,
-3.946921098295));
#61523=CARTESIAN_POINT('Ctrl Pts',(0.76274843048684,-0.338485459826917,
-3.95751216395792));
#61524=CARTESIAN_POINT('Ctrl Pts',(0.586955159983497,-0.532480671489366,
-3.96810322962085));
#61525=CARTESIAN_POINT('Ctrl Pts',(0.411161889480155,-0.726475883151815,
-3.97869429528378));
#61526=CARTESIAN_POINT('Ctrl Pts',(0.130219378182655,-0.823404840131275,
-3.98928536094672));
#61527=CARTESIAN_POINT('Ctrl Pts',(-0.129042526256825,-0.781385346657027,
-3.99987642660965));
#61528=CARTESIAN_POINT('Ctrl Pts',(-0.258673478476572,-0.760375599919902,
-4.00517195944111));
#61529=CARTESIAN_POINT('Ctrl Pts',(-0.382884278981814,-0.704628740569346,
-4.01046749227258));
#61530=CARTESIAN_POINT('Ctrl Pts',(-0.486691749451913,-0.623275648299921,
-4.01576302510404));
#61531=CARTESIAN_POINT('Ctrl Pts',(-0.590499219922001,-0.541922556030505,
-4.0210585579355));
#61532=CARTESIAN_POINT('Ctrl Pts',(-0.67390336035695,-0.434963230842226,
-4.02635409076697));
#61533=CARTESIAN_POINT('Ctrl Pts',(-0.726098836681858,-0.314621567823627,
-4.03164962359843));
#61534=CARTESIAN_POINT('Ctrl Pts',(-0.768866977999572,-0.216015527362374,
-4.03598869879106));
#61535=CARTESIAN_POINT('Ctrl Pts',(-0.790681926886867,-0.108424715917689,
-4.04032777398368));
#61536=CARTESIAN_POINT('Ctrl Pts',(-0.790747516019094,-0.000477347360857,
-4.04466684917631));
#61537=CARTESIAN_POINT('Ctrl Pts',(-0.789613844031706,-0.000310489881695122,
-4.07313315082369));
#61538=CARTESIAN_POINT('Ctrl Pts',(-0.789996680236759,-0.101762033633977,
-4.06906221513896));
#61539=CARTESIAN_POINT('Ctrl Pts',(-0.771809470400046,-0.203076637401392,
-4.06499127945423));
#61540=CARTESIAN_POINT('Ctrl Pts',(-0.734334414868844,-0.296601080911116,
-4.0609203437695));
#61541=CARTESIAN_POINT('Ctrl Pts',(-0.68558631313122,-0.418259048392196,
-4.05562481093804));
#61542=CARTESIAN_POINT('Ctrl Pts',(-0.604200885316122,-0.526735139340602,
-4.05032927810657));
#61543=CARTESIAN_POINT('Ctrl Pts',(-0.50213564953078,-0.610577301274807,
-4.04503374527511));
#61544=CARTESIAN_POINT('Ctrl Pts',(-0.400070413745437,-0.694419463209012,
-4.03973821244364));
#61545=CARTESIAN_POINT('Ctrl Pts',(-0.277325369989872,-0.753627696129009,
-4.03444267961218));
#61546=CARTESIAN_POINT('Ctrl Pts',(-0.148480305168211,-0.778026279350681,
-4.02914714678072));
#61547=CARTESIAN_POINT('Ctrl Pts',(0.109209824475106,-0.826823445794026,
-4.01855608111779));
#61548=CARTESIAN_POINT('Ctrl Pts',(0.391300038382742,-0.736382013444024,
-4.00796501545485));
#61549=CARTESIAN_POINT('Ctrl Pts',(0.573073513987495,-0.546756873982823,
-3.99737394979192));
#61550=CARTESIAN_POINT('Ctrl Pts',(0.663960251789879,-0.451944304252214,
-3.99207841696046));
#61551=CARTESIAN_POINT('Ctrl Pts',(0.729767805016544,-0.332335807743801,
-3.986782884129));
#61552=CARTESIAN_POINT('Ctrl Pts',(0.76379769728162,-0.204860512977544,
-3.98148735129753));
#61553=CARTESIAN_POINT('Ctrl Pts',(0.797827589546692,-0.0773852182113021,
-3.97619181846607));
#61554=CARTESIAN_POINT('Ctrl Pts',(0.800079820850182,0.0579568748127813,
-3.9708962856346));
#61555=CARTESIAN_POINT('Ctrl Pts',(0.769291022740716,0.185465829470251,
-3.96560075280314));
#61556=CARTESIAN_POINT('Ctrl Pts',(0.73850222463125,0.312974784127721,-3.96030521997167));
#61557=CARTESIAN_POINT('Ctrl Pts',(0.674672397108829,0.432650600418577,
-3.95500968714021));
#61558=CARTESIAN_POINT('Ctrl Pts',(0.586350956631833,0.530597727478346,
-3.94971415430875));
#61559=CARTESIAN_POINT('Ctrl Pts',(0.498029516154827,0.628544854538127,
-3.94441862147728));
#61560=CARTESIAN_POINT('Ctrl Pts',(0.385216462723241,0.704763292366816,
-3.93912308864582));
#61561=CARTESIAN_POINT('Ctrl Pts',(0.261107514977984,0.747688370362337,
-3.93382755581435));
#61562=CARTESIAN_POINT('Ctrl Pts',(0.0128896194874833,0.833538526353374,
-3.92323649015142));
#61563=CARTESIAN_POINT('Ctrl Pts',(-0.280511853257697,0.786215243011755,
-3.91264542448849));
#61564=CARTESIAN_POINT('Ctrl Pts',(-0.486964156575668,0.625234304522367,
-3.90205435882556));
#61565=CARTESIAN_POINT('Ctrl Pts',(-0.67488512684609,0.478703150983351,
-3.89241395615827));
#61566=CARTESIAN_POINT('Ctrl Pts',(-0.79076563914733,0.23800261569534,-3.88277355349098));
#61567=CARTESIAN_POINT('Ctrl Pts',(-0.792351145598852,-0.000743163040590685,
-3.87313315082368));
#61568=CARTESIAN_POINT('Origin',(0.,0.,-5.925));
#61569=CARTESIAN_POINT('',(-0.7911,2.80775402927702E-13,-3.64466684917631));
#61570=CARTESIAN_POINT('',(-0.7911,-2.86048962294672E-13,-3.67313315082368));
#61571=CARTESIAN_POINT('',(-0.7911,-9.68818082805471E-17,-5.925));
#61572=CARTESIAN_POINT('Ctrl Pts',(-0.7911,2.80775402927702E-13,-3.64466684917631));
#61573=CARTESIAN_POINT('Ctrl Pts',(-0.791099999999922,0.22016758966696,
-3.65352559274958));
#61574=CARTESIAN_POINT('Ctrl Pts',(-0.694214576672213,0.438610418338935,
-3.66238433632285));
#61575=CARTESIAN_POINT('Ctrl Pts',(-0.531017389080114,0.586395551223352,
-3.67124307989613));
#61576=CARTESIAN_POINT('Ctrl Pts',(-0.367820201488015,0.734180684107769,
-3.6801018234694));
#61577=CARTESIAN_POINT('Ctrl Pts',(-0.140868175871441,0.80899266657139,
-3.68896056704267));
#61578=CARTESIAN_POINT('Ctrl Pts',(0.0782205473250622,0.787223447298267,
-3.69781931061594));
#61579=CARTESIAN_POINT('Ctrl Pts',(0.297309270521566,0.765454228025144,
-3.70667805418922));
#61580=CARTESIAN_POINT('Ctrl Pts',(0.505102072675852,0.647444880834032,
-3.71553679776249));
#61581=CARTESIAN_POINT('Ctrl Pts',(0.63602679576192,0.470435038100719,-3.72439554133576));
#61582=CARTESIAN_POINT('Ctrl Pts',(0.766951518847987,0.293425195367407,
-3.73325428490903));
#61583=CARTESIAN_POINT('Ctrl Pts',(0.818956872247096,0.060188196009593,
-3.74211302848231));
#61584=CARTESIAN_POINT('Ctrl Pts',(0.775631781004145,-0.155674501111576,
-3.75097177205558));
#61585=CARTESIAN_POINT('Ctrl Pts',(0.732306689761194,-0.371537198232744,
-3.75983051562885));
#61586=CARTESIAN_POINT('Ctrl Pts',(0.594329958849972,-0.566643518936753,
-3.76868925920212));
#61587=CARTESIAN_POINT('Ctrl Pts',(0.405242230243747,-0.67942471608492,
-3.7775480027754));
#61588=CARTESIAN_POINT('Ctrl Pts',(0.216154501637521,-0.792205913233088,
-3.78640674634867));
#61589=CARTESIAN_POINT('Ctrl Pts',(-0.0210816529303789,-0.820894963712994,
-3.79526548992194));
#61590=CARTESIAN_POINT('Ctrl Pts',(-0.231602780753555,-0.756438604215319,
-3.80412423349522));
#61591=CARTESIAN_POINT('Ctrl Pts',(-0.44212390857673,-0.691982244717645,
-3.81298297706849));
#61592=CARTESIAN_POINT('Ctrl Pts',(-0.622631625634417,-0.535390358803255,
-3.82184172064176));
#61593=CARTESIAN_POINT('Ctrl Pts',(-0.716163994722308,-0.336077881841972,
-3.83070046421503));
#61594=CARTESIAN_POINT('Ctrl Pts',(-0.76531728085958,-0.231334857514206,
-3.83535592586879));
#61595=CARTESIAN_POINT('Ctrl Pts',(-0.791100000000042,-0.115702837836215,
-3.84001138752255));
#61596=CARTESIAN_POINT('Ctrl Pts',(-0.7911,2.86215495748365E-13,-3.84466684917631));
#61597=CARTESIAN_POINT('Ctrl Pts',(-0.7911,-3.0320190802513E-13,-3.87313315082368));
#61598=CARTESIAN_POINT('Ctrl Pts',(-0.791099999999916,-0.22016758966699,
-3.86427440725041));
#61599=CARTESIAN_POINT('Ctrl Pts',(-0.694214576672194,-0.43861041833897,
-3.85541566367714));
#61600=CARTESIAN_POINT('Ctrl Pts',(-0.531017389080081,-0.586395551223382,
-3.84655692010386));
#61601=CARTESIAN_POINT('Ctrl Pts',(-0.367820201487968,-0.734180684107795,
-3.83769817653059));
#61602=CARTESIAN_POINT('Ctrl Pts',(-0.14086817587138,-0.808992666571403,
-3.82883943295732));
#61603=CARTESIAN_POINT('Ctrl Pts',(0.0782205473251291,-0.787223447298261,
-3.81998068938405));
#61604=CARTESIAN_POINT('Ctrl Pts',(0.297309270521638,-0.765454228025119,
-3.81112194581077));
#61605=CARTESIAN_POINT('Ctrl Pts',(0.505102072675921,-0.64744488083398,
-3.8022632022375));
#61606=CARTESIAN_POINT('Ctrl Pts',(0.636026795761973,-0.470435038100647,
-3.79340445866423));
#61607=CARTESIAN_POINT('Ctrl Pts',(0.766951518848025,-0.293425195367314,
-3.78454571509095));
#61608=CARTESIAN_POINT('Ctrl Pts',(0.818956872247106,-0.0601881960094841,
-3.77568697151768));
#61609=CARTESIAN_POINT('Ctrl Pts',(0.775631781004123,0.155674501111686,
-3.76682822794441));
#61610=CARTESIAN_POINT('Ctrl Pts',(0.732306689761141,0.371537198232848,
-3.75796948437113));
#61611=CARTESIAN_POINT('Ctrl Pts',(0.594329958849892,0.566643518936837,
-3.74911074079786));
#61612=CARTESIAN_POINT('Ctrl Pts',(0.40524223024365,0.679424716084978,-3.74025199722459));
#61613=CARTESIAN_POINT('Ctrl Pts',(0.216154501637408,0.792205913233119,
-3.73139325365132));
#61614=CARTESIAN_POINT('Ctrl Pts',(-0.0210816529304954,0.820894963712992,
-3.72253451007804));
#61615=CARTESIAN_POINT('Ctrl Pts',(-0.231602780753662,0.756438604215287,
-3.71367576650477));
#61616=CARTESIAN_POINT('Ctrl Pts',(-0.442123908576829,0.691982244717582,
-3.7048170229315));
#61617=CARTESIAN_POINT('Ctrl Pts',(-0.622631625634493,0.535390358803167,
-3.69595827935823));
#61618=CARTESIAN_POINT('Ctrl Pts',(-0.716163994722355,0.33607788184187,
-3.68709953578495));
#61619=CARTESIAN_POINT('Ctrl Pts',(-0.765317280859597,0.231334857514131,
-3.6824440741312));
#61620=CARTESIAN_POINT('Ctrl Pts',(-0.791100000000042,0.115702837836177,
-3.67778861247744));
#61621=CARTESIAN_POINT('Ctrl Pts',(-0.7911,-2.86048962294672E-13,-3.67313315082368));
#61622=CARTESIAN_POINT('Origin',(0.,0.,-5.925));
#61623=CARTESIAN_POINT('',(-0.790808073136235,0.000138710378817367,-3.44466684917631));
#61624=CARTESIAN_POINT('',(-0.790458003125287,-0.000155518975336373,-3.47313315082369));
#61625=CARTESIAN_POINT('',(-0.7911,-9.68818082805471E-17,-5.925));
#61626=CARTESIAN_POINT('Ctrl Pts',(-0.7911,2.97872837506929E-13,-3.44466684917631));
#61627=CARTESIAN_POINT('Ctrl Pts',(-0.791099999999917,0.220167589666978,
-3.45352559274958));
#61628=CARTESIAN_POINT('Ctrl Pts',(-0.694214576672203,0.43861041833895,
-3.46238433632285));
#61629=CARTESIAN_POINT('Ctrl Pts',(-0.531017389080101,0.586395551223364,
-3.47124307989613));
#61630=CARTESIAN_POINT('Ctrl Pts',(-0.367820201487999,0.734180684107777,
-3.4801018234694));
#61631=CARTESIAN_POINT('Ctrl Pts',(-0.140868175871424,0.808992666571393,
-3.48896056704267));
#61632=CARTESIAN_POINT('Ctrl Pts',(0.078220547325079,0.787223447298266,
-3.49781931061594));
#61633=CARTESIAN_POINT('Ctrl Pts',(0.297309270521582,0.765454228025138,
-3.50667805418922));
#61634=CARTESIAN_POINT('Ctrl Pts',(0.505102072675866,0.647444880834021,
-3.51553679776249));
#61635=CARTESIAN_POINT('Ctrl Pts',(0.63602679576193,0.470435038100706,-3.52439554133576));
#61636=CARTESIAN_POINT('Ctrl Pts',(0.766951518847993,0.29342519536739,-3.53325428490903));
#61637=CARTESIAN_POINT('Ctrl Pts',(0.818956872247097,0.0601881960095753,
-3.54211302848231));
#61638=CARTESIAN_POINT('Ctrl Pts',(0.775631781004142,-0.155674501111592,
-3.55097177205558));
#61639=CARTESIAN_POINT('Ctrl Pts',(0.732306689761186,-0.37153719823276,
-3.55983051562885));
#61640=CARTESIAN_POINT('Ctrl Pts',(0.59432995884996,-0.566643518936766,
-3.56868925920213));
#61641=CARTESIAN_POINT('Ctrl Pts',(0.405242230243732,-0.679424716084929,
-3.5775480027754));
#61642=CARTESIAN_POINT('Ctrl Pts',(0.216154501637504,-0.792205913233092,
-3.58640674634867));
#61643=CARTESIAN_POINT('Ctrl Pts',(-0.0210816529303965,-0.820894963712994,
-3.59526548992194));
#61644=CARTESIAN_POINT('Ctrl Pts',(-0.231602780753571,-0.756438604215315,
-3.60412423349522));
#61645=CARTESIAN_POINT('Ctrl Pts',(-0.442123908576745,-0.691982244717635,
-3.61298297706849));
#61646=CARTESIAN_POINT('Ctrl Pts',(-0.622631625634429,-0.535390358803242,
-3.62184172064176));
#61647=CARTESIAN_POINT('Ctrl Pts',(-0.716163994722315,-0.336077881841956,
-3.63070046421503));
#61648=CARTESIAN_POINT('Ctrl Pts',(-0.765317280859582,-0.231334857514196,
-3.63535592586879));
#61649=CARTESIAN_POINT('Ctrl Pts',(-0.791100000000041,-0.115702837836213,
-3.64001138752255));
#61650=CARTESIAN_POINT('Ctrl Pts',(-0.7911,2.80775402927702E-13,-3.64466684917631));
#61651=CARTESIAN_POINT('Ctrl Pts',(-0.7911,-2.86048962294672E-13,-3.67313315082368));
#61652=CARTESIAN_POINT('Ctrl Pts',(-0.791099999999921,-0.220167589666966,
-3.66427440725041));
#61653=CARTESIAN_POINT('Ctrl Pts',(-0.69421457667221,-0.43861041833894,
-3.65541566367714));
#61654=CARTESIAN_POINT('Ctrl Pts',(-0.53101738908011,-0.586395551223356,
-3.64655692010387));
#61655=CARTESIAN_POINT('Ctrl Pts',(-0.36782020148801,-0.734180684107771,
-3.63769817653059));
#61656=CARTESIAN_POINT('Ctrl Pts',(-0.140868175871436,-0.808992666571391,
-3.62883943295732));
#61657=CARTESIAN_POINT('Ctrl Pts',(0.0782205473250674,-0.787223447298267,
-3.61998068938405));
#61658=CARTESIAN_POINT('Ctrl Pts',(0.297309270521571,-0.765454228025143,
-3.61112194581078));
#61659=CARTESIAN_POINT('Ctrl Pts',(0.505102072675857,-0.647444880834028,
-3.6022632022375));
#61660=CARTESIAN_POINT('Ctrl Pts',(0.636026795761923,-0.470435038100715,
-3.59340445866423));
#61661=CARTESIAN_POINT('Ctrl Pts',(0.766951518847989,-0.293425195367402,
-3.58454571509096));
#61662=CARTESIAN_POINT('Ctrl Pts',(0.818956872247096,-0.0601881960095875,
-3.57568697151768));
#61663=CARTESIAN_POINT('Ctrl Pts',(0.775631781004144,0.155674501111581,
-3.56682822794441));
#61664=CARTESIAN_POINT('Ctrl Pts',(0.732306689761192,0.371537198232749,
-3.55796948437114));
#61665=CARTESIAN_POINT('Ctrl Pts',(0.594329958849968,0.566643518936757,
-3.54911074079787));
#61666=CARTESIAN_POINT('Ctrl Pts',(0.405242230243742,0.679424716084923,
-3.54025199722459));
#61667=CARTESIAN_POINT('Ctrl Pts',(0.216154501637516,0.792205913233089,
-3.53139325365132));
#61668=CARTESIAN_POINT('Ctrl Pts',(-0.0210816529303844,0.820894963712995,
-3.52253451007805));
#61669=CARTESIAN_POINT('Ctrl Pts',(-0.23160278075356,0.756438604215318,
-3.51367576650478));
#61670=CARTESIAN_POINT('Ctrl Pts',(-0.442123908576735,0.691982244717642,
-3.5048170229315));
#61671=CARTESIAN_POINT('Ctrl Pts',(-0.622631625634421,0.535390358803251,
-3.49595827935823));
#61672=CARTESIAN_POINT('Ctrl Pts',(-0.71616399472231,0.336077881841967,
-3.48709953578496));
#61673=CARTESIAN_POINT('Ctrl Pts',(-0.765317280859573,0.231334857514221,
-3.4824440741312));
#61674=CARTESIAN_POINT('Ctrl Pts',(-0.791100000000033,0.115702837836254,
-3.47778861247744));
#61675=CARTESIAN_POINT('Ctrl Pts',(-0.7911,-2.24043006369357E-13,-3.47313315082369));
#61676=CARTESIAN_POINT('Origin',(0.,0.,-5.925));
#61677=CARTESIAN_POINT('',(-0.790501282281534,-0.000660443323588278,-3.24466684917631));
#61678=CARTESIAN_POINT('',(-0.791626275438383,-0.000301773140805729,-3.27313315082369));
#61679=CARTESIAN_POINT('',(-0.7911,-9.68818082805471E-17,-5.925));
#61680=CARTESIAN_POINT('Ctrl Pts',(-0.790501282281534,-0.000660443323588278,
-3.24466684917631));
#61681=CARTESIAN_POINT('Ctrl Pts',(-0.788726547930076,0.201687602482837,
-3.25280886474005));
#61682=CARTESIAN_POINT('Ctrl Pts',(-0.710464001792085,0.405146793643893,
-3.26095088030379));
#61683=CARTESIAN_POINT('Ctrl Pts',(-0.570712392114347,0.550076468829417,
-3.26909289586753));
#61684=CARTESIAN_POINT('Ctrl Pts',(-0.388924668545188,0.738599776649255,
-3.27968396153046));
#61685=CARTESIAN_POINT('Ctrl Pts',(-0.103093830595221,0.828087698747892,
-3.29027502719339));
#61686=CARTESIAN_POINT('Ctrl Pts',(0.153756508941375,0.777438718677672,
-3.30086609285632));
#61687=CARTESIAN_POINT('Ctrl Pts',(0.410606848477986,0.726789738607448,
-3.31145715851925));
#61688=CARTESIAN_POINT('Ctrl Pts',(0.638476689601239,0.536003856368347,
-3.32204822418218));
#61689=CARTESIAN_POINT('Ctrl Pts',(0.7361029627146,0.292177106967427,-3.33263928984511));
#61690=CARTESIAN_POINT('Ctrl Pts',(0.784916099271274,0.17026373226698,-3.33793482267657));
#61691=CARTESIAN_POINT('Ctrl Pts',(0.801168343825486,0.0350901407761204,
-3.34323035550804));
#61692=CARTESIAN_POINT('Ctrl Pts',(0.784961259371031,-0.0957977767742774,
-3.3485258883395));
#61693=CARTESIAN_POINT('Ctrl Pts',(0.768754174916574,-0.22668569432469,
-3.35382142117096));
#61694=CARTESIAN_POINT('Ctrl Pts',(0.720087761453432,-0.353287937934607,
-3.35911695400243));
#61695=CARTESIAN_POINT('Ctrl Pts',(0.643867493490231,-0.460044456979054,
-3.36441248683389));
#61696=CARTESIAN_POINT('Ctrl Pts',(0.56764722552703,-0.5668009760235,-3.36970801966536));
#61697=CARTESIAN_POINT('Ctrl Pts',(0.463873103063763,-0.653711770502485,
-3.37500355249682));
#61698=CARTESIAN_POINT('Ctrl Pts',(0.345239232099723,-0.711452475411619,
-3.38029908532829));
#61699=CARTESIAN_POINT('Ctrl Pts',(0.226605361135696,-0.769193180320747,
-3.38559461815975));
#61700=CARTESIAN_POINT('Ctrl Pts',(0.09311174167089,-0.797763795660035,
-3.39089015099122));
#61701=CARTESIAN_POINT('Ctrl Pts',(-0.0380598711096725,-0.791143335870662,
-3.39618568382268));
#61702=CARTESIAN_POINT('Ctrl Pts',(-0.300403096670812,-0.777902416291914,
-3.40677674948561));
#61703=CARTESIAN_POINT('Ctrl Pts',(-0.553458295495004,-0.623897196198503,
-3.41736781514854));
#61704=CARTESIAN_POINT('Ctrl Pts',(-0.685293196148034,-0.397170653115661,
-3.42795888081147));
#61705=CARTESIAN_POINT('Ctrl Pts',(-0.751210646474553,-0.283807381574233,
-3.43325441364294));
#61706=CARTESIAN_POINT('Ctrl Pts',(-0.786823022258281,-0.152263779285441,
-3.4385499464744));
#61707=CARTESIAN_POINT('Ctrl Pts',(-0.790275839006138,-0.0202225034273728,
-3.44384547930586));
#61708=CARTESIAN_POINT('Ctrl Pts',(-0.790454356745215,-0.0133956974447719,
-3.44411926926268));
#61709=CARTESIAN_POINT('Ctrl Pts',(-0.790546908669895,-0.00656756112944958,
-3.44439305921949));
#61710=CARTESIAN_POINT('Ctrl Pts',(-0.790553609093959,0.000259620127130655,
-3.44466684917631));
#61711=CARTESIAN_POINT('Ctrl Pts',(-0.789563719361682,-0.000372152575058701,
-3.47313315082369));
#61712=CARTESIAN_POINT('Ctrl Pts',(-0.789761280241986,-0.132415731864222,
-3.4678319675433));
#61713=CARTESIAN_POINT('Ctrl Pts',(-0.758600248492401,-0.264319284924409,
-3.46253078426292));
#61714=CARTESIAN_POINT('Ctrl Pts',(-0.695813536878054,-0.379335665655462,
-3.45722960098254));
#61715=CARTESIAN_POINT('Ctrl Pts',(-0.570373960410714,-0.609123238770098,
-3.44663853531961));
#61716=CARTESIAN_POINT('Ctrl Pts',(-0.318701195330903,-0.771506044022968,
-3.43604746965668));
#61717=CARTESIAN_POINT('Ctrl Pts',(-0.0575027298276114,-0.790563211979342,
-3.42545640399375));
#61718=CARTESIAN_POINT('Ctrl Pts',(0.20369573567568,-0.809620379935717,
-3.41486533833082));
#61719=CARTESIAN_POINT('Ctrl Pts',(0.474419901602451,-0.685351910595596,
-3.40427427266789));
#61720=CARTESIAN_POINT('Ctrl Pts',(0.632670215342768,-0.476390210517119,
-3.39368320700496));
#61721=CARTESIAN_POINT('Ctrl Pts',(0.711795372212922,-0.371909360477886,
-3.3883876741735));
#61722=CARTESIAN_POINT('Ctrl Pts',(0.762802066036466,-0.246255202754067,
-3.38309214134204));
#61723=CARTESIAN_POINT('Ctrl Pts',(0.782040115544297,-0.115577286008921,
-3.37779660851057));
#61724=CARTESIAN_POINT('Ctrl Pts',(0.80127816505213,0.0151006307362397,
-3.37250107567911));
#61725=CARTESIAN_POINT('Ctrl Pts',(0.788747570244242,0.150802306502729,
-3.36720554284764));
#61726=CARTESIAN_POINT('Ctrl Pts',(0.743243492909288,0.273788974633951,
-3.36191001001617));
#61727=CARTESIAN_POINT('Ctrl Pts',(0.652235338239384,0.519762310896381,
-3.35131894435324));
#61728=CARTESIAN_POINT('Ctrl Pts',(0.42933325346123,0.71487561661775,-3.34072787869032));
#61729=CARTESIAN_POINT('Ctrl Pts',(0.17314530709567,0.772901697703007,-3.33013681302739));
#61730=CARTESIAN_POINT('Ctrl Pts',(0.0450513339128974,0.801914738245634,
-3.32484128019593));
#61731=CARTESIAN_POINT('Ctrl Pts',(-0.0913641046667258,0.796655972629236,
-3.31954574736446));
#61732=CARTESIAN_POINT('Ctrl Pts',(-0.218141339923086,0.760111247099192,
-3.314250214533));
#61733=CARTESIAN_POINT('Ctrl Pts',(-0.344918575179461,0.723566521569144,
-3.30895468170153));
#61734=CARTESIAN_POINT('Ctrl Pts',(-0.462057607112571,0.655735836125442,
-3.30365914887007));
#61735=CARTESIAN_POINT('Ctrl Pts',(-0.555453563471992,0.563628947443981,
-3.2983636160386));
#61736=CARTESIAN_POINT('Ctrl Pts',(-0.648849519831414,0.47152205876252,
-3.29306808320714));
#61737=CARTESIAN_POINT('Ctrl Pts',(-0.718502400617147,0.355138966843301,
-3.28777255037567));
#61738=CARTESIAN_POINT('Ctrl Pts',(-0.756911456836638,0.228968205779075,
-3.28247701754421));
#61739=CARTESIAN_POINT('Ctrl Pts',(-0.779502139310456,0.15475957163837,
-3.27936239530403));
#61740=CARTESIAN_POINT('Ctrl Pts',(-0.791284565813894,0.0771650641309663,
-3.27624777306386));
#61741=CARTESIAN_POINT('Ctrl Pts',(-0.791626275438383,-0.000301773140805729,
-3.27313315082369));
#61742=CARTESIAN_POINT('Origin',(0.,0.,-5.925));
#61743=CARTESIAN_POINT('',(-0.792512397087544,4.98421984640521E-5,-3.04466684917631));
#61744=CARTESIAN_POINT('',(-0.791208548896392,0.000277519652998023,-3.07313315082369));
#61745=CARTESIAN_POINT('',(-0.7911,-9.68818082805471E-17,-5.925));
#61746=CARTESIAN_POINT('Ctrl Pts',(-0.792512397087544,4.98421984640521E-5,
-3.04466684917631));
#61747=CARTESIAN_POINT('Ctrl Pts',(-0.792602493697506,0.0166490096803601,
-3.04533807176621));
#61748=CARTESIAN_POINT('Ctrl Pts',(-0.792131796472667,0.033246426247799,
-3.04600929435612));
#61749=CARTESIAN_POINT('Ctrl Pts',(-0.79108507893974,0.0498111829976684,
-3.04668051694602));
#61750=CARTESIAN_POINT('Ctrl Pts',(-0.77456916560708,0.31118264019715,-3.05727158260895));
#61751=CARTESIAN_POINT('Ctrl Pts',(-0.61464174908658,0.564422798090375,
-3.06786264827188));
#61752=CARTESIAN_POINT('Ctrl Pts',(-0.386085039148666,0.692091300253508,
-3.07845371393481));
#61753=CARTESIAN_POINT('Ctrl Pts',(-0.157528329210766,0.819759802416634,
-3.08904477959774));
#61754=CARTESIAN_POINT('Ctrl Pts',(0.139657674144527,0.821856648849676,
-3.09963584526066));
#61755=CARTESIAN_POINT('Ctrl Pts',(0.371909359946098,0.699212744118375,
-3.11022691092359));
#61756=CARTESIAN_POINT('Ctrl Pts',(0.48803520284691,0.637890791752711,-3.11552244375506));
#61757=CARTESIAN_POINT('Ctrl Pts',(0.587927466359278,0.545383651595948,
-3.12081797658652));
#61758=CARTESIAN_POINT('Ctrl Pts',(0.660305185987155,0.43513038747796,-3.12611350941799));
#61759=CARTESIAN_POINT('Ctrl Pts',(0.732682905615016,0.324877123359996,
-3.13140904224946));
#61760=CARTESIAN_POINT('Ctrl Pts',(0.777546081358393,0.196877735280824,
-3.13670457508092));
#61761=CARTESIAN_POINT('Ctrl Pts',(0.788560784364571,0.0661675217374577,
-3.14200010791238));
#61762=CARTESIAN_POINT('Ctrl Pts',(0.799575487370749,-0.0645426918059086,
-3.14729564074385));
#61763=CARTESIAN_POINT('Ctrl Pts',(0.776741717639716,-0.1979637308135,-3.15259117357531));
#61764=CARTESIAN_POINT('Ctrl Pts',(0.72369865590798,-0.318771089635041,
-3.15788670640678));
#61765=CARTESIAN_POINT('Ctrl Pts',(0.670655594176238,-0.439578448456596,
-3.16318223923824));
#61766=CARTESIAN_POINT('Ctrl Pts',(0.587403240443787,-0.547772127092131,
-3.16847777206971));
#61767=CARTESIAN_POINT('Ctrl Pts',(0.483139671131421,-0.627640334794113,
-3.17377330490117));
#61768=CARTESIAN_POINT('Ctrl Pts',(0.274612532506713,-0.787376750198057,
-3.1843643705641));
#61769=CARTESIAN_POINT('Ctrl Pts',(-0.0179594684376078,-0.833811281867799,
-3.19495543622703));
#61770=CARTESIAN_POINT('Ctrl Pts',(-0.265214795997095,-0.746346035272733,
-3.20554650188996));
#61771=CARTESIAN_POINT('Ctrl Pts',(-0.388842459776839,-0.7026134119752,
-3.21084203472142));
#61772=CARTESIAN_POINT('Ctrl Pts',(-0.501140955210369,-0.625405844111466,
-3.21613756755288));
#61773=CARTESIAN_POINT('Ctrl Pts',(-0.589249900279902,-0.527000385561387,
-3.22143310038435));
#61774=CARTESIAN_POINT('Ctrl Pts',(-0.677358845349455,-0.428594927011285,
-3.22672863321581));
#61775=CARTESIAN_POINT('Ctrl Pts',(-0.741278240054995,-0.308991577774832,
-3.23202416604728));
#61776=CARTESIAN_POINT('Ctrl Pts',(-0.770933734993954,-0.181329562693679,
-3.23731969887875));
#61777=CARTESIAN_POINT('Ctrl Pts',(-0.784648651912265,-0.122289107153613,
-3.23976874897794));
#61778=CARTESIAN_POINT('Ctrl Pts',(-0.791035107512577,-0.06152504101114,
-3.24221779907712));
#61779=CARTESIAN_POINT('Ctrl Pts',(-0.790501282281534,-0.000660443323588278,
-3.24466684917631));
#61780=CARTESIAN_POINT('Ctrl Pts',(-0.791626275438383,-0.000301773140805729,
-3.27313315082369));
#61781=CARTESIAN_POINT('Ctrl Pts',(-0.791865546233275,-0.0545453483971053,
-3.2709522402324));
#61782=CARTESIAN_POINT('Ctrl Pts',(-0.786495393900723,-0.1087263264945,
-3.26877132964111));
#61783=CARTESIAN_POINT('Ctrl Pts',(-0.775298682791673,-0.161638442254814,
-3.26659041904982));
#61784=CARTESIAN_POINT('Ctrl Pts',(-0.72092455895627,-0.418593355775735,
-3.25599935338689));
#61785=CARTESIAN_POINT('Ctrl Pts',(-0.529141260837061,-0.645624375501621,
-3.24540828772396));
#61786=CARTESIAN_POINT('Ctrl Pts',(-0.284778825431726,-0.739562739682541,
-3.23481722206103));
#61787=CARTESIAN_POINT('Ctrl Pts',(-0.0404163900263632,-0.833501103863472,
-3.2242261563981));
#61788=CARTESIAN_POINT('Ctrl Pts',(0.256525182665126,-0.794346812499395,
-3.21363509073517));
#61789=CARTESIAN_POINT('Ctrl Pts',(0.467944958166465,-0.639784551391566,
-3.20304402507224));
#61790=CARTESIAN_POINT('Ctrl Pts',(0.679364733667791,-0.485222290283745,
-3.19245295940931));
#61791=CARTESIAN_POINT('Ctrl Pts',(0.805262711978977,-0.215252059432152,
-3.18186189374638));
#61792=CARTESIAN_POINT('Ctrl Pts',(0.790607784950011,0.0464603533655111,
-3.17127082808345));
#61793=CARTESIAN_POINT('Ctrl Pts',(0.783280321435528,0.177316559764335,
-3.16597529525199));
#61794=CARTESIAN_POINT('Ctrl Pts',(0.74081463158602,0.306108311649677,-3.16067976242052));
#61795=CARTESIAN_POINT('Ctrl Pts',(0.670883030216598,0.418163617653569,
-3.15538422958906));
#61796=CARTESIAN_POINT('Ctrl Pts',(0.600951428847175,0.53021892365746,-3.15008869675759));
#61797=CARTESIAN_POINT('Ctrl Pts',(0.503553915957842,0.625537783779891,
-3.14479316392613));
#61798=CARTESIAN_POINT('Ctrl Pts',(0.389255408503693,0.689819918046538,
-3.13949763109466));
#61799=CARTESIAN_POINT('Ctrl Pts',(0.160658393595382,0.818384186579839,
-3.12890656543173));
#61800=CARTESIAN_POINT('Ctrl Pts',(-0.135542599572178,0.822801551689975,
-3.11831549976881));
#61801=CARTESIAN_POINT('Ctrl Pts',(-0.368370023734614,0.701184609995972,
-3.10772443410588));
#61802=CARTESIAN_POINT('Ctrl Pts',(-0.484783735815838,0.640376139148968,
-3.10242890127441));
#61803=CARTESIAN_POINT('Ctrl Pts',(-0.585354055645775,0.548059091600927,
-3.09713336844295));
#61804=CARTESIAN_POINT('Ctrl Pts',(-0.65832518346277,0.438135487000128,
-3.09183783561148));
#61805=CARTESIAN_POINT('Ctrl Pts',(-0.731296311279756,0.328211882399341,
-3.08654230278002));
#61806=CARTESIAN_POINT('Ctrl Pts',(-0.776668247083802,0.200681720745806,
-3.08124676994855));
#61807=CARTESIAN_POINT('Ctrl Pts',(-0.7882281697482,0.0700185974291656,
-3.07595123711709));
#61808=CARTESIAN_POINT('Ctrl Pts',(-0.7902787572056,0.0468405737004255,
-3.07501187501929));
#61809=CARTESIAN_POINT('Ctrl Pts',(-0.791265403124425,0.0235639670201663,
-3.07407251292149));
#61810=CARTESIAN_POINT('Ctrl Pts',(-0.791208548896392,0.000277519652998023,
-3.07313315082369));
#61811=CARTESIAN_POINT('Origin',(0.,0.,-5.925));
#61812=CARTESIAN_POINT('',(-0.79070696665834,0.000316758284698436,-2.84466684917631));
#61813=CARTESIAN_POINT('',(-0.7911,-2.17936779733918E-13,-2.87313315082369));
#61814=CARTESIAN_POINT('',(-0.7911,-9.68818082805471E-17,-5.925));
#61815=CARTESIAN_POINT('Ctrl Pts',(-0.790135803578584,0.000777077086083156,
-2.84466684917631));
#61816=CARTESIAN_POINT('Ctrl Pts',(-0.790729188995581,0.0953959190884639,
-2.8484583444553));
#61817=CARTESIAN_POINT('Ctrl Pts',(-0.775074050339769,0.189770316634575,
-2.8522498397343));
#61818=CARTESIAN_POINT('Ctrl Pts',(-0.742297451277547,0.277572547576085,
-2.85604133501329));
#61819=CARTESIAN_POINT('Ctrl Pts',(-0.650740140155824,0.522837047417337,
-2.86663240067622));
#61820=CARTESIAN_POINT('Ctrl Pts',(-0.425585096270472,0.716819323845514,
-2.87722346633915));
#61821=CARTESIAN_POINT('Ctrl Pts',(-0.169171165385708,0.77368995751212,
-2.88781453200208));
#61822=CARTESIAN_POINT('Ctrl Pts',(-0.040964199943333,0.802125274345422,
-2.89311006483355));
#61823=CARTESIAN_POINT('Ctrl Pts',(0.0950574872488943,0.796282680488336,
-2.89840559766501));
#61824=CARTESIAN_POINT('Ctrl Pts',(0.221595838120345,0.75910254727276,-2.90370113049647));
#61825=CARTESIAN_POINT('Ctrl Pts',(0.348134188991795,0.721922414057184,
-2.90899666332794));
#61826=CARTESIAN_POINT('Ctrl Pts',(0.465189203542468,0.65340474148312,-2.9142921961594));
#61827=CARTESIAN_POINT('Ctrl Pts',(0.558200082457864,0.560909011796547,
-2.91958772899087));
#61828=CARTESIAN_POINT('Ctrl Pts',(0.651210961373282,0.468413282109953,
-2.92488326182233));
#61829=CARTESIAN_POINT('Ctrl Pts',(0.72017770465341,0.351939495310839,-2.9301787946538));
#61830=CARTESIAN_POINT('Ctrl Pts',(0.757953706571736,0.225523681338111,
-2.93547432748526));
#61831=CARTESIAN_POINT('Ctrl Pts',(0.795729708490053,0.0991078673654118,
-2.94076986031673));
#61832=CARTESIAN_POINT('Ctrl Pts',(0.802314969046581,-0.0372499737808963,
-2.94606539314819));
#61833=CARTESIAN_POINT('Ctrl Pts',(0.774549111808285,-0.165620062427354,
-2.95136092597966));
#61834=CARTESIAN_POINT('Ctrl Pts',(0.71901739733169,-0.422360239720285,
-2.96195199164259));
#61835=CARTESIAN_POINT('Ctrl Pts',(0.526081211675783,-0.647149407013813,
-2.97254305730551));
#61836=CARTESIAN_POINT('Ctrl Pts',(0.281004632411375,-0.740545534688081,
-2.98313412296844));
#61837=CARTESIAN_POINT('Ctrl Pts',(0.158466342779164,-0.787243598525218,
-2.98842965579991));
#61838=CARTESIAN_POINT('Ctrl Pts',(0.0228929547448268,-0.801093402457536,
-2.99372518863137));
#61839=CARTESIAN_POINT('Ctrl Pts',(-0.107965886047362,-0.78312720474501,
-2.99902072146284));
#61840=CARTESIAN_POINT('Ctrl Pts',(-0.238824726839536,-0.765161007032487,
-3.0043162542943));
#61841=CARTESIAN_POINT('Ctrl Pts',(-0.364969020389562,-0.715378807675126,
-3.00961178712577));
#61842=CARTESIAN_POINT('Ctrl Pts',(-0.470214481065443,-0.637273548685935,
-3.01490731995723));
#61843=CARTESIAN_POINT('Ctrl Pts',(-0.667365265940161,-0.49096307587624,
-3.02482716303026));
#61844=CARTESIAN_POINT('Ctrl Pts',(-0.791180880172482,-0.245265406483679,
-3.03474700610328));
#61845=CARTESIAN_POINT('Ctrl Pts',(-0.792512397087544,4.98421984640521E-5,
-3.04466684917631));
#61846=CARTESIAN_POINT('Ctrl Pts',(-0.791208548896392,0.000277519652998023,
-3.07313315082369));
#61847=CARTESIAN_POINT('Ctrl Pts',(-0.790944894737022,-0.107710380592565,
-3.06877698009002));
#61848=CARTESIAN_POINT('Ctrl Pts',(-0.768240549118296,-0.215909906892349,
-3.06442080935636));
#61849=CARTESIAN_POINT('Ctrl Pts',(-0.725134083974273,-0.315471001848098,
-3.0600646386227));
#61850=CARTESIAN_POINT('Ctrl Pts',(-0.672732166011195,-0.436501392828995,
-3.05476910579123));
#61851=CARTESIAN_POINT('Ctrl Pts',(-0.590180420560288,-0.544766089811032,
-3.04947357295977));
#61852=CARTESIAN_POINT('Ctrl Pts',(-0.486288498717086,-0.625090817056648,
-3.0441780401283));
#61853=CARTESIAN_POINT('Ctrl Pts',(-0.278504655030694,-0.78574027154787,
-3.03358697446538));
#61854=CARTESIAN_POINT('Ctrl Pts',(0.0146398942248702,-0.83462984709342,
-3.02299590880244));
#61855=CARTESIAN_POINT('Ctrl Pts',(0.261701926009823,-0.748040190941482,
-3.01240484313951));
#61856=CARTESIAN_POINT('Ctrl Pts',(0.508763957794776,-0.661450534789544,
-3.00181377747658));
#61857=CARTESIAN_POINT('Ctrl Pts',(0.709743472109117,-0.439381646940117,
-2.99122271181366));
#61858=CARTESIAN_POINT('Ctrl Pts',(0.770829429168333,-0.184712607043331,
-2.98063164615073));
#61859=CARTESIAN_POINT('Ctrl Pts',(0.831915386227548,0.0699564328534561,
-2.9700405804878));
#61860=CARTESIAN_POINT('Ctrl Pts',(0.753107786031637,0.357225624797604,
-2.95944951482487));
#61861=CARTESIAN_POINT('Ctrl Pts',(0.572517770699919,0.547213519835908,
-2.94885844916194));
#61862=CARTESIAN_POINT('Ctrl Pts',(0.482222763034065,0.642207467355056,
-2.94356291633048));
#61863=CARTESIAN_POINT('Ctrl Pts',(0.366482151584262,0.712881090647745,
-2.93826738349901));
#61864=CARTESIAN_POINT('Ctrl Pts',(0.240641653404015,0.75301822422084,-2.93297185066755));
#61865=CARTESIAN_POINT('Ctrl Pts',(0.114801155223755,0.793155357793939,
-2.92767631783608));
#61866=CARTESIAN_POINT('Ctrl Pts',(-0.0211392296869517,0.802756001647437,
-2.92238078500462));
#61867=CARTESIAN_POINT('Ctrl Pts',(-0.149869697759458,0.777759838302671,
-2.91708525217315));
#61868=CARTESIAN_POINT('Ctrl Pts',(-0.407330633904457,0.727767511613141,
-2.90649418651022));
#61869=CARTESIAN_POINT('Ctrl Pts',(-0.635951902696659,0.539387956130569,
-2.8959031208473));
#61870=CARTESIAN_POINT('Ctrl Pts',(-0.734681805311768,0.295971242902559,
-2.88531205518437));
#61871=CARTESIAN_POINT('Ctrl Pts',(-0.772525716389172,0.202667793733097,
-2.88125242039747));
#61872=CARTESIAN_POINT('Ctrl Pts',(-0.791285386387945,0.101278030456626,
-2.87719278561058));
#61873=CARTESIAN_POINT('Ctrl Pts',(-0.790978541062857,4.5186565332119E-6,
-2.87313315082368));
#61874=CARTESIAN_POINT('Origin',(0.,0.,-5.925));
#61875=CARTESIAN_POINT('',(-0.790765068286233,-0.000289649196591382,-2.64466684917631));
#61876=CARTESIAN_POINT('',(-0.79086137551975,-3.96814382399647E-5,-2.67313315082369));
#61877=CARTESIAN_POINT('',(-0.7911,-9.68818082805471E-17,-5.925));
#61878=CARTESIAN_POINT('Ctrl Pts',(-0.7911,3.66040531218914E-13,-2.64466684917631));
#61879=CARTESIAN_POINT('Ctrl Pts',(-0.791099999999898,0.220167589667046,
-2.65352559274958));
#61880=CARTESIAN_POINT('Ctrl Pts',(-0.694214576672165,0.43861041833901,
-2.66238433632286));
#61881=CARTESIAN_POINT('Ctrl Pts',(-0.531017389080051,0.586395551223409,
-2.67124307989613));
#61882=CARTESIAN_POINT('Ctrl Pts',(-0.367820201487936,0.734180684107808,
-2.6801018234694));
#61883=CARTESIAN_POINT('Ctrl Pts',(-0.140868175871354,0.808992666571405,
-2.68896056704267));
#61884=CARTESIAN_POINT('Ctrl Pts',(0.078220547325147,0.787223447298259,
-2.69781931061595));
#61885=CARTESIAN_POINT('Ctrl Pts',(0.297309270521648,0.765454228025112,
-2.70667805418922));
#61886=CARTESIAN_POINT('Ctrl Pts',(0.505102072675922,0.647444880833977,
-2.71553679776249));
#61887=CARTESIAN_POINT('Ctrl Pts',(0.63602679576197,0.470435038100651,-2.72439554133577));
#61888=CARTESIAN_POINT('Ctrl Pts',(0.766951518848019,0.293425195367324,
-2.73325428490904));
#61889=CARTESIAN_POINT('Ctrl Pts',(0.818956872247102,0.0601881960095046,
-2.74211302848231));
#61890=CARTESIAN_POINT('Ctrl Pts',(0.775631781004128,-0.155674501111659,
-2.75097177205558));
#61891=CARTESIAN_POINT('Ctrl Pts',(0.732306689761154,-0.371537198232823,
-2.75983051562886));
#61892=CARTESIAN_POINT('Ctrl Pts',(0.594329958849911,-0.566643518936817,
-2.76868925920213));
#61893=CARTESIAN_POINT('Ctrl Pts',(0.405242230243673,-0.679424716084964,
-2.7775480027754));
#61894=CARTESIAN_POINT('Ctrl Pts',(0.216154501637436,-0.792205913233111,
-2.78640674634867));
#61895=CARTESIAN_POINT('Ctrl Pts',(-0.0210816529304674,-0.820894963712992,
-2.79526548992195));
#61896=CARTESIAN_POINT('Ctrl Pts',(-0.231602780753636,-0.756438604215295,
-2.80412423349522));
#61897=CARTESIAN_POINT('Ctrl Pts',(-0.442123908576805,-0.691982244717597,
-2.81298297706849));
#61898=CARTESIAN_POINT('Ctrl Pts',(-0.622631625634475,-0.535390358803188,
-2.82184172064176));
#61899=CARTESIAN_POINT('Ctrl Pts',(-0.716163994722344,-0.336077881841895,
-2.83070046421504));
#61900=CARTESIAN_POINT('Ctrl Pts',(-0.765317280859602,-0.23133485751413,
-2.83535592586879));
#61901=CARTESIAN_POINT('Ctrl Pts',(-0.791100000000051,-0.115702837836144,
-2.84001138752255));
#61902=CARTESIAN_POINT('Ctrl Pts',(-0.7911,3.48998607790918E-13,-2.84466684917631));
#61903=CARTESIAN_POINT('Ctrl Pts',(-0.7911,-2.17936779733918E-13,-2.87313315082369));
#61904=CARTESIAN_POINT('Ctrl Pts',(-0.79109999999994,-0.220167589666883,
-2.86427440725041));
#61905=CARTESIAN_POINT('Ctrl Pts',(-0.694214576672262,-0.438610418338851,
-2.85541566367714));
#61906=CARTESIAN_POINT('Ctrl Pts',(-0.531017389080194,-0.58639555122328,
-2.84655692010387));
#61907=CARTESIAN_POINT('Ctrl Pts',(-0.367820201488126,-0.734180684107709,
-2.8376981765306));
#61908=CARTESIAN_POINT('Ctrl Pts',(-0.140868175871583,-0.808992666571361,
-2.82883943295733));
#61909=CARTESIAN_POINT('Ctrl Pts',(0.07822054732491,-0.787223447298283,
-2.81998068938405));
#61910=CARTESIAN_POINT('Ctrl Pts',(0.297309270521403,-0.765454228025204,
-2.81112194581078));
#61911=CARTESIAN_POINT('Ctrl Pts',(0.505102072675699,-0.647444880834146,
-2.80226320223751));
#61912=CARTESIAN_POINT('Ctrl Pts',(0.636026795761802,-0.470435038100878,
-2.79340445866424));
#61913=CARTESIAN_POINT('Ctrl Pts',(0.766951518847905,-0.293425195367611,
-2.78454571509097));
#61914=CARTESIAN_POINT('Ctrl Pts',(0.818956872247075,-0.0601881960098297,
-2.77568697151769));
#61915=CARTESIAN_POINT('Ctrl Pts',(0.775631781004193,0.155674501111338,
-2.76682822794442));
#61916=CARTESIAN_POINT('Ctrl Pts',(0.732306689761311,0.371537198232505,
-2.75796948437115));
#61917=CARTESIAN_POINT('Ctrl Pts',(0.594329958850165,0.566643518936544,
-2.74911074079788));
#61918=CARTESIAN_POINT('Ctrl Pts',(0.405242230243994,0.679424716084773,
-2.74025199722461));
#61919=CARTESIAN_POINT('Ctrl Pts',(0.216154501637822,0.792205913233001,
-2.73139325365133));
#61920=CARTESIAN_POINT('Ctrl Pts',(-0.021081652930048,0.820894963712999,
-2.72253451007806));
#61921=CARTESIAN_POINT('Ctrl Pts',(-0.231602780753237,0.756438604215417,
-2.71367576650479));
#61922=CARTESIAN_POINT('Ctrl Pts',(-0.442123908576425,0.691982244717835,
-2.70481702293152));
#61923=CARTESIAN_POINT('Ctrl Pts',(-0.622631625634168,0.535390358803539,
-2.69595827935824));
#61924=CARTESIAN_POINT('Ctrl Pts',(-0.716163994722147,0.336077881842314,
-2.68709953578497));
#61925=CARTESIAN_POINT('Ctrl Pts',(-0.765317280859505,0.231334857514496,
-2.68244407413121));
#61926=CARTESIAN_POINT('Ctrl Pts',(-0.791100000000023,0.115702837836428,
-2.67778861247745));
#61927=CARTESIAN_POINT('Ctrl Pts',(-0.7911,-1.55819801506141E-13,-2.67313315082369));
#61928=CARTESIAN_POINT('Origin',(0.,0.,-5.925));
#61929=CARTESIAN_POINT('',(-0.792018129320091,-0.000125529594581231,-2.44466684917631));
#61930=CARTESIAN_POINT('',(-0.792074714116757,-0.00038587903788701,-2.47313315082369));
#61931=CARTESIAN_POINT('',(-0.7911,-9.68818082805471E-17,-5.925));
#61932=CARTESIAN_POINT('Ctrl Pts',(-0.792018129320091,-0.000125529594581231,
-2.44466684917631));
#61933=CARTESIAN_POINT('Ctrl Pts',(-0.791984392204006,0.11739493153915,
-2.44940335700203));
#61934=CARTESIAN_POINT('Ctrl Pts',(-0.764359052987853,0.23524448466125,
-2.45413986482774));
#61935=CARTESIAN_POINT('Ctrl Pts',(-0.713221964095025,0.341549151193039,
-2.45887637265346));
#61936=CARTESIAN_POINT('Ctrl Pts',(-0.656049434648901,0.460400396133606,
-2.46417190548492));
#61937=CARTESIAN_POINT('Ctrl Pts',(-0.569487705445131,0.564820772132129,
-2.46946743831638));
#61938=CARTESIAN_POINT('Ctrl Pts',(-0.463156154873996,0.641632782651323,
-2.47476297114785));
#61939=CARTESIAN_POINT('Ctrl Pts',(-0.356824604302849,0.718444793170525,
-2.48005850397931));
#61940=CARTESIAN_POINT('Ctrl Pts',(-0.23072323236434,0.767648438210387,
-2.48535403681077));
#61941=CARTESIAN_POINT('Ctrl Pts',(-0.0998597826367812,0.784463368145296,
-2.49064956964224));
#61942=CARTESIAN_POINT('Ctrl Pts',(0.0310036670907922,0.801278298080207,
-2.4959451024737));
#61943=CARTESIAN_POINT('Ctrl Pts',(0.166629194607407,0.785704512910156,
-2.50124063530517));
#61944=CARTESIAN_POINT('Ctrl Pts',(0.288811906477642,0.737525602510308,
-2.50653616813664));
#61945=CARTESIAN_POINT('Ctrl Pts',(0.533177330218084,0.641167781710625,
-2.51712723379956));
#61946=CARTESIAN_POINT('Ctrl Pts',(0.72377149137302,0.414389459991754,-2.52771829946249));
#61947=CARTESIAN_POINT('Ctrl Pts',(0.776265456590592,0.157426914113526,
-2.53830936512542));
#61948=CARTESIAN_POINT('Ctrl Pts',(0.802512439199381,0.0289456411743981,
-2.54360489795689));
#61949=CARTESIAN_POINT('Ctrl Pts',(0.794234372823836,-0.107081687804533,
-2.54890043078835));
#61950=CARTESIAN_POINT('Ctrl Pts',(0.755323031929162,-0.23330659827588,
-2.55419596361981));
#61951=CARTESIAN_POINT('Ctrl Pts',(0.716411691034492,-0.359531508747212,
-2.55949149645128));
#61952=CARTESIAN_POINT('Ctrl Pts',(0.646867075620673,-0.475954000710952,
-2.56478702928274));
#61953=CARTESIAN_POINT('Ctrl Pts',(0.5527558084356,-0.56716862598271,-2.57008256211421));
#61954=CARTESIAN_POINT('Ctrl Pts',(0.364533274065442,-0.749597876526237,
-2.58067362777714));
#61955=CARTESIAN_POINT('Ctrl Pts',(0.0780441326101909,-0.831195660301974,
-2.59126469344007));
#61956=CARTESIAN_POINT('Ctrl Pts',(-0.177206969668502,-0.772589442054205,
-2.601855759103));
#61957=CARTESIAN_POINT('Ctrl Pts',(-0.432458071947195,-0.713983223806436,
-2.61244682476593));
#61958=CARTESIAN_POINT('Ctrl Pts',(-0.656471135049315,-0.515173003535163,
-2.62303789042885));
#61959=CARTESIAN_POINT('Ctrl Pts',(-0.745459561574409,-0.268964806988401,
-2.63362895609178));
#61960=CARTESIAN_POINT('Ctrl Pts',(-0.7763738173256,-0.183432974891788,
-2.63730825378663));
#61961=CARTESIAN_POINT('Ctrl Pts',(-0.790992728343168,-0.0921809543713075,
-2.64098755148147));
#61962=CARTESIAN_POINT('Ctrl Pts',(-0.790257091081424,-0.000728948263829188,
-2.64466684917631));
#61963=CARTESIAN_POINT('Ctrl Pts',(-0.789984210644415,-0.000185547291381985,
-2.67313315082369));
#61964=CARTESIAN_POINT('Ctrl Pts',(-0.790630089050473,-0.0849598024118021,
-2.66972199263674));
#61965=CARTESIAN_POINT('Ctrl Pts',(-0.778080687464463,-0.169671162325107,
-2.6663108344498));
#61966=CARTESIAN_POINT('Ctrl Pts',(-0.751565426157115,-0.250011483509697,
-2.66289967626285));
#61967=CARTESIAN_POINT('Ctrl Pts',(-0.710402739147965,-0.374732996030462,
-2.65760414343139));
#61968=CARTESIAN_POINT('Ctrl Pts',(-0.63558244117862,-0.488920339945901,
-2.65230861059992));
#61969=CARTESIAN_POINT('Ctrl Pts',(-0.538920306497888,-0.578722433809465,
-2.64701307776846));
#61970=CARTESIAN_POINT('Ctrl Pts',(-0.442258171817167,-0.668524527673019,
-2.64171754493699));
#61971=CARTESIAN_POINT('Ctrl Pts',(-0.323754200425058,-0.733941371484708,
-2.63642201210553));
#61972=CARTESIAN_POINT('Ctrl Pts',(-0.196685444636518,-0.766499241642599,
-2.63112647927406));
#61973=CARTESIAN_POINT('Ctrl Pts',(-0.0696166888479782,-0.79905711180049,
-2.6258309464426));
#61974=CARTESIAN_POINT('Ctrl Pts',(0.0660168513370011,-0.798756008304586,
-2.62053541361114));
#61975=CARTESIAN_POINT('Ctrl Pts',(0.193933392624089,-0.766636310106404,
-2.61523988077967));
#61976=CARTESIAN_POINT('Ctrl Pts',(0.321849933911193,-0.734516611908218,
-2.60994434794821));
#61977=CARTESIAN_POINT('Ctrl Pts',(0.442049476300412,-0.670578319007744,
-2.60464881511674));
#61978=CARTESIAN_POINT('Ctrl Pts',(0.538131844813672,-0.581058646911393,
-2.59935328228528));
#61979=CARTESIAN_POINT('Ctrl Pts',(0.730296581840193,-0.402019302718692,
-2.58876221662235));
#61980=CARTESIAN_POINT('Ctrl Pts',(0.82599262336289,-0.12065444174251,-2.57817115095942));
#61981=CARTESIAN_POINT('Ctrl Pts',(0.780536751463461,0.137165611418776,
-2.56758008529649));
#61982=CARTESIAN_POINT('Ctrl Pts',(0.735080879564037,0.394985664580032,
-2.55698901963356));
#61983=CARTESIAN_POINT('Ctrl Pts',(0.548473094242492,0.629260909926376,
-2.54639795397063));
#61984=CARTESIAN_POINT('Ctrl Pts',(0.307050557510526,0.730764470404245,
-2.53580688830771));
#61985=CARTESIAN_POINT('Ctrl Pts',(0.065628020778533,0.832268030882126,
-2.52521582264478));
#61986=CARTESIAN_POINT('Ctrl Pts',(-0.230609267363913,0.800999906491504,
-2.51462475698184));
#61987=CARTESIAN_POINT('Ctrl Pts',(-0.447323677468425,0.653544766358459,
-2.50403369131891));
#61988=CARTESIAN_POINT('Ctrl Pts',(-0.555680882520669,0.579817196291946,
-2.49873815848745));
#61989=CARTESIAN_POINT('Ctrl Pts',(-0.644157368063439,0.47704287228983,
-2.49344262565599));
#61990=CARTESIAN_POINT('Ctrl Pts',(-0.704134940177837,0.359358925563953,
-2.48814709282452));
#61991=CARTESIAN_POINT('Ctrl Pts',(-0.760817922969531,0.248139399798586,
-2.48314244549091));
#61992=CARTESIAN_POINT('Ctrl Pts',(-0.792046912168715,0.123603245585912,
-2.4781377981573));
#61993=CARTESIAN_POINT('Ctrl Pts',(-0.792074714116757,-0.00038587903788701,
-2.47313315082369));
#61994=CARTESIAN_POINT('Origin',(0.,0.,-5.925));
#61995=CARTESIAN_POINT('',(-0.791060221705291,6.8858939410166E-5,-2.24466684917632));
#61996=CARTESIAN_POINT('',(-0.791211456379323,0.000596892318849943,-2.27313315082369));
#61997=CARTESIAN_POINT('',(-0.7911,-9.68818082805471E-17,-5.925));
#61998=CARTESIAN_POINT('Ctrl Pts',(-0.790839757919185,0.000450496766933234,
-2.24466684917631));
#61999=CARTESIAN_POINT('Ctrl Pts',(-0.790967177237201,0.0640755268736169,
-2.24722809685965));
#62000=CARTESIAN_POINT('Ctrl Pts',(-0.783524433324388,0.127612789595849,
-2.24978934454299));
#62001=CARTESIAN_POINT('Ctrl Pts',(-0.768375904261664,0.189221355350329,
-2.25235059222633));
#62002=CARTESIAN_POINT('Ctrl Pts',(-0.737055414048305,0.31660075124959,
-2.2576461250578));
#62003=CARTESIAN_POINT('Ctrl Pts',(-0.672794205261668,0.435735346289252,
-2.26294165788926));
#62004=CARTESIAN_POINT('Ctrl Pts',(-0.583936471318637,0.533266302717569,
-2.26823719072073));
#62005=CARTESIAN_POINT('Ctrl Pts',(-0.495078737375595,0.630797259145896,
-2.27353272355219));
#62006=CARTESIAN_POINT('Ctrl Pts',(-0.381624478276152,0.706724576962874,
-2.27882825638366));
#62007=CARTESIAN_POINT('Ctrl Pts',(-0.257309202990711,0.749098328484138,
-2.28412378921512));
#62008=CARTESIAN_POINT('Ctrl Pts',(-0.00867865241984256,0.833845831526662,
-2.29471485487805));
#62009=CARTESIAN_POINT('Ctrl Pts',(0.283395962895014,0.78437906938635,-2.30530592054098));
#62010=CARTESIAN_POINT('Ctrl Pts',(0.489751707774617,0.62250667234573,-2.31589698620391));
#62011=CARTESIAN_POINT('Ctrl Pts',(0.592929580214424,0.541570473825415,
-2.32119251903537));
#62012=CARTESIAN_POINT('Ctrl Pts',(0.674677735045415,0.43253286658002,-2.32648805186684));
#62013=CARTESIAN_POINT('Ctrl Pts',(0.726731869991776,0.311136048216823,
-2.3317835846983));
#62014=CARTESIAN_POINT('Ctrl Pts',(0.778786004938132,0.189739229853641,
-2.33707911752977));
#62015=CARTESIAN_POINT('Ctrl Pts',(0.801146119999865,0.0559832003726588,
-2.34237465036123));
#62016=CARTESIAN_POINT('Ctrl Pts',(0.788463385113155,-0.074462906163491,
-2.3476701831927));
#62017=CARTESIAN_POINT('Ctrl Pts',(0.763097915339735,-0.335355119235806,
-2.35826124885562));
#62018=CARTESIAN_POINT('Ctrl Pts',(0.597561045772532,-0.583007640528791,
-2.36885231451856));
#62019=CARTESIAN_POINT('Ctrl Pts',(0.365072122371674,-0.70357593871576,
-2.37944338018149));
#62020=CARTESIAN_POINT('Ctrl Pts',(0.132583198970817,-0.824144236902728,
-2.39003444584441));
#62021=CARTESIAN_POINT('Ctrl Pts',(-0.166857778263693,-0.817628311983679,
-2.40062551150734));
#62022=CARTESIAN_POINT('Ctrl Pts',(-0.394067412302621,-0.687577559190332,
-2.41121657717027));
#62023=CARTESIAN_POINT('Ctrl Pts',(-0.621277046341549,-0.557526806396985,
-2.4218076428332));
#62024=CARTESIAN_POINT('Ctrl Pts',(-0.776255337184895,-0.303941225729339,
-2.43239870849613));
#62025=CARTESIAN_POINT('Ctrl Pts',(-0.790870327881392,-0.0417032136632777,
-2.44298977415906));
#62026=CARTESIAN_POINT('Ctrl Pts',(-0.791641746501405,-0.0278615842306018,
-2.44354879916481));
#62027=CARTESIAN_POINT('Ctrl Pts',(-0.792022111133741,-0.0139958490110292,
-2.44410782417056));
#62028=CARTESIAN_POINT('Ctrl Pts',(-0.792018129320091,-0.000125529594581231,
-2.44466684917631));
#62029=CARTESIAN_POINT('Ctrl Pts',(-0.792074714116757,-0.00038587903788701,
-2.47313315082369));
#62030=CARTESIAN_POINT('Ctrl Pts',(-0.792076330051498,-0.00759250836469937,
-2.47284226532584));
#62031=CARTESIAN_POINT('Ctrl Pts',(-0.791972539265708,-0.0147972896658409,
-2.47255137982798));
#62032=CARTESIAN_POINT('Ctrl Pts',(-0.791762213259279,-0.02199750071887,
-2.47226049433013));
#62033=CARTESIAN_POINT('Ctrl Pts',(-0.784104297821294,-0.284155320933407,
-2.4616694286672));
#62034=CARTESIAN_POINT('Ctrl Pts',(-0.635215916763238,-0.540254503778407,
-2.45107836300427));
#62035=CARTESIAN_POINT('Ctrl Pts',(-0.410990726089976,-0.67708415632732,
-2.44048729734134));
#62036=CARTESIAN_POINT('Ctrl Pts',(-0.298878130753351,-0.745498982601772,
-2.43519176450988));
#62037=CARTESIAN_POINT('Ctrl Pts',(-0.167931333012931,-0.784096426302203,
-2.42989623167841));
#62038=CARTESIAN_POINT('Ctrl Pts',(-0.0361227386238225,-0.789968290442371,
-2.42460069884695));
#62039=CARTESIAN_POINT('Ctrl Pts',(0.0956858557653013,-0.79584015458254,
-2.41930516601548));
#62040=CARTESIAN_POINT('Ctrl Pts',(0.228356246803106,-0.768986439162439,
-2.41400963318402));
#62041=CARTESIAN_POINT('Ctrl Pts',(0.346283301642012,-0.711543481857892,
-2.40871410035255));
#62042=CARTESIAN_POINT('Ctrl Pts',(0.464210356480919,-0.654100524553346,
-2.40341856752109));
#62043=CARTESIAN_POINT('Ctrl Pts',(0.567394075120918,-0.566068325364358,
-2.39812303468962));
#62044=CARTESIAN_POINT('Ctrl Pts',(0.644098123696367,-0.458779903438533,
-2.39282750185816));
#62045=CARTESIAN_POINT('Ctrl Pts',(0.720802172271807,-0.35149148151272,
-2.38753196902669));
#62046=CARTESIAN_POINT('Ctrl Pts',(0.771026550782695,-0.224946836850083,
-2.38223643619523));
#62047=CARTESIAN_POINT('Ctrl Pts',(0.786308873044694,-0.0945166108377294,
-2.37694090336377));
#62048=CARTESIAN_POINT('Ctrl Pts',(0.816873517568692,0.166343841186993,
-2.36634983770084));
#62049=CARTESIAN_POINT('Ctrl Pts',(0.707669937097088,0.442746618610588,
-2.35575877203791));
#62050=CARTESIAN_POINT('Ctrl Pts',(0.506123452891804,0.609828726589603,
-2.34516770637498));
#62051=CARTESIAN_POINT('Ctrl Pts',(0.304576968686531,0.776910834568609,
-2.33457664071205));
#62052=CARTESIAN_POINT('Ctrl Pts',(0.0106875807475982,0.834672273103086,
-2.32398557504912));
#62053=CARTESIAN_POINT('Ctrl Pts',(-0.239031035420305,0.755751890621927,
-2.31339450938619));
#62054=CARTESIAN_POINT('Ctrl Pts',(-0.488749651588223,0.676831508140765,
-2.30280344372326));
#62055=CARTESIAN_POINT('Ctrl Pts',(-0.694297495985092,0.461229304643954,
-2.29221237806033));
#62056=CARTESIAN_POINT('Ctrl Pts',(-0.764019786897861,0.208549752545901,
-2.2816213123974));
#62057=CARTESIAN_POINT('Ctrl Pts',(-0.782645991581197,0.141046791942381,
-2.27879192520617));
#62058=CARTESIAN_POINT('Ctrl Pts',(-0.791578555337622,0.0708976834333845,
-2.27596253801493));
#62059=CARTESIAN_POINT('Ctrl Pts',(-0.791211456379323,0.000596892318849943,
-2.27313315082369));
#62060=CARTESIAN_POINT('Origin',(0.,0.,-5.925));
#62061=CARTESIAN_POINT('',(-0.7911,4.17277323805365E-13,-2.04466684917631));
#62062=CARTESIAN_POINT('',(-0.78949630379784,-0.000100922603766505,-2.07313315082369));
#62063=CARTESIAN_POINT('',(-0.7911,-9.68818082805471E-17,-5.925));
#62064=CARTESIAN_POINT('Ctrl Pts',(-0.7911,4.17277323805365E-13,-2.04466684917631));
#62065=CARTESIAN_POINT('Ctrl Pts',(-0.791099999999884,0.220167589667097,
-2.05352559274959));
#62066=CARTESIAN_POINT('Ctrl Pts',(-0.694214576672137,0.438610418339055,
-2.06238433632286));
#62067=CARTESIAN_POINT('Ctrl Pts',(-0.531017389080013,0.586395551223444,
-2.07124307989613));
#62068=CARTESIAN_POINT('Ctrl Pts',(-0.367820201487889,0.734180684107832,
-2.0801018234694));
#62069=CARTESIAN_POINT('Ctrl Pts',(-0.140868175871302,0.808992666571414,
-2.08896056704268));
#62070=CARTESIAN_POINT('Ctrl Pts',(0.0782205473251979,0.787223447298254,
-2.09781931061595));
#62071=CARTESIAN_POINT('Ctrl Pts',(0.297309270521698,0.765454228025093,
-2.10667805418922));
#62072=CARTESIAN_POINT('Ctrl Pts',(0.505102072675964,0.647444880833945,
-2.11553679776249));
#62073=CARTESIAN_POINT('Ctrl Pts',(0.636026795762001,0.47043503810061,-2.12439554133577));
#62074=CARTESIAN_POINT('Ctrl Pts',(0.766951518848038,0.293425195367275,
-2.13325428490904));
#62075=CARTESIAN_POINT('Ctrl Pts',(0.818956872247106,0.0601881960094517,
-2.14211302848231));
#62076=CARTESIAN_POINT('Ctrl Pts',(0.775631781004118,-0.155674501111709,
-2.15097177205558));
#62077=CARTESIAN_POINT('Ctrl Pts',(0.73230668976113,-0.371537198232871,
-2.15983051562886));
#62078=CARTESIAN_POINT('Ctrl Pts',(0.594329958849874,-0.566643518936855,
-2.16868925920213));
#62079=CARTESIAN_POINT('Ctrl Pts',(0.405242230243629,-0.67942471608499,
-2.1775480027754));
#62080=CARTESIAN_POINT('Ctrl Pts',(0.216154501637384,-0.792205913233125,
-2.18640674634868));
#62081=CARTESIAN_POINT('Ctrl Pts',(-0.0210816529305205,-0.820894963712991,
-2.19526548992195));
#62082=CARTESIAN_POINT('Ctrl Pts',(-0.231602780753685,-0.75643860421528,
-2.20412423349522));
#62083=CARTESIAN_POINT('Ctrl Pts',(-0.44212390857685,-0.691982244717568,
-2.21298297706849));
#62084=CARTESIAN_POINT('Ctrl Pts',(-0.62263162563451,-0.535390358803148,
-2.22184172064177));
#62085=CARTESIAN_POINT('Ctrl Pts',(-0.716163994722366,-0.336077881841848,
-2.23070046421504));
#62086=CARTESIAN_POINT('Ctrl Pts',(-0.765317280859623,-0.231334857514067,
-2.2353559258688));
#62087=CARTESIAN_POINT('Ctrl Pts',(-0.791100000000065,-0.115702837836063,
-2.24001138752256));
#62088=CARTESIAN_POINT('Ctrl Pts',(-0.7911,4.45199432874688E-13,-2.24466684917631));
#62089=CARTESIAN_POINT('Ctrl Pts',(-0.791211456379323,0.000596892318849943,
-2.27313315082369));
#62090=CARTESIAN_POINT('Ctrl Pts',(-0.790891486211103,-0.0606785633870678,
-2.27066700518346));
#62091=CARTESIAN_POINT('Ctrl Pts',(-0.783506390675429,-0.122069255167356,
-2.26820085954324));
#62092=CARTESIAN_POINT('Ctrl Pts',(-0.769317056038747,-0.181923386758272,
-2.26573471390301));
#62093=CARTESIAN_POINT('Ctrl Pts',(-0.738848422637895,-0.310447636814053,
-2.26043918107154));
#62094=CARTESIAN_POINT('Ctrl Pts',(-0.677006398750834,-0.431887023726298,
-2.25514364824008));
#62095=CARTESIAN_POINT('Ctrl Pts',(-0.589233752287982,-0.529315480170128,
-2.24984811540861));
#62096=CARTESIAN_POINT('Ctrl Pts',(-0.413688459362257,-0.724172393057811,
-2.23925704974568));
#62097=CARTESIAN_POINT('Ctrl Pts',(-0.134420676133361,-0.822985584071841,
-2.22866598408276));
#62098=CARTESIAN_POINT('Ctrl Pts',(0.125058712097984,-0.782123168183783,
-2.21807491841983));
#62099=CARTESIAN_POINT('Ctrl Pts',(0.254798406213642,-0.761691960239756,
-2.21277938558836));
#62100=CARTESIAN_POINT('Ctrl Pts',(0.37959100157991,-0.706341850570208,
-2.2074838527569));
#62101=CARTESIAN_POINT('Ctrl Pts',(0.48385546721716,-0.625490718551596,
-2.20218831992543));
#62102=CARTESIAN_POINT('Ctrl Pts',(0.588119932854422,-0.544639586532975,
-2.19689278709397));
#62103=CARTESIAN_POINT('Ctrl Pts',(0.671856268762669,-0.438287432165276,
-2.19159725426251));
#62104=CARTESIAN_POINT('Ctrl Pts',(0.724553349368237,-0.318164572964707,
-2.18630172143104));
#62105=CARTESIAN_POINT('Ctrl Pts',(0.777250429973799,-0.198041713764152,
-2.18100618859958));
#62106=CARTESIAN_POINT('Ctrl Pts',(0.798908255276695,-0.0641481497307185,
-2.17571065576811));
#62107=CARTESIAN_POINT('Ctrl Pts',(0.787917956791281,0.0672806518555208,
-2.17041512293665));
#62108=CARTESIAN_POINT('Ctrl Pts',(0.776927658305866,0.198709453441775,
-2.16511959010518));
#62109=CARTESIAN_POINT('Ctrl Pts',(0.733289236032133,0.327673492580847,
-2.15982405727372));
#62110=CARTESIAN_POINT('Ctrl Pts',(0.660502958879976,0.436979261365872,
-2.15452852444225));
#62111=CARTESIAN_POINT('Ctrl Pts',(0.514930404575669,0.655590798935909,
-2.14393745877932));
#62112=CARTESIAN_POINT('Ctrl Pts',(0.252766430757701,0.79556925508978,-2.1333463931164));
#62113=CARTESIAN_POINT('Ctrl Pts',(-0.00901145599943075,0.792446098483543,
-2.12275532745347));
#62114=CARTESIAN_POINT('Ctrl Pts',(-0.270789342756577,0.789322941877306,
-2.11216426179054));
#62115=CARTESIAN_POINT('Ctrl Pts',(-0.532181142452879,0.643098172510908,
-2.10157319612761));
#62116=CARTESIAN_POINT('Ctrl Pts',(-0.671425077549028,0.421289830533569,
-2.09098213046468));
#62117=CARTESIAN_POINT('Ctrl Pts',(-0.749647050727828,0.296686298142697,
-2.08503247058435));
#62118=CARTESIAN_POINT('Ctrl Pts',(-0.789322001462229,0.148230349834439,
-2.07908281070402));
#62119=CARTESIAN_POINT('Ctrl Pts',(-0.78949630379784,-0.000100922603766505,
-2.07313315082369));
#62120=CARTESIAN_POINT('Origin',(0.,0.,-5.925));
#62121=CARTESIAN_POINT('',(-0.7911,4.34319247233361E-13,-1.84466684917631));
#62122=CARTESIAN_POINT('',(-0.7914071948316,-0.000324170431651095,-1.87313315082369));
#62123=CARTESIAN_POINT('',(-0.7911,-9.68818082805471E-17,-5.925));
#62124=CARTESIAN_POINT('Ctrl Pts',(-0.7911,4.34319247233361E-13,-1.84466684917631));
#62125=CARTESIAN_POINT('Ctrl Pts',(-0.791099999999879,0.220167589667114,
-1.85352559274959));
#62126=CARTESIAN_POINT('Ctrl Pts',(-0.694214576672128,0.43861041833907,
-1.86238433632286));
#62127=CARTESIAN_POINT('Ctrl Pts',(-0.53101738908,0.586395551223455,-1.87124307989613));
#62128=CARTESIAN_POINT('Ctrl Pts',(-0.367820201487873,0.73418068410784,
-1.8801018234694));
#62129=CARTESIAN_POINT('Ctrl Pts',(-0.140868175871284,0.808992666571417,
-1.88896056704268));
#62130=CARTESIAN_POINT('Ctrl Pts',(0.0782205473252149,0.787223447298252,
-1.89781931061595));
#62131=CARTESIAN_POINT('Ctrl Pts',(0.297309270521714,0.765454228025087,
-1.90667805418922));
#62132=CARTESIAN_POINT('Ctrl Pts',(0.505102072675978,0.647444880833934,
-1.9155367977625));
#62133=CARTESIAN_POINT('Ctrl Pts',(0.636026795762011,0.470435038100596,
-1.92439554133577));
#62134=CARTESIAN_POINT('Ctrl Pts',(0.766951518848044,0.293425195367258,
-1.93325428490904));
#62135=CARTESIAN_POINT('Ctrl Pts',(0.818956872247108,0.060188196009434,
-1.94211302848231));
#62136=CARTESIAN_POINT('Ctrl Pts',(0.775631781004115,-0.155674501111726,
-1.95097177205558));
#62137=CARTESIAN_POINT('Ctrl Pts',(0.732306689761122,-0.371537198232887,
-1.95983051562886));
#62138=CARTESIAN_POINT('Ctrl Pts',(0.594329958849862,-0.566643518936868,
-1.96868925920213));
#62139=CARTESIAN_POINT('Ctrl Pts',(0.405242230243615,-0.679424716084999,
-1.9775480027754));
#62140=CARTESIAN_POINT('Ctrl Pts',(0.216154501637367,-0.79220591323313,
-1.98640674634868));
#62141=CARTESIAN_POINT('Ctrl Pts',(-0.0210816529305382,-0.82089496371299,
-1.99526548992195));
#62142=CARTESIAN_POINT('Ctrl Pts',(-0.231602780753701,-0.756438604215275,
-2.00412423349522));
#62143=CARTESIAN_POINT('Ctrl Pts',(-0.442123908576865,-0.691982244717559,
-2.0129829770685));
#62144=CARTESIAN_POINT('Ctrl Pts',(-0.622631625634521,-0.535390358803134,
-2.02184172064177));
#62145=CARTESIAN_POINT('Ctrl Pts',(-0.716163994722373,-0.336077881841833,
-2.03070046421504));
#62146=CARTESIAN_POINT('Ctrl Pts',(-0.765317280859622,-0.231334857514064,
-2.0353559258688));
#62147=CARTESIAN_POINT('Ctrl Pts',(-0.791100000000061,-0.115702837836076,
-2.04001138752256));
#62148=CARTESIAN_POINT('Ctrl Pts',(-0.7911,4.17277323805365E-13,-2.04466684917631));
#62149=CARTESIAN_POINT('Ctrl Pts',(-0.78949630379784,-0.000100922603766505,
-2.07313315082369));
#62150=CARTESIAN_POINT('Ctrl Pts',(-0.78963227927958,-0.115816045734007,
-2.06849174504109));
#62151=CARTESIAN_POINT('Ctrl Pts',(-0.765729109396082,-0.23145529412585,
-2.06385033925849));
#62152=CARTESIAN_POINT('Ctrl Pts',(-0.717334052693458,-0.33563535407461,
-2.05920893347589));
#62153=CARTESIAN_POINT('Ctrl Pts',(-0.662118537469595,-0.454497818095894,
-2.05391340064442));
#62154=CARTESIAN_POINT('Ctrl Pts',(-0.575021247009803,-0.558443535480751,
-2.04861786781296));
#62155=CARTESIAN_POINT('Ctrl Pts',(-0.468597849765866,-0.636679594895684,
-2.0433223349815));
#62156=CARTESIAN_POINT('Ctrl Pts',(-0.362174452521929,-0.714915654310618,
-2.03802680215003));
#62157=CARTESIAN_POINT('Ctrl Pts',(-0.23642494849386,-0.767442055755619,
-2.03273126931857));
#62158=CARTESIAN_POINT('Ctrl Pts',(-0.106454896091932,-0.784881295153073,
-2.0274357364871));
#62159=CARTESIAN_POINT('Ctrl Pts',(0.15348520871194,-0.819759773947982,
-2.01684467082417));
#62160=CARTESIAN_POINT('Ctrl Pts',(0.430307507011247,-0.71428960455265,
-2.00625360516124));
#62161=CARTESIAN_POINT('Ctrl Pts',(0.60162792982051,-0.515170035756479,
-1.99566253949832));
#62162=CARTESIAN_POINT('Ctrl Pts',(0.687288141225137,-0.415610251358399,
-1.99036700666685));
#62163=CARTESIAN_POINT('Ctrl Pts',(0.746572883757262,-0.292638117110115,
-1.98507147383539));
#62164=CARTESIAN_POINT('Ctrl Pts',(0.773703125728235,-0.163518272338253,
-1.97977594100392));
#62165=CARTESIAN_POINT('Ctrl Pts',(0.800833367699212,-0.0343984275663764,
-1.97448040817246));
#62166=CARTESIAN_POINT('Ctrl Pts',(0.795809109109027,0.100869127729068,
-1.96918487534099));
#62167=CARTESIAN_POINT('Ctrl Pts',(0.758212516041847,0.226539250656562,
-1.96388934250953));
#62168=CARTESIAN_POINT('Ctrl Pts',(0.720615922974666,0.352209373584056,
-1.95859380967806));
#62169=CARTESIAN_POINT('Ctrl Pts',(0.650446995430492,0.468282064143586,
-1.9532982768466));
#62170=CARTESIAN_POINT('Ctrl Pts',(0.556989537706041,0.561341293362837,
-1.94800274401513));
#62171=CARTESIAN_POINT('Ctrl Pts',(0.46353207998161,0.654400522582066,-1.94270721118367));
#62172=CARTESIAN_POINT('Ctrl Pts',(0.346786092076882,0.724446290461038,
-1.9374116783522));
#62173=CARTESIAN_POINT('Ctrl Pts',(0.220549705811982,0.760639770732056,
-1.93211614552074));
#62174=CARTESIAN_POINT('Ctrl Pts',(-0.0319230667178758,0.833026731274109,
-1.92152507985781));
#62175=CARTESIAN_POINT('Ctrl Pts',(-0.322357432688538,0.77000454138438,
-1.91093401419488));
#62176=CARTESIAN_POINT('Ctrl Pts',(-0.519860350901303,0.598161550838729,
-1.90034294853195));
#62177=CARTESIAN_POINT('Ctrl Pts',(-0.688997074953855,0.450999368450243,
-1.89127301596253));
#62178=CARTESIAN_POINT('Ctrl Pts',(-0.78997977571041,0.224030236294755,
-1.88220308339311));
#62179=CARTESIAN_POINT('Ctrl Pts',(-0.791972689379438,-0.000920914233180042,
-1.87313315082369));
#62180=CARTESIAN_POINT('Origin',(0.,0.,-5.925));
#62181=CARTESIAN_POINT('',(-0.7911,4.51416681812589E-13,-1.64466684917631));
#62182=CARTESIAN_POINT('',(-0.7911,-1.15518705712248E-13,-1.67313315082369));
#62183=CARTESIAN_POINT('',(-0.7911,-9.68818082805471E-17,-5.925));
#62184=CARTESIAN_POINT('Ctrl Pts',(-0.7911,4.51416681812589E-13,-1.64466684917631));
#62185=CARTESIAN_POINT('Ctrl Pts',(-0.791099999999874,0.220167589667131,
-1.65352559274959));
#62186=CARTESIAN_POINT('Ctrl Pts',(-0.694214576672118,0.438610418339085,
-1.66238433632286));
#62187=CARTESIAN_POINT('Ctrl Pts',(-0.531017389079988,0.586395551223466,
-1.67124307989613));
#62188=CARTESIAN_POINT('Ctrl Pts',(-0.367820201487857,0.734180684107848,
-1.6801018234694));
#62189=CARTESIAN_POINT('Ctrl Pts',(-0.140868175871267,0.80899266657142,
-1.68896056704268));
#62190=CARTESIAN_POINT('Ctrl Pts',(0.0782205473252319,0.78722344729825,
-1.69781931061595));
#62191=CARTESIAN_POINT('Ctrl Pts',(0.297309270521731,0.76545422802508,-1.70667805418922));
#62192=CARTESIAN_POINT('Ctrl Pts',(0.505102072675992,0.647444880833923,
-1.7155367977625));
#62193=CARTESIAN_POINT('Ctrl Pts',(0.636026795762021,0.470435038100582,
-1.72439554133577));
#62194=CARTESIAN_POINT('Ctrl Pts',(0.76695151884805,0.293425195367242,-1.73325428490904));
#62195=CARTESIAN_POINT('Ctrl Pts',(0.818956872247109,0.0601881960094164,
-1.74211302848231));
#62196=CARTESIAN_POINT('Ctrl Pts',(0.775631781004111,-0.155674501111743,
-1.75097177205559));
#62197=CARTESIAN_POINT('Ctrl Pts',(0.732306689761114,-0.371537198232902,
-1.75983051562886));
#62198=CARTESIAN_POINT('Ctrl Pts',(0.59432995884985,-0.566643518936881,
-1.76868925920213));
#62199=CARTESIAN_POINT('Ctrl Pts',(0.4052422302436,-0.679424716085008,-1.7775480027754));
#62200=CARTESIAN_POINT('Ctrl Pts',(0.21615450163735,-0.792205913233134,
-1.78640674634868));
#62201=CARTESIAN_POINT('Ctrl Pts',(-0.021081652930556,-0.82089496371299,
-1.79526548992195));
#62202=CARTESIAN_POINT('Ctrl Pts',(-0.231602780753718,-0.75643860421527,
-1.80412423349522));
#62203=CARTESIAN_POINT('Ctrl Pts',(-0.44212390857688,-0.691982244717549,
-1.8129829770685));
#62204=CARTESIAN_POINT('Ctrl Pts',(-0.622631625634533,-0.535390358803121,
-1.82184172064177));
#62205=CARTESIAN_POINT('Ctrl Pts',(-0.71616399472238,-0.336077881841817,
-1.83070046421504));
#62206=CARTESIAN_POINT('Ctrl Pts',(-0.765317280859627,-0.231334857514047,
-1.8353559258688));
#62207=CARTESIAN_POINT('Ctrl Pts',(-0.791100000000064,-0.115702837836059,
-1.84001138752256));
#62208=CARTESIAN_POINT('Ctrl Pts',(-0.7911,4.34319247233361E-13,-1.84466684917631));
#62209=CARTESIAN_POINT('Ctrl Pts',(-0.7911,-8.75965966429249E-14,-1.87313315082369));
#62210=CARTESIAN_POINT('Ctrl Pts',(-0.791099999999976,-0.220167589666752,
-1.86427440725042));
#62211=CARTESIAN_POINT('Ctrl Pts',(-0.694214576672334,-0.438610418338736,
-1.85541566367715));
#62212=CARTESIAN_POINT('Ctrl Pts',(-0.531017389080291,-0.586395551223192,
-1.84655692010388));
#62213=CARTESIAN_POINT('Ctrl Pts',(-0.367820201488247,-0.734180684107648,
-1.8376981765306));
#62214=CARTESIAN_POINT('Ctrl Pts',(-0.140868175871716,-0.808992666571338,
-1.82883943295733));
#62215=CARTESIAN_POINT('Ctrl Pts',(0.0782205473247804,-0.787223447298295,
-1.81998068938406));
#62216=CARTESIAN_POINT('Ctrl Pts',(0.297309270521277,-0.765454228025253,
-1.81112194581079));
#62217=CARTESIAN_POINT('Ctrl Pts',(0.505102072675593,-0.647444880834229,
-1.80226320223752));
#62218=CARTESIAN_POINT('Ctrl Pts',(0.636026795761725,-0.470435038100983,
-1.79340445866424));
#62219=CARTESIAN_POINT('Ctrl Pts',(0.766951518847857,-0.293425195367737,
-1.78454571509097));
#62220=CARTESIAN_POINT('Ctrl Pts',(0.818956872247065,-0.0601881960099645,
-1.7756869715177));
#62221=CARTESIAN_POINT('Ctrl Pts',(0.775631781004219,0.15567450111121,-1.76682822794443));
#62222=CARTESIAN_POINT('Ctrl Pts',(0.732306689761372,0.371537198232384,
-1.75796948437115));
#62223=CARTESIAN_POINT('Ctrl Pts',(0.594329958850259,0.566643518936446,
-1.74911074079788));
#62224=CARTESIAN_POINT('Ctrl Pts',(0.405242230244105,0.679424716084706,
-1.74025199722461));
#62225=CARTESIAN_POINT('Ctrl Pts',(0.216154501637952,0.792205913232966,
-1.73139325365134));
#62226=CARTESIAN_POINT('Ctrl Pts',(-0.0210816529299128,0.820894963713003,
-1.72253451007807));
#62227=CARTESIAN_POINT('Ctrl Pts',(-0.231602780753112,0.756438604215455,
-1.71367576650479));
#62228=CARTESIAN_POINT('Ctrl Pts',(-0.442123908576311,0.691982244717908,
-1.70481702293152));
#62229=CARTESIAN_POINT('Ctrl Pts',(-0.62263162563408,0.535390358803641,
-1.69595827935825));
#62230=CARTESIAN_POINT('Ctrl Pts',(-0.716163994722092,0.336077881842432,
-1.68709953578498));
#62231=CARTESIAN_POINT('Ctrl Pts',(-0.765317280859473,0.231334857514609,
-1.68244407413122));
#62232=CARTESIAN_POINT('Ctrl Pts',(-0.79110000000001,0.115702837836528,
-1.67778861247745));
#62233=CARTESIAN_POINT('Ctrl Pts',(-0.7911,-7.05546732149287E-14,-1.67313315082369));
#62234=CARTESIAN_POINT('Origin',(0.,0.,-5.925));
#62235=CARTESIAN_POINT('',(-0.790643101388239,0.000413675204086472,-1.44466684917632));
#62236=CARTESIAN_POINT('',(-0.790455823492844,-7.84331714051887E-5,-1.4731331508237));
#62237=CARTESIAN_POINT('',(-0.7911,-9.68818082805471E-17,-5.925));
#62238=CARTESIAN_POINT('Ctrl Pts',(-0.790643101388239,0.000413675204086472,
-1.44466684917632));
#62239=CARTESIAN_POINT('Ctrl Pts',(-0.790904615161135,0.111330088002923,
-1.44911812195309));
#62240=CARTESIAN_POINT('Ctrl Pts',(-0.76848813566008,0.22195367907901,-1.45356939472987));
#62241=CARTESIAN_POINT('Ctrl Pts',(-0.723356415587075,0.322451128215468,
-1.45802066750665));
#62242=CARTESIAN_POINT('Ctrl Pts',(-0.615972969380901,0.561568148478508,
-1.46861173316958));
#62243=CARTESIAN_POINT('Ctrl Pts',(-0.379993291021312,0.743358736491673,
-1.47920279883251));
#62244=CARTESIAN_POINT('Ctrl Pts',(-0.121169674969144,0.783335602370142,
-1.48979386449544));
#62245=CARTESIAN_POINT('Ctrl Pts',(0.137653941083039,0.823312468248613,
-1.50038493015837));
#62246=CARTESIAN_POINT('Ctrl Pts',(0.419321494827788,0.721475611992372,
-1.51097599582129));
#62247=CARTESIAN_POINT('Ctrl Pts',(0.593077223590446,0.525653338426826,
-1.52156706148422));
#62248=CARTESIAN_POINT('Ctrl Pts',(0.766832952353103,0.329831064861279,
-1.53215812714715));
#62249=CARTESIAN_POINT('Ctrl Pts',(0.832676856133661,0.0400233739863956,
-1.54274919281008));
#62250=CARTESIAN_POINT('Ctrl Pts',(0.76274880853202,-0.213141475635434,
-1.55334025847301));
#62251=CARTESIAN_POINT('Ctrl Pts',(0.727784784731201,-0.339723900446341,
-1.55863579130448));
#62252=CARTESIAN_POINT('Ctrl Pts',(0.658877773084845,-0.457145614943989,
-1.56393132413594));
#62253=CARTESIAN_POINT('Ctrl Pts',(0.566731889921311,-0.551503724098459,
-1.5692268569674));
#62254=CARTESIAN_POINT('Ctrl Pts',(0.474586006757777,-0.64586183325293,
-1.57452238979887));
#62255=CARTESIAN_POINT('Ctrl Pts',(0.359201252077072,-0.717156337064215,
-1.57981792263033));
#62256=CARTESIAN_POINT('Ctrl Pts',(0.233902728280942,-0.755973389262662,
-1.5851134554618));
#62257=CARTESIAN_POINT('Ctrl Pts',(0.108604204484811,-0.794790441461109,
-1.59040898829326));
#62258=CARTESIAN_POINT('Ctrl Pts',(-0.0266080884267369,-0.801130042046715,
-1.59570452112473));
#62259=CARTESIAN_POINT('Ctrl Pts',(-0.155985688497453,-0.775256871710341,
-1.60100005395619));
#62260=CARTESIAN_POINT('Ctrl Pts',(-0.285363288568183,-0.749383701373963,
-1.60629558678765));
#62261=CARTESIAN_POINT('Ctrl Pts',(-0.408906195798072,-0.691297760115601,
-1.61159111961912));
#62262=CARTESIAN_POINT('Ctrl Pts',(-0.509294381945595,-0.606609894578137,
-1.61688665245058));
#62263=CARTESIAN_POINT('Ctrl Pts',(-0.684838791977828,-0.458519945320396,
-1.62614671802583));
#62264=CARTESIAN_POINT('Ctrl Pts',(-0.789580741841121,-0.229086684800661,
-1.63540678360107));
#62265=CARTESIAN_POINT('Ctrl Pts',(-0.79151332369587,0.000198305622813172,
-1.64466684917632));
#62266=CARTESIAN_POINT('Ctrl Pts',(-0.7911,-7.05546732149287E-14,-1.67313315082369));
#62267=CARTESIAN_POINT('Ctrl Pts',(-0.79109999999998,-0.22016758966675,
-1.66427440725042));
#62268=CARTESIAN_POINT('Ctrl Pts',(-0.694214576672329,-0.438610418338751,
-1.65541566367715));
#62269=CARTESIAN_POINT('Ctrl Pts',(-0.53101738908027,-0.586395551223211,
-1.64655692010387));
#62270=CARTESIAN_POINT('Ctrl Pts',(-0.36782020148821,-0.734180684107671,
-1.6376981765306));
#62271=CARTESIAN_POINT('Ctrl Pts',(-0.140868175871656,-0.808992666571353,
-1.62883943295733));
#62272=CARTESIAN_POINT('Ctrl Pts',(0.078220547324853,-0.787223447298288,
-1.61998068938406));
#62273=CARTESIAN_POINT('Ctrl Pts',(0.297309270521362,-0.765454228025224,
-1.61112194581078));
#62274=CARTESIAN_POINT('Ctrl Pts',(0.50510207267568,-0.647444880834166,
-1.60226320223751));
#62275=CARTESIAN_POINT('Ctrl Pts',(0.636026795761795,-0.470435038100888,
-1.59340445866424));
#62276=CARTESIAN_POINT('Ctrl Pts',(0.766951518847909,-0.293425195367611,
-1.58454571509097));
#62277=CARTESIAN_POINT('Ctrl Pts',(0.81895687224708,-0.0601881960098106,
-1.57568697151769));
#62278=CARTESIAN_POINT('Ctrl Pts',(0.775631781004187,0.15567450111137,-1.56682822794442));
#62279=CARTESIAN_POINT('Ctrl Pts',(0.732306689761293,0.37153719823255,-1.55796948437115));
#62280=CARTESIAN_POINT('Ctrl Pts',(0.594329958850123,0.566643518936595,
-1.54911074079787));
#62281=CARTESIAN_POINT('Ctrl Pts',(0.405242230243927,0.679424716084813,
-1.5402519972246));
#62282=CARTESIAN_POINT('Ctrl Pts',(0.216154501637731,0.79220591323303,-1.53139325365133));
#62283=CARTESIAN_POINT('Ctrl Pts',(-0.0210816529301607,0.820894963713,-1.52253451007806));
#62284=CARTESIAN_POINT('Ctrl Pts',(-0.231602780753354,0.756438604215381,
-1.51367576650478));
#62285=CARTESIAN_POINT('Ctrl Pts',(-0.442123908576547,0.691982244717762,
-1.50481702293151));
#62286=CARTESIAN_POINT('Ctrl Pts',(-0.622631625634275,0.535390358803421,
-1.49595827935824));
#62287=CARTESIAN_POINT('Ctrl Pts',(-0.716163994722218,0.336077881842162,
-1.48709953578497));
#62288=CARTESIAN_POINT('Ctrl Pts',(-0.765317280859516,0.231334857514416,
-1.48244407413121));
#62289=CARTESIAN_POINT('Ctrl Pts',(-0.791100000000008,0.11570283783644,
-1.47778861247745));
#62290=CARTESIAN_POINT('Ctrl Pts',(-0.7911,-5.35127497869325E-14,-1.47313315082369));
#62291=CARTESIAN_POINT('Origin',(0.,0.,-5.925));
#62292=CARTESIAN_POINT('',(-0.790116780300585,-0.000593511115090206,-1.24466684917632));
#62293=CARTESIAN_POINT('',(-0.791419810366198,-0.000275355779050857,-1.27313315082369));
#62294=CARTESIAN_POINT('',(-0.7911,-9.68818082805471E-17,-5.925));
#62295=CARTESIAN_POINT('Ctrl Pts',(-0.790116780300585,-0.000593511115090206,
-1.24466684917632));
#62296=CARTESIAN_POINT('Ctrl Pts',(-0.788689659215958,0.187798474330122,
-1.25223839464219));
#62297=CARTESIAN_POINT('Ctrl Pts',(-0.721977966372551,0.377047291568571,
-1.25980994010805));
#62298=CARTESIAN_POINT('Ctrl Pts',(-0.599448613644661,0.518611719566975,
-1.26738148557392));
#62299=CARTESIAN_POINT('Ctrl Pts',(-0.428054751423635,0.716631814569354,
-1.27797255123685));
#62300=CARTESIAN_POINT('Ctrl Pts',(-0.147445993055172,0.821350871343271,
-1.28856361689978));
#62301=CARTESIAN_POINT('Ctrl Pts',(0.111755050952167,0.784578124808293,
-1.29915468256271));
#62302=CARTESIAN_POINT('Ctrl Pts',(0.370956094959505,0.747805378273315,
-1.30974574822564));
#62303=CARTESIAN_POINT('Ctrl Pts',(0.608749424605719,0.569540828429441,
-1.32033681388857));
#62304=CARTESIAN_POINT('Ctrl Pts',(0.719337787722662,0.331312813979979,
-1.3309278795515));
#62305=CARTESIAN_POINT('Ctrl Pts',(0.774631969281131,0.212198806755254,
-1.33622341238296));
#62306=CARTESIAN_POINT('Ctrl Pts',(0.798124909207285,0.0780939333791335,
-1.34151894521443));
#62307=CARTESIAN_POINT('Ctrl Pts',(0.788975113880318,-0.0534758115954189,
-1.34681447804589));
#62308=CARTESIAN_POINT('Ctrl Pts',(0.77982531855335,-0.185045556570001,
-1.35211001087735));
#62309=CARTESIAN_POINT('Ctrl Pts',(0.738032787973245,-0.314080173143015,
-1.35740554370882));
#62310=CARTESIAN_POINT('Ctrl Pts',(0.66765971662573,-0.424778476815616,
-1.36270107654029));
#62311=CARTESIAN_POINT('Ctrl Pts',(0.597286645278231,-0.535476780488192,
-1.36799660937175));
#62312=CARTESIAN_POINT('Ctrl Pts',(0.498333033163336,-0.627838771260365,
-1.37329214220321));
#62313=CARTESIAN_POINT('Ctrl Pts',(0.382973555042227,-0.691871381319134,
-1.37858767503468));
#62314=CARTESIAN_POINT('Ctrl Pts',(0.267614076921119,-0.755903991377902,
-1.38388320786614));
#62315=CARTESIAN_POINT('Ctrl Pts',(0.135848732793798,-0.791607220723266,
-1.38917874069761));
#62316=CARTESIAN_POINT('Ctrl Pts',(0.00451088429379835,-0.792045442890957,
-1.39447427352907));
#62317=CARTESIAN_POINT('Ctrl Pts',(-0.258164812706215,-0.792921887226339,
-1.405065339192));
#62318=CARTESIAN_POINT('Ctrl Pts',(-0.519130527196939,-0.652738302851012,
-1.41565640485493));
#62319=CARTESIAN_POINT('Ctrl Pts',(-0.66295912681962,-0.433424143939486,
-1.42624747051786));
#62320=CARTESIAN_POINT('Ctrl Pts',(-0.734873426630964,-0.323767064483717,
-1.43154300334932));
#62321=CARTESIAN_POINT('Ctrl Pts',(-0.777503447725295,-0.194327341393895,
-1.43683853618079));
#62322=CARTESIAN_POINT('Ctrl Pts',(-0.788047125740096,-0.0626624207519821,
-1.44213406901225));
#62323=CARTESIAN_POINT('Ctrl Pts',(-0.789728090897084,-0.0416712501485153,
-1.44297832906694));
#62324=CARTESIAN_POINT('Ctrl Pts',(-0.790593500826045,-0.0206235205444637,
-1.44382258912163));
#62325=CARTESIAN_POINT('Ctrl Pts',(-0.790643101388239,0.000413675204086472,
-1.44466684917632));
#62326=CARTESIAN_POINT('Ctrl Pts',(-0.78954155091179,-0.000189752502548938,
-1.47313315082369));
#62327=CARTESIAN_POINT('Ctrl Pts',(-0.789371393251466,-0.146463581773617,
-1.46726149744544));
#62328=CARTESIAN_POINT('Ctrl Pts',(-0.750711606351124,-0.292708100538373,
-1.46138984406718));
#62329=CARTESIAN_POINT('Ctrl Pts',(-0.67442271127103,-0.416180287691346,
-1.45551819068893));
#62330=CARTESIAN_POINT('Ctrl Pts',(-0.536815695819837,-0.638894735810089,
-1.444927125026));
#62331=CARTESIAN_POINT('Ctrl Pts',(-0.276780209019268,-0.78751809107129,
-1.43433605936307));
#62332=CARTESIAN_POINT('Ctrl Pts',(-0.0149350547827386,-0.792511009520599,
-1.42374499370014));
#62333=CARTESIAN_POINT('Ctrl Pts',(0.246910099453776,-0.797503927969907,
-1.41315392803721));
#62334=CARTESIAN_POINT('Ctrl Pts',(0.510564921126274,-0.658866409607309,
-1.40256286237428));
#62335=CARTESIAN_POINT('Ctrl Pts',(0.657357033665679,-0.441702348135788,
-1.39197179671135));
#62336=CARTESIAN_POINT('Ctrl Pts',(0.73075308993539,-0.333120317400014,
-1.38667626387989));
#62337=CARTESIAN_POINT('Ctrl Pts',(0.774933468921821,-0.204906650887048,
-1.38138073104843));
#62338=CARTESIAN_POINT('Ctrl Pts',(0.787121134869292,-0.0733837202913743,
-1.37608519821696));
#62339=CARTESIAN_POINT('Ctrl Pts',(0.799308800816764,0.0581392103042997,
-1.3707896653855));
#62340=CARTESIAN_POINT('Ctrl Pts',(0.779503753725249,0.192971404982673,
-1.36549413255403));
#62341=CARTESIAN_POINT('Ctrl Pts',(0.727456171333946,0.313334982361156,
-1.36019859972257));
#62342=CARTESIAN_POINT('Ctrl Pts',(0.623361006551351,0.554062137118093,
-1.34960753405964));
#62343=CARTESIAN_POINT('Ctrl Pts',(0.390295700569642,0.736914822675632,
-1.33901646839671));
#62344=CARTESIAN_POINT('Ctrl Pts',(0.131359649808987,0.781089606948847,
-1.32842540273378));
#62345=CARTESIAN_POINT('Ctrl Pts',(0.00189162442864507,0.803176999085456,
-1.32312986990231));
#62346=CARTESIAN_POINT('Ctrl Pts',(-0.134044087146429,0.790594915900975,
-1.31783433707085));
#62347=CARTESIAN_POINT('Ctrl Pts',(-0.258674226552509,0.747290035172147,
-1.31253880423938));
#62348=CARTESIAN_POINT('Ctrl Pts',(-0.383304365958575,0.703985154443324,
-1.30724327140792));
#62349=CARTESIAN_POINT('Ctrl Pts',(-0.496628933195643,0.629957476170163,
-1.30194773857646));
#62350=CARTESIAN_POINT('Ctrl Pts',(-0.584940139616044,0.53296461855972,
-1.29665220574499));
#62351=CARTESIAN_POINT('Ctrl Pts',(-0.673251346036456,0.435971760949266,
-1.29135667291353));
#62352=CARTESIAN_POINT('Ctrl Pts',(-0.736549191640189,0.316013724001529,
-1.28606114008206));
#62353=CARTESIAN_POINT('Ctrl Pts',(-0.768122374764371,0.187961193161232,
-1.2807656072506));
#62354=CARTESIAN_POINT('Ctrl Pts',(-0.783291194228088,0.126440448973076,
-1.2782214551083));
#62355=CARTESIAN_POINT('Ctrl Pts',(-0.791137438528416,0.0630513621358539,
-1.27567730296599));
#62356=CARTESIAN_POINT('Ctrl Pts',(-0.791419810366198,-0.000275355779050857,
-1.27313315082369));
#62357=CARTESIAN_POINT('Origin',(0.,0.,-5.925));
#62358=CARTESIAN_POINT('',(-0.792649648621414,-0.000247240842943735,-1.04466684917632));
#62359=CARTESIAN_POINT('',(-0.791304392674353,0.000147799391554101,-1.07313315082369));
#62360=CARTESIAN_POINT('',(-0.7911,-9.68818082805471E-17,-5.925));
#62361=CARTESIAN_POINT('Ctrl Pts',(-0.792649648621414,-0.000247240842943735,
-1.04466684917632));
#62362=CARTESIAN_POINT('Ctrl Pts',(-0.792652320571416,0.00224400151945376,
-1.04476760166835));
#62363=CARTESIAN_POINT('Ctrl Pts',(-0.792642050515285,0.00473530815100578,
-1.04486835416038));
#62364=CARTESIAN_POINT('Ctrl Pts',(-0.792618781414662,0.00722657743760985,
-1.04496910665241));
#62365=CARTESIAN_POINT('Ctrl Pts',(-0.790172741940626,0.269107907285088,
-1.05556017231534));
#62366=CARTESIAN_POINT('Ctrl Pts',(-0.644085458455419,0.530576570280527,
-1.06615123797827));
#62367=CARTESIAN_POINT('Ctrl Pts',(-0.422719876558179,0.670343144444435,
-1.0767423036412));
#62368=CARTESIAN_POINT('Ctrl Pts',(-0.20135429466094,0.810109718608342,
-1.08733336930413));
#62369=CARTESIAN_POINT('Ctrl Pts',(0.0952895856483443,0.828174203940726,
-1.09792443496705));
#62370=CARTESIAN_POINT('Ctrl Pts',(0.333796502775129,0.718188643942634,
-1.10851550062998));
#62371=CARTESIAN_POINT('Ctrl Pts',(0.453049961338528,0.663195863943586,
-1.11381103346145));
#62372=CARTESIAN_POINT('Ctrl Pts',(0.557769179106307,0.576190572611911,
-1.11910656629292));
#62373=CARTESIAN_POINT('Ctrl Pts',(0.635967282330499,0.469986179108929,
-1.12440209912438));
#62374=CARTESIAN_POINT('Ctrl Pts',(0.714165385554682,0.363781785605958,
-1.12969763195584));
#62375=CARTESIAN_POINT('Ctrl Pts',(0.765842374235291,0.238378289931675,
-1.13499316478731));
#62376=CARTESIAN_POINT('Ctrl Pts',(0.783865480633038,0.10844888124126,-1.14028869761877));
#62377=CARTESIAN_POINT('Ctrl Pts',(0.801888587030786,-0.0214805274491695,
-1.14558423045024));
#62378=CARTESIAN_POINT('Ctrl Pts',(0.786257811145676,-0.155935849155701,
-1.1508797632817));
#62379=CARTESIAN_POINT('Ctrl Pts',(0.739783541611409,-0.27941915415914,
-1.15617529611317));
#62380=CARTESIAN_POINT('Ctrl Pts',(0.693309272077147,-0.402902459162565,
-1.16147082894463));
#62381=CARTESIAN_POINT('Ctrl Pts',(0.615991508893732,-0.515413747462867,
-1.16676636177609));
#62382=CARTESIAN_POINT('Ctrl Pts',(0.516170691110303,-0.600769630823793,
-1.17206189460756));
#62383=CARTESIAN_POINT('Ctrl Pts',(0.316529055543421,-0.771481397545664,
-1.18265296027049));
#62384=CARTESIAN_POINT('Ctrl Pts',(0.0268752015764362,-0.833571544510021,
-1.19324402593342));
#62385=CARTESIAN_POINT('Ctrl Pts',(-0.224723188338764,-0.759520099145486,
-1.20383509159635));
#62386=CARTESIAN_POINT('Ctrl Pts',(-0.35052238329635,-0.722494376463222,
-1.20913062442781));
#62387=CARTESIAN_POINT('Ctrl Pts',(-0.466807712240998,-0.651433255698741,
-1.21442615725928));
#62388=CARTESIAN_POINT('Ctrl Pts',(-0.560077612187121,-0.557904937859935,
-1.21972169009074));
#62389=CARTESIAN_POINT('Ctrl Pts',(-0.653347512133266,-0.464376620021107,
-1.22501722292221));
#62390=CARTESIAN_POINT('Ctrl Pts',(-0.723601983080881,-0.348381105107937,
-1.23031275575367));
#62391=CARTESIAN_POINT('Ctrl Pts',(-0.760075136033682,-0.222497239627344,
-1.23560828858514));
#62392=CARTESIAN_POINT('Ctrl Pts',(-0.780872178653654,-0.150718084176908,
-1.2386278087822));
#62393=CARTESIAN_POINT('Ctrl Pts',(-0.790685913901923,-0.0757239329794748,
-1.24164732897926));
#62394=CARTESIAN_POINT('Ctrl Pts',(-0.790116780300585,-0.000593511115090206,
-1.24466684917632));
#62395=CARTESIAN_POINT('Ctrl Pts',(-0.791419810366198,-0.000275355779050857,
-1.27313315082369));
#62396=CARTESIAN_POINT('Ctrl Pts',(-0.791725182206475,-0.0687602179388454,
-1.27038177013453));
#62397=CARTESIAN_POINT('Ctrl Pts',(-0.783184299960073,-0.137172137127078,
-1.26763038944537));
#62398=CARTESIAN_POINT('Ctrl Pts',(-0.76549197012783,-0.2030691439458,-1.26487900875621));
#62399=CARTESIAN_POINT('Ctrl Pts',(-0.697387753317123,-0.456730707013651,
-1.25428794309328));
#62400=CARTESIAN_POINT('Ctrl Pts',(-0.493681020306463,-0.673127297285795,
-1.24369687743035));
#62401=CARTESIAN_POINT('Ctrl Pts',(-0.244623479252935,-0.753797969444869,
-1.23310581176742));
#62402=CARTESIAN_POINT('Ctrl Pts',(0.00443406180057812,-0.834468641603939,
-1.22251474610449));
#62403=CARTESIAN_POINT('Ctrl Pts',(0.298842410896965,-0.779413395649963,
-1.21192368044156));
#62404=CARTESIAN_POINT('Ctrl Pts',(0.501650560616659,-0.613712857210694,
-1.20133261477863));
#62405=CARTESIAN_POINT('Ctrl Pts',(0.704458710336341,-0.448012318771434,
-1.1907415491157));
#62406=CARTESIAN_POINT('Ctrl Pts',(0.815666660679348,-0.171666487846932,
-1.18015048345277));
#62407=CARTESIAN_POINT('Ctrl Pts',(0.786968579401671,0.0888801951670066,
-1.16955941778984));
#62408=CARTESIAN_POINT('Ctrl Pts',(0.772619538762829,0.219153536674006,
-1.16426388495838));
#62409=CARTESIAN_POINT('Ctrl Pts',(0.723293990218791,0.345477091203361,
-1.15896835212691));
#62410=CARTESIAN_POINT('Ctrl Pts',(0.647441629484383,0.453612376123417,
-1.15367281929545));
#62411=CARTESIAN_POINT('Ctrl Pts',(0.571589268749992,0.561747661043449,
-1.14837728646398));
#62412=CARTESIAN_POINT('Ctrl Pts',(0.469210095825238,0.651694676354199,
-1.14308175363252));
#62413=CARTESIAN_POINT('Ctrl Pts',(0.351622253064786,0.709741561085972,
-1.13778622080105));
#62414=CARTESIAN_POINT('Ctrl Pts',(0.116446567543868,0.825835330549523,
-1.12719515513813));
#62415=CARTESIAN_POINT('Ctrl Pts',(-0.179563797319874,0.814328577697159,
-1.11660408947519));
#62416=CARTESIAN_POINT('Ctrl Pts',(-0.40551913086259,0.680375312739883,
-1.10601302381227));
#62417=CARTESIAN_POINT('Ctrl Pts',(-0.518496797633955,0.613398680261241,
-1.1007174909808));
#62418=CARTESIAN_POINT('Ctrl Pts',(-0.613960706575066,0.515810419756364,
-1.09542195814934));
#62419=CARTESIAN_POINT('Ctrl Pts',(-0.680919134805824,0.402124214646937,
-1.09012642531787));
#62420=CARTESIAN_POINT('Ctrl Pts',(-0.747877563036576,0.288438009537523,
-1.08483089248641));
#62421=CARTESIAN_POINT('Ctrl Pts',(-0.786330510556985,0.158653859823556,
-1.07953535965494));
#62422=CARTESIAN_POINT('Ctrl Pts',(-0.790851939689893,0.0275583210533076,
-1.07423982682348));
#62423=CARTESIAN_POINT('Ctrl Pts',(-0.791166906868543,0.0184260775156362,
-1.07387093482355));
#62424=CARTESIAN_POINT('Ctrl Pts',(-0.791317216198072,0.00928747026329368,
-1.07350204282362));
#62425=CARTESIAN_POINT('Ctrl Pts',(-0.791304392674353,0.000147799391554101,
-1.07313315082369));
#62426=CARTESIAN_POINT('Origin',(0.,0.,-5.925));
#62427=CARTESIAN_POINT('',(-0.790929060525409,0.000272143640698088,-0.844666849176317));
#62428=CARTESIAN_POINT('',(-0.7911,-2.33146835171283E-15,-0.873133150823696));
#62429=CARTESIAN_POINT('',(-0.7911,-9.68818082805471E-17,-5.925));
#62430=CARTESIAN_POINT('Ctrl Pts',(-0.790491490569074,0.000968775477774575,
-0.844666849176317));
#62431=CARTESIAN_POINT('Ctrl Pts',(-0.791140089290106,0.0812481867562639,
-0.84788787435744));
#62432=CARTESIAN_POINT('Ctrl Pts',(-0.779937728478808,0.161300589550352,
-0.851108899538562));
#62433=CARTESIAN_POINT('Ctrl Pts',(-0.756141466551346,0.237280652184228,
-0.854329924719685));
#62434=CARTESIAN_POINT('Ctrl Pts',(-0.677896883403394,0.487110997238635,
-0.864920990382615));
#62435=CARTESIAN_POINT('Ctrl Pts',(-0.463491730456965,0.692912716729475,
-0.875512056045544));
#62436=CARTESIAN_POINT('Ctrl Pts',(-0.210504529835239,0.763480763656139,
-0.886103121708472));
#62437=CARTESIAN_POINT('Ctrl Pts',(-0.0840109295243834,0.79876478711947,
-0.891398654539936));
#62438=CARTESIAN_POINT('Ctrl Pts',(0.0521281827052891,0.800240392441759,
-0.8966941873714));
#62439=CARTESIAN_POINT('Ctrl Pts',(0.18048173029882,0.769914110648867,-0.901989720202864));
#62440=CARTESIAN_POINT('Ctrl Pts',(0.308835277892352,0.739587828855975,
-0.907285253034329));
#62441=CARTESIAN_POINT('Ctrl Pts',(0.429403260849733,0.677459659947905,
-0.912580785865794));
#62442=CARTESIAN_POINT('Ctrl Pts',(0.527250424553959,0.590095959466128,
-0.917876318697259));
#62443=CARTESIAN_POINT('Ctrl Pts',(0.625097588258208,0.502732258984331,
-0.923171851528724));
#62444=CARTESIAN_POINT('Ctrl Pts',(0.700223932709283,0.390133026928822,
-0.928467384360189));
#62445=CARTESIAN_POINT('Ctrl Pts',(0.744738887959545,0.265929954895926,
-0.933762917191654));
#62446=CARTESIAN_POINT('Ctrl Pts',(0.789253843209797,0.141726882863057,
-0.939058450023118));
#62447=CARTESIAN_POINT('Ctrl Pts',(0.803157409259246,0.00591997085281483,
-0.944353982854583));
#62448=CARTESIAN_POINT('Ctrl Pts',(0.782330236569644,-0.123756747817209,
-0.949649515686047));
#62449=CARTESIAN_POINT('Ctrl Pts',(0.740675891190436,-0.383110185157272,
-0.960240581348976));
#62450=CARTESIAN_POINT('Ctrl Pts',(0.560098590854975,-0.617942849136481,
-0.970831647011908));
#62451=CARTESIAN_POINT('Ctrl Pts',(0.320395226075553,-0.724374344859862,
-0.981422712674837));
#62452=CARTESIAN_POINT('Ctrl Pts',(0.200543543685848,-0.777590092721549,
-0.986718245506301));
#62453=CARTESIAN_POINT('Ctrl Pts',(0.0659103451851567,-0.798705548519292,
-0.992013778337765));
#62454=CARTESIAN_POINT('Ctrl Pts',(-0.0657248991611227,-0.787797619310929,
-0.997309311169229));
#62455=CARTESIAN_POINT('Ctrl Pts',(-0.197360143507402,-0.776889690102566,
-1.00260484400069));
#62456=CARTESIAN_POINT('Ctrl Pts',(-0.325997433699261,-0.733958375888098,
-1.00790037683216));
#62457=CARTESIAN_POINT('Ctrl Pts',(-0.435288161250025,-0.661621833628534,
-1.01319590966362));
#62458=CARTESIAN_POINT('Ctrl Pts',(-0.651790257483054,-0.518325019851074,
-1.02368622283452));
#62459=CARTESIAN_POINT('Ctrl Pts',(-0.792371446149874,-0.259634498065135,
-1.03417653600542));
#62460=CARTESIAN_POINT('Ctrl Pts',(-0.792649648621414,-0.000247240842943735,
-1.04466684917632));
#62461=CARTESIAN_POINT('Ctrl Pts',(-0.791304392674353,0.000147799391554101,
-1.07313315082369));
#62462=CARTESIAN_POINT('Ctrl Pts',(-0.791133131450012,-0.121914689662786,
-1.06820650999216));
#62463=CARTESIAN_POINT('Ctrl Pts',(-0.761865101488357,-0.244166888435379,
-1.06327986916062));
#62464=CARTESIAN_POINT('Ctrl Pts',(-0.707132953686239,-0.353983585155056,
-1.05835322832909));
#62465=CARTESIAN_POINT('Ctrl Pts',(-0.648302627804268,-0.472023024766635,
-1.05305769549762));
#62466=CARTESIAN_POINT('Ctrl Pts',(-0.560052065294921,-0.575694976163254,
-1.04776216266616));
#62467=CARTESIAN_POINT('Ctrl Pts',(-0.451993647262742,-0.650320518196367,
-1.04246662983469));
#62468=CARTESIAN_POINT('Ctrl Pts',(-0.235876811198358,-0.799571602262608,
-1.03187556417176));
#62469=CARTESIAN_POINT('Ctrl Pts',(0.0594714469573586,-0.832637048874779,
-1.02128449850883));
#62470=CARTESIAN_POINT('Ctrl Pts',(0.301523172572088,-0.732895491692423,
-1.0106934328459));
#62471=CARTESIAN_POINT('Ctrl Pts',(0.54357489818679,-0.633153934510077,
-1.00010236718298));
#62472=CARTESIAN_POINT('Ctrl Pts',(0.732330091260526,-0.400605373533196,
-0.989511301520047));
#62473=CARTESIAN_POINT('Ctrl Pts',(0.779641955417371,-0.143021597759585,
-0.978920235857118));
#62474=CARTESIAN_POINT('Ctrl Pts',(0.826953819574218,0.114562178014041,
-0.968329170194189));
#62475=CARTESIAN_POINT('Ctrl Pts',(0.732822354814194,0.397181168584429,
-0.957738104531258));
#62476=CARTESIAN_POINT('Ctrl Pts',(0.542283414281508,0.577189685158702,
-0.947147038868329));
#62477=CARTESIAN_POINT('Ctrl Pts',(0.447013944015171,0.667193943445833,
-0.941851506036865));
#62478=CARTESIAN_POINT('Ctrl Pts',(0.327642604805676,0.731545583233934,
-0.936555973205402));
#62479=CARTESIAN_POINT('Ctrl Pts',(0.199826993358222,0.764862094816524,
-0.931260440373937));
#62480=CARTESIAN_POINT('Ctrl Pts',(0.072011381910739,0.798178606399122,
-0.925964907542472));
#62481=CARTESIAN_POINT('Ctrl Pts',(-0.0642485017746986,0.800459989776192,
-0.920669374711006));
#62482=CARTESIAN_POINT('Ctrl Pts',(-0.191449667115583,0.768582017317925,
-0.915373841879541));
#62483=CARTESIAN_POINT('Ctrl Pts',(-0.445851997797293,0.704826072401405,
-0.904782776216612));
#62484=CARTESIAN_POINT('Ctrl Pts',(-0.664019455100784,0.504432704143612,
-0.894191710553685));
#62485=CARTESIAN_POINT('Ctrl Pts',(-0.749525564601939,0.25606202313024,
-0.883600644890755));
#62486=CARTESIAN_POINT('Ctrl Pts',(-0.777695052683879,0.174237753735608,
-0.880111480201735));
#62487=CARTESIAN_POINT('Ctrl Pts',(-0.791466346747543,0.0872063409719881,
-0.876622315512715));
#62488=CARTESIAN_POINT('Ctrl Pts',(-0.791130549170082,0.000167441804084007,
-0.873133150823694));
#62489=CARTESIAN_POINT('Origin',(0.,0.,-5.925));
#62490=CARTESIAN_POINT('',(-0.790728689320429,-0.000203321923638479,-0.64466684917632));
#62491=CARTESIAN_POINT('',(-0.790791327823967,-2.33035369215209E-5,-0.673133150823699));
#62492=CARTESIAN_POINT('',(-0.7911,-9.68818082805471E-17,-5.925));
#62493=CARTESIAN_POINT('Ctrl Pts',(-0.7911,5.8164584260112E-13,-0.644666849176319));
#62494=CARTESIAN_POINT('Ctrl Pts',(-0.791099999999838,0.220167589667276,
-0.653525592749593));
#62495=CARTESIAN_POINT('Ctrl Pts',(-0.694214576672032,0.438610418339229,
-0.662384336322865));
#62496=CARTESIAN_POINT('Ctrl Pts',(-0.531017389079858,0.586395551223584,
-0.671243079896138));
#62497=CARTESIAN_POINT('Ctrl Pts',(-0.367820201487683,0.73418068410794,
-0.680101823469412));
#62498=CARTESIAN_POINT('Ctrl Pts',(-0.140868175871057,0.808992666571461,
-0.688960567042685));
#62499=CARTESIAN_POINT('Ctrl Pts',(0.0782205473254509,0.787223447298229,
-0.697819310615959));
#62500=CARTESIAN_POINT('Ctrl Pts',(0.297309270521959,0.765454228024996,
-0.706678054189232));
#62501=CARTESIAN_POINT('Ctrl Pts',(0.5051020726762,0.647444880833766,-0.715536797762506));
#62502=CARTESIAN_POINT('Ctrl Pts',(0.636026795762179,0.470435038100369,
-0.724395541335779));
#62503=CARTESIAN_POINT('Ctrl Pts',(0.766951518848158,0.293425195366972,
-0.733254284909053));
#62504=CARTESIAN_POINT('Ctrl Pts',(0.818956872247135,0.06018819600911,-0.742113028482325));
#62505=CARTESIAN_POINT('Ctrl Pts',(0.77563178100405,-0.155674501112047,
-0.750971772055598));
#62506=CARTESIAN_POINT('Ctrl Pts',(0.732306689760965,-0.371537198233204,
-0.759830515628871));
#62507=CARTESIAN_POINT('Ctrl Pts',(0.594329958849608,-0.56664351893714,
-0.768689259202145));
#62508=CARTESIAN_POINT('Ctrl Pts',(0.405242230243295,-0.679424716085189,
-0.777548002775418));
#62509=CARTESIAN_POINT('Ctrl Pts',(0.216154501636982,-0.792205913233239,
-0.786406746348692));
#62510=CARTESIAN_POINT('Ctrl Pts',(-0.0210816529309567,-0.820894963712984,
-0.795265489921966));
#62511=CARTESIAN_POINT('Ctrl Pts',(-0.2316027807541,-0.756438604215153,
-0.804124233495239));
#62512=CARTESIAN_POINT('Ctrl Pts',(-0.442123908577244,-0.691982244717321,
-0.812982977068512));
#62513=CARTESIAN_POINT('Ctrl Pts',(-0.622631625634828,-0.535390358802784,
-0.821841720641784));
#62514=CARTESIAN_POINT('Ctrl Pts',(-0.716163994722569,-0.336077881841415,
-0.830700464215058));
#62515=CARTESIAN_POINT('Ctrl Pts',(-0.765317280859706,-0.231334857513725,
-0.83535592586881));
#62516=CARTESIAN_POINT('Ctrl Pts',(-0.791100000000076,-0.115702837835854,
-0.840011387522564));
#62517=CARTESIAN_POINT('Ctrl Pts',(-0.7911,5.19639886675805E-13,-0.844666849176317));
#62518=CARTESIAN_POINT('Ctrl Pts',(-0.7911,-2.33146835171283E-15,-0.873133150823696));
#62519=CARTESIAN_POINT('Ctrl Pts',(-0.791099999999999,-0.220167589666667,
-0.864274407250424));
#62520=CARTESIAN_POINT('Ctrl Pts',(-0.694214576672381,-0.438610418338662,
-0.855415663677151));
#62521=CARTESIAN_POINT('Ctrl Pts',(-0.531017389080354,-0.586395551223135,
-0.846556920103879));
#62522=CARTESIAN_POINT('Ctrl Pts',(-0.367820201488326,-0.734180684107609,
-0.837698176530607));
#62523=CARTESIAN_POINT('Ctrl Pts',(-0.140868175871803,-0.808992666571323,
-0.828839432957334));
#62524=CARTESIAN_POINT('Ctrl Pts',(0.0782205473246955,-0.787223447298304,
-0.819980689384062));
#62525=CARTESIAN_POINT('Ctrl Pts',(0.297309270521194,-0.765454228025285,
-0.81112194581079));
#62526=CARTESIAN_POINT('Ctrl Pts',(0.505102072675523,-0.647444880834284,
-0.802263202237519));
#62527=CARTESIAN_POINT('Ctrl Pts',(0.636026795761674,-0.470435038101052,
-0.793404458664247));
#62528=CARTESIAN_POINT('Ctrl Pts',(0.766951518847825,-0.29342519536782,
-0.784545715090975));
#62529=CARTESIAN_POINT('Ctrl Pts',(0.818956872247058,-0.0601881960100528,
-0.775686971517702));
#62530=CARTESIAN_POINT('Ctrl Pts',(0.775631781004235,0.155674501111126,
-0.76682822794443));
#62531=CARTESIAN_POINT('Ctrl Pts',(0.732306689761412,0.371537198232305,
-0.757969484371158));
#62532=CARTESIAN_POINT('Ctrl Pts',(0.59432995885032,0.566643518936382,-0.749110740797887));
#62533=CARTESIAN_POINT('Ctrl Pts',(0.405242230244179,0.679424716084662,
-0.740251997224615));
#62534=CARTESIAN_POINT('Ctrl Pts',(0.216154501638038,0.792205913232943,
-0.731393253651343));
#62535=CARTESIAN_POINT('Ctrl Pts',(-0.0210816529298243,0.820894963713005,
-0.72253451007807));
#62536=CARTESIAN_POINT('Ctrl Pts',(-0.23160278075303,0.75643860421548,-0.713675766504798));
#62537=CARTESIAN_POINT('Ctrl Pts',(-0.442123908576237,0.691982244717956,
-0.704817022931526));
#62538=CARTESIAN_POINT('Ctrl Pts',(-0.622631625634022,0.535390358803709,
-0.695958279358253));
#62539=CARTESIAN_POINT('Ctrl Pts',(-0.716163994722056,0.336077881842509,
-0.687099535784981));
#62540=CARTESIAN_POINT('Ctrl Pts',(-0.765317280859448,0.231334857514691,
-0.682444074131219));
#62541=CARTESIAN_POINT('Ctrl Pts',(-0.791099999999998,0.115702837836613,
-0.677788612477458));
#62542=CARTESIAN_POINT('Ctrl Pts',(-0.7911,1.47104550762833E-14,-0.673133150823697));
#62543=CARTESIAN_POINT('Origin',(0.,0.,-5.925));
#62544=CARTESIAN_POINT('',(-0.791944510864312,-0.00022813924889703,-0.444666849176321));
#62545=CARTESIAN_POINT('',(-0.791972558534597,-0.000546350253884251,-0.473133150823699));
#62546=CARTESIAN_POINT('',(-0.7911,-9.68818082805471E-17,-5.925));
#62547=CARTESIAN_POINT('Ctrl Pts',(-0.791944510864312,-0.00022813924889703,
-0.444666849176321));
#62548=CARTESIAN_POINT('Ctrl Pts',(-0.791679905405434,0.103219919931978,
-0.448832886904162));
#62549=CARTESIAN_POINT('Ctrl Pts',(-0.770434409145543,0.206944064816135,
-0.452998924632003));
#62550=CARTESIAN_POINT('Ctrl Pts',(-0.730546028063464,0.302727261406224,
-0.457164962359844));
#62551=CARTESIAN_POINT('Ctrl Pts',(-0.679843119109353,0.424479174226344,
-0.462460495191308));
#62552=CARTESIAN_POINT('Ctrl Pts',(-0.599018054451231,0.533400536236713,
-0.467756028022773));
#62553=CARTESIAN_POINT('Ctrl Pts',(-0.496968020873342,0.61581579008526,
-0.473051560854237));
#62554=CARTESIAN_POINT('Ctrl Pts',(-0.394917987295454,0.698231043933806,
-0.478347093685701));
#62555=CARTESIAN_POINT('Ctrl Pts',(-0.271642984797799,0.75414018962053,
-0.483642626517165));
#62556=CARTESIAN_POINT('Ctrl Pts',(-0.141872253513096,0.777963364750619,
-0.488938159348629));
#62557=CARTESIAN_POINT('Ctrl Pts',(-0.0121015222283782,0.80178653988071,
-0.494233692180094));
#62558=CARTESIAN_POINT('Ctrl Pts',(0.124164937843389,0.793523744454159,
-0.499529225011559));
#62559=CARTESIAN_POINT('Ctrl Pts',(0.248760203786074,0.75198051656646,-0.504824757843024));
#62560=CARTESIAN_POINT('Ctrl Pts',(0.497950735671431,0.668894060791067,
-0.515415823505954));
#62561=CARTESIAN_POINT('Ctrl Pts',(0.700456491040463,0.452685875171097,
-0.526006889168883));
#62562=CARTESIAN_POINT('Ctrl Pts',(0.766683676846839,0.19891565103887,-0.536597954831812));
#62563=CARTESIAN_POINT('Ctrl Pts',(0.799797269750025,0.0720305389727643,
-0.541893487663276));
#62564=CARTESIAN_POINT('Ctrl Pts',(0.798841220262551,-0.0642450827214051,
-0.54718902049474));
#62565=CARTESIAN_POINT('Ctrl Pts',(0.76676938702351,-0.19237867589465,-0.552484553326204));
#62566=CARTESIAN_POINT('Ctrl Pts',(0.734697553784463,-0.320512269067924,
-0.55778008615767));
#62567=CARTESIAN_POINT('Ctrl Pts',(0.671509936793835,-0.440503833720271,
-0.563075618989136));
#62568=CARTESIAN_POINT('Ctrl Pts',(0.58243650440451,-0.536644159129025,
-0.568371151820601));
#62569=CARTESIAN_POINT('Ctrl Pts',(0.4042896396259,-0.728924809946489,-0.57896221748353));
#62570=CARTESIAN_POINT('Ctrl Pts',(0.122599513252553,-0.825800503789633,
-0.589553283146457));
#62571=CARTESIAN_POINT('Ctrl Pts',(-0.135432224195654,-0.780996074233637,
-0.600144348809386));
#62572=CARTESIAN_POINT('Ctrl Pts',(-0.393463961643877,-0.736191644677638,
-0.610735414472315));
#62573=CARTESIAN_POINT('Ctrl Pts',(-0.627837310166959,-0.549707091722483,
-0.621326480135245));
#62574=CARTESIAN_POINT('Ctrl Pts',(-0.729928286435418,-0.308636876853086,
-0.631917545798174));
#62575=CARTESIAN_POINT('Ctrl Pts',(-0.770893280580547,-0.211905115617681,
-0.63616731359089));
#62576=CARTESIAN_POINT('Ctrl Pts',(-0.79055957674958,-0.106384552767054,
-0.640417081383606));
#62577=CARTESIAN_POINT('Ctrl Pts',(-0.789917699687958,-0.00064740280164427,
-0.644666849176321));
#62578=CARTESIAN_POINT('Ctrl Pts',(-0.789692040475088,-0.000106295414249275,
-0.673133150823697));
#62579=CARTESIAN_POINT('Ctrl Pts',(-0.790252451913751,-0.0991149986681245,
-0.669151522538878));
#62580=CARTESIAN_POINT('Ctrl Pts',(-0.772988227439065,-0.198061641529546,
-0.665169894254059));
#62581=CARTESIAN_POINT('Ctrl Pts',(-0.737043873044512,-0.290039067860967,
-0.661188265969241));
#62582=CARTESIAN_POINT('Ctrl Pts',(-0.689238177689206,-0.412368287479148,
-0.655892733137777));
#62583=CARTESIAN_POINT('Ctrl Pts',(-0.608389609690481,-0.522369812631978,
-0.650597200306314));
#62584=CARTESIAN_POINT('Ctrl Pts',(-0.50704122135461,-0.60684755250419,
-0.64530166747485));
#62585=CARTESIAN_POINT('Ctrl Pts',(-0.405692833018717,-0.691325292376421,
-0.640006134643385));
#62586=CARTESIAN_POINT('Ctrl Pts',(-0.283844624345669,-0.750279246968022,
-0.63471060181192));
#62587=CARTESIAN_POINT('Ctrl Pts',(-0.155209837063072,-0.775961441139558,
-0.629415068980455));
#62588=CARTESIAN_POINT('Ctrl Pts',(-0.0265750497804897,-0.80164363531109,
-0.62411953614899));
#62589=CARTESIAN_POINT('Ctrl Pts',(0.10884631611164,-0.794054069062565,
-0.618824003317526));
#62590=CARTESIAN_POINT('Ctrl Pts',(0.234851914639674,-0.75510659557873,
-0.613528470486062));
#62591=CARTESIAN_POINT('Ctrl Pts',(0.360857513167722,-0.71615912209489,
-0.608232937654597));
#62592=CARTESIAN_POINT('Ctrl Pts',(0.477447344331671,-0.645853741375732,
-0.602937404823133));
#62593=CARTESIAN_POINT('Ctrl Pts',(0.568580117099377,-0.551299994986477,
-0.597641871991668));
#62594=CARTESIAN_POINT('Ctrl Pts',(0.750845662634779,-0.362192502207977,
-0.587050806328739));
#62595=CARTESIAN_POINT('Ctrl Pts',(0.83128297458522,-0.0760915467490993,
-0.576459740665809));
#62596=CARTESIAN_POINT('Ctrl Pts',(0.772037630551969,0.178913169173971,
-0.56586867500288));
#62597=CARTESIAN_POINT('Ctrl Pts',(0.712792286518719,0.433917885097042,
-0.55527760933995));
#62598=CARTESIAN_POINT('Ctrl Pts',(0.513864286501777,0.657826361484306,
-0.544686543677022));
#62599=CARTESIAN_POINT('Ctrl Pts',(0.267335844472759,0.746209288054612,
-0.534095478014093));
#62600=CARTESIAN_POINT('Ctrl Pts',(0.0208074024437416,0.834592214624919,
-0.523504412351164));
#62601=CARTESIAN_POINT('Ctrl Pts',(-0.273321481597352,0.787449591378269,
-0.512913346688235));
#62602=CARTESIAN_POINT('Ctrl Pts',(-0.481798547418916,0.628561369235547,
-0.502322281025305));
#62603=CARTESIAN_POINT('Ctrl Pts',(-0.586037080329692,0.54911725816419,
-0.497026748193841));
#62604=CARTESIAN_POINT('Ctrl Pts',(-0.668862658685588,0.441736747368818,
-0.491731215362376));
#62605=CARTESIAN_POINT('Ctrl Pts',(-0.722429270106406,0.320999684593171,
-0.486435682530912));
#62606=CARTESIAN_POINT('Ctrl Pts',(-0.767282896080836,0.219901352790059,
-0.482001505295174));
#62607=CARTESIAN_POINT('Ctrl Pts',(-0.79162179447004,0.10943816453247,-0.477567328059436));
#62608=CARTESIAN_POINT('Ctrl Pts',(-0.791972558534597,-0.000546350253884251,
-0.473133150823699));
#62609=CARTESIAN_POINT('Origin',(0.,0.,-5.925));
#62610=CARTESIAN_POINT('',(-0.7911,5.70765656959793E-13,-0.244666849176319));
#62611=CARTESIAN_POINT('',(-0.791468851257481,0.000547557155766596,-0.273133150823697));
#62612=CARTESIAN_POINT('',(-0.7911,-9.68818082805471E-17,-5.925));
#62613=CARTESIAN_POINT('Ctrl Pts',(-0.790957246177156,0.000419304332940074,
-0.244666849176318));
#62614=CARTESIAN_POINT('Ctrl Pts',(-0.791091484198145,0.0498428586940881,
-0.246657626761787));
#62615=CARTESIAN_POINT('Ctrl Pts',(-0.786624458151161,0.0992128624228036,
-0.248648404347256));
#62616=CARTESIAN_POINT('Ctrl Pts',(-0.777442989937871,0.147665862313506,
-0.250639181932724));
#62617=CARTESIAN_POINT('Ctrl Pts',(-0.753019987228064,0.276552410754211,
-0.255934714764189));
#62618=CARTESIAN_POINT('Ctrl Pts',(-0.695238665495522,0.398950448890937,
-0.261230247595654));
#62619=CARTESIAN_POINT('Ctrl Pts',(-0.611746352354572,0.501110679595837,
-0.266525780427119));
#62620=CARTESIAN_POINT('Ctrl Pts',(-0.528254039213631,0.603270910300727,
-0.271821313258583));
#62621=CARTESIAN_POINT('Ctrl Pts',(-0.419050734664292,0.68519333357379,
-0.277116846090047));
#62622=CARTESIAN_POINT('Ctrl Pts',(-0.297195225769133,0.734189991186984,
-0.282412378921512));
#62623=CARTESIAN_POINT('Ctrl Pts',(-0.0534842079788134,0.832183306413372,
-0.293003444584441));
#62624=CARTESIAN_POINT('Ctrl Pts',(0.240835627194766,0.798473559000276,
-0.303594510247369));
#62625=CARTESIAN_POINT('Ctrl Pts',(0.455592400909156,0.647924259310542,
-0.314185575910298));
#62626=CARTESIAN_POINT('Ctrl Pts',(0.562970787766375,0.572649609465658,
-0.319481108741763));
#62627=CARTESIAN_POINT('Ctrl Pts',(0.650458409258781,0.468165071551605,
-0.324776641573228));
#62628=CARTESIAN_POINT('Ctrl Pts',(0.708960624034482,0.349741654396658,
-0.330072174404694));
#62629=CARTESIAN_POINT('Ctrl Pts',(0.767462838810163,0.231318237241752,
-0.335367707236158));
#62630=CARTESIAN_POINT('Ctrl Pts',(0.79697964686916,0.0989559408459271,
-0.340663240067623));
#62631=CARTESIAN_POINT('Ctrl Pts',(0.791325851080046,-0.0319838013192029,
-0.345958772899087));
#62632=CARTESIAN_POINT('Ctrl Pts',(0.780018259501817,-0.293863285649508,
-0.356549838562016));
#62633=CARTESIAN_POINT('Ctrl Pts',(0.628028252531147,-0.55005255305717,
-0.367140904224945));
#62634=CARTESIAN_POINT('Ctrl Pts',(0.402354296443651,-0.682940171345567,
-0.377731969887874));
#62635=CARTESIAN_POINT('Ctrl Pts',(0.176680340356142,-0.815827789633971,
-0.388323035550804));
#62636=CARTESIAN_POINT('Ctrl Pts',(-0.122677564848187,-0.825413758803086,
-0.398914101213734));
#62637=CARTESIAN_POINT('Ctrl Pts',(-0.356547662793433,-0.707761206253896,
-0.409505166876663));
#62638=CARTESIAN_POINT('Ctrl Pts',(-0.590417760738652,-0.59010865370472,
-0.420096232539592));
#62639=CARTESIAN_POINT('Ctrl Pts',(-0.758800051424793,-0.345217579437281,
-0.43068729820252));
#62640=CARTESIAN_POINT('Ctrl Pts',(-0.78748647732005,-0.0841439365083014,
-0.441278363865449));
#62641=CARTESIAN_POINT('Ctrl Pts',(-0.790545770749094,-0.0563014690212264,
-0.442407858969073));
#62642=CARTESIAN_POINT('Ctrl Pts',(-0.79201625062994,-0.0282749511016459,
-0.443537354072697));
#62643=CARTESIAN_POINT('Ctrl Pts',(-0.791944510864312,-0.00022813924889703,
-0.444666849176321));
#62644=CARTESIAN_POINT('Ctrl Pts',(-0.791972558534597,-0.000546350253884251,
-0.473133150823699));
#62645=CARTESIAN_POINT('Ctrl Pts',(-0.792040695772629,-0.021911255673313,
-0.472271795227972));
#62646=CARTESIAN_POINT('Ctrl Pts',(-0.791203652207818,-0.0432580985777029,
-0.471410439632245));
#62647=CARTESIAN_POINT('Ctrl Pts',(-0.789435967515537,-0.0645147251750589,
-0.470549084036518));
#62648=CARTESIAN_POINT('Ctrl Pts',(-0.767700850520675,-0.325882189648303,
-0.459958018373589));
#62649=CARTESIAN_POINT('Ctrl Pts',(-0.605264921593145,-0.573610124044309,
-0.449366952710658));
#62650=CARTESIAN_POINT('Ctrl Pts',(-0.37401057509831,-0.698192255756164,
-0.438775887047729));
#62651=CARTESIAN_POINT('Ctrl Pts',(-0.258383401850899,-0.760483321612088,
-0.433480354216265));
#62652=CARTESIAN_POINT('Ctrl Pts',(-0.125551624211664,-0.791987936796978,
-0.428184821384802));
#62653=CARTESIAN_POINT('Ctrl Pts',(0.00638206399365039,-0.790767982704263,
-0.422889288553338));
#62654=CARTESIAN_POINT('Ctrl Pts',(0.138315752198995,-0.789548028611547,
-0.417593755721872));
#62655=CARTESIAN_POINT('Ctrl Pts',(0.269351350970419,-0.755603505241211,
-0.412298222890406));
#62656=CARTESIAN_POINT('Ctrl Pts',(0.384021022517093,-0.691906175253571,
-0.40700269005894));
#62657=CARTESIAN_POINT('Ctrl Pts',(0.498690694063741,-0.628208845265947,
-0.401707157227476));
#62658=CARTESIAN_POINT('Ctrl Pts',(0.596994438385647,-0.534758708661034,
-0.396411624396013));
#62659=CARTESIAN_POINT('Ctrl Pts',(0.667822021137814,-0.423503296328635,
-0.391116091564548));
#62660=CARTESIAN_POINT('Ctrl Pts',(0.738649603889981,-0.312247883996236,
-0.385820558733084));
#62661=CARTESIAN_POINT('Ctrl Pts',(0.782001025072408,-0.183187195936352,
-0.380525025901619));
#62662=CARTESIAN_POINT('Ctrl Pts',(0.790251999425748,-0.0521241922399114,
-0.375229493070155));
#62663=CARTESIAN_POINT('Ctrl Pts',(0.80675394813243,0.210001815152985,-0.364638427407225));
#62664=CARTESIAN_POINT('Ctrl Pts',(0.682854109522748,0.480137085092108,
-0.354047361744297));
#62665=CARTESIAN_POINT('Ctrl Pts',(0.472620005630473,0.636146595683167,
-0.343456296081368));
#62666=CARTESIAN_POINT('Ctrl Pts',(0.262385901738198,0.792156106274226,
-0.332865230418439));
#62667=CARTESIAN_POINT('Ctrl Pts',(-0.034182467436671,0.83403985751722,
-0.322274164755509));
#62668=CARTESIAN_POINT('Ctrl Pts',(-0.279299302753248,0.741814098670096,
-0.31168309909258));
#62669=CARTESIAN_POINT('Ctrl Pts',(-0.524416138069826,0.649588339822972,
-0.301092033429651));
#62670=CARTESIAN_POINT('Ctrl Pts',(-0.718081439528112,0.423253070885729,
-0.290500967766722));
#62671=CARTESIAN_POINT('Ctrl Pts',(-0.774123310097696,0.167190510788659,
-0.279909902103793));
#62672=CARTESIAN_POINT('Ctrl Pts',(-0.786076209211229,0.112576167682588,
-0.277650985010427));
#62673=CARTESIAN_POINT('Ctrl Pts',(-0.791768541684542,0.0566095135191815,
-0.275392067917062));
#62674=CARTESIAN_POINT('Ctrl Pts',(-0.791468851257481,0.000547557155766596,
-0.273133150823697));
#62675=CARTESIAN_POINT('Origin',(0.,0.,-5.925));
#62676=CARTESIAN_POINT('',(-0.7911,-9.68818082805471E-17,-0.0599999999999969));
#62677=CARTESIAN_POINT('',(-0.789664670674245,0.000390155355157968,-0.0731331508236992));
#62678=CARTESIAN_POINT('',(-0.7911,-9.68818082805471E-17,-5.925));
#62679=CARTESIAN_POINT('',(-0.701077753000047,0.366509473613445,-0.0599999999999987));
#62680=CARTESIAN_POINT('Origin',(0.,0.,-0.0599999999999996));
#62681=CARTESIAN_POINT('Ctrl Pts',(-0.701077753000086,0.366509473613371,
-0.0599999999999969));
#62682=CARTESIAN_POINT('Ctrl Pts',(-0.599076100370241,0.561623364457742,
-0.0688587435732708));
#62683=CARTESIAN_POINT('Ctrl Pts',(-0.41201304761304,0.710322621163273,
-0.0777174871465436));
#62684=CARTESIAN_POINT('Ctrl Pts',(-0.198919167149933,0.765682946747789,
-0.0865762307198175));
#62685=CARTESIAN_POINT('Ctrl Pts',(0.0141747133131744,0.821043272332304,
-0.0954349742930914));
#62686=CARTESIAN_POINT('Ctrl Pts',(0.249960728318654,0.782197297258215,
-0.104293717866366));
#62687=CARTESIAN_POINT('Ctrl Pts',(0.434033038607528,0.661403455840016,
-0.11315246143964));
#62688=CARTESIAN_POINT('Ctrl Pts',(0.618105348896402,0.540609614421817,
-0.122011205012914));
#62689=CARTESIAN_POINT('Ctrl Pts',(0.747579962856046,0.339760469560251,
-0.130869948586188));
#62690=CARTESIAN_POINT('Ctrl Pts',(0.781599209966111,0.12223700331876,-0.139728692159462));
#62691=CARTESIAN_POINT('Ctrl Pts',(0.815618457076177,-0.0952864629227309,
-0.148587435732736));
#62692=CARTESIAN_POINT('Ctrl Pts',(0.753649333631875,-0.32607615591435,
-0.157446179306009));
#62693=CARTESIAN_POINT('Ctrl Pts',(0.615247132757394,-0.497302901292367,
-0.166304922879283));
#62694=CARTESIAN_POINT('Ctrl Pts',(0.476844931882912,-0.668529646670385,
-0.175163666452556));
#62695=CARTESIAN_POINT('Ctrl Pts',(0.264178099151975,-0.777510713410496,
-0.184022410025831));
#62696=CARTESIAN_POINT('Ctrl Pts',(0.0443568665752726,-0.789855479431284,
-0.192881153599105));
#62697=CARTESIAN_POINT('Ctrl Pts',(-0.17546436600143,-0.802200245452072,
-0.201739897172379));
#62698=CARTESIAN_POINT('Ctrl Pts',(-0.398995903057064,-0.717715296537093,
-0.210598640745653));
#62699=CARTESIAN_POINT('Ctrl Pts',(-0.555698990988761,-0.563061134703926,
-0.219457384318927));
#62700=CARTESIAN_POINT('Ctrl Pts',(-0.70434313206,-0.416360547292378,-0.227860539271391));
#62701=CARTESIAN_POINT('Ctrl Pts',(-0.791100000000151,-0.20884478212649,
-0.236263694223855));
#62702=CARTESIAN_POINT('Ctrl Pts',(-0.7911,5.70765656959793E-13,-0.244666849176319));
#62703=CARTESIAN_POINT('Ctrl Pts',(-0.791468851257481,0.000547557155766596,
-0.273133150823697));
#62704=CARTESIAN_POINT('Ctrl Pts',(-0.791065983586929,-0.074815376482576,
-0.270096535085597));
#62705=CARTESIAN_POINT('Ctrl Pts',(-0.779835008433342,-0.150350529500286,
-0.267059919347497));
#62706=CARTESIAN_POINT('Ctrl Pts',(-0.758428280312644,-0.223004338239144,
-0.264023303609398));
#62707=CARTESIAN_POINT('Ctrl Pts',(-0.721097237680188,-0.34970480437989,
-0.258727770777933));
#62708=CARTESIAN_POINT('Ctrl Pts',(-0.652820074852665,-0.467642633822896,
-0.253432237946469));
#62709=CARTESIAN_POINT('Ctrl Pts',(-0.559938392265368,-0.560213600724365,
-0.248136705115005));
#62710=CARTESIAN_POINT('Ctrl Pts',(-0.374175027090764,-0.745355534527313,
-0.237545639452076));
#62711=CARTESIAN_POINT('Ctrl Pts',(-0.089993582877054,-0.829030018164101,
-0.226954573789146));
#62712=CARTESIAN_POINT('Ctrl Pts',(0.166910245748897,-0.774274444394978,
-0.216363508126217));
#62713=CARTESIAN_POINT('Ctrl Pts',(0.29536216006188,-0.746896657510415,
-0.211067975294752));
#62714=CARTESIAN_POINT('Ctrl Pts',(0.416994670477923,-0.68491135627437,
-0.205772442463288));
#62715=CARTESIAN_POINT('Ctrl Pts',(0.516766904098013,-0.598579551649639,
-0.200476909631823));
#62716=CARTESIAN_POINT('Ctrl Pts',(0.616539137718092,-0.512247747024917,
-0.195181376800359));
#62717=CARTESIAN_POINT('Ctrl Pts',(0.694451094542224,-0.401569439011514,
-0.189885843968895));
#62718=CARTESIAN_POINT('Ctrl Pts',(0.740611247050816,-0.278779106530895,
-0.184590311137431));
#62719=CARTESIAN_POINT('Ctrl Pts',(0.786771399559408,-0.155988774050276,
-0.179294778305966));
#62720=CARTESIAN_POINT('Ctrl Pts',(0.801179747752459,-0.0210864171024406,
-0.173999245474501));
#62721=CARTESIAN_POINT('Ctrl Pts',(0.783148445581123,0.109551658983387,
-0.168703712643037));
#62722=CARTESIAN_POINT('Ctrl Pts',(0.765117143409784,0.24018973506923,-0.163408179811572));
#62723=CARTESIAN_POINT('Ctrl Pts',(0.71464619087405,0.366563530293064,-0.158112646980107));
#62724=CARTESIAN_POINT('Ctrl Pts',(0.636094778853461,0.471793541056986,
-0.152817114148643));
#62725=CARTESIAN_POINT('Ctrl Pts',(0.478991954812292,0.682253562584816,
-0.142226048485714));
#62726=CARTESIAN_POINT('Ctrl Pts',(0.209567292831717,0.808138446273004,
-0.131634982822784));
#62727=CARTESIAN_POINT('Ctrl Pts',(-0.0516326420874012,0.790898324967994,
-0.121043917159855));
#62728=CARTESIAN_POINT('Ctrl Pts',(-0.312832577006519,0.773658203662983,
-0.110452851496926));
#62729=CARTESIAN_POINT('Ctrl Pts',(-0.565807784864179,0.613293077364774,
-0.0998617858339976));
#62730=CARTESIAN_POINT('Ctrl Pts',(-0.693025188183458,0.384481595935094,
-0.0892707201710682));
#62731=CARTESIAN_POINT('Ctrl Pts',(-0.757638757569675,0.268268513872607,
-0.083891530388612));
#62732=CARTESIAN_POINT('Ctrl Pts',(-0.789811691001155,0.134398926932358,
-0.0785123406061555));
#62733=CARTESIAN_POINT('Ctrl Pts',(-0.789664670674245,0.000390155355157968,
-0.0731331508236992));
#62734=CARTESIAN_POINT('Origin',(0.,0.,-12.278617978381));
#62735=CARTESIAN_POINT('',(-0.6767,5.98871479897751E-13,-0.17861797838103));
#62736=CARTESIAN_POINT('',(-0.675472231886313,0.000333735468832419,-0.139182021619022));
#62737=CARTESIAN_POINT('',(-0.6767,6.12423655037739E-13,-12.278617978381));
#62738=CARTESIAN_POINT('',(0.564209944071435,0.373617490236885,-0.0599999999999987));
#62739=CARTESIAN_POINT('Ctrl Pts',(-0.6767,5.98871479897751E-13,-0.17861797838103));
#62740=CARTESIAN_POINT('Ctrl Pts',(-0.67670000000009,-0.10198549600935,
-0.173820728251383));
#62741=CARTESIAN_POINT('Ctrl Pts',(-0.653245593890205,-0.203961661393933,
-0.169020603322871));
#62742=CARTESIAN_POINT('Ctrl Pts',(-0.608664118325269,-0.295720951343193,
-0.164221915793792));
#62743=CARTESIAN_POINT('Ctrl Pts',(-0.523085967092649,-0.471861159641993,
-0.155010403570885));
#62744=CARTESIAN_POINT('Ctrl Pts',(-0.357381681450831,-0.607083368831098,
-0.145798891347978));
#62745=CARTESIAN_POINT('Ctrl Pts',(-0.167658291688701,-0.65560169861588,
-0.136587379125071));
#62746=CARTESIAN_POINT('Ctrl Pts',(0.0220650980734294,-0.704120028400661,
-0.127375866902165));
#62747=CARTESIAN_POINT('Ctrl Pts',(0.232341935463792,-0.665048199736589,
-0.118164354679259));
#62748=CARTESIAN_POINT('Ctrl Pts',(0.391973042749502,-0.55161582986504,
-0.108952842456352));
#62749=CARTESIAN_POINT('Ctrl Pts',(0.551604150035213,-0.438183459993492,
-0.0997413302334453));
#62750=CARTESIAN_POINT('Ctrl Pts',(0.657673563169899,-0.252462605657446,
-0.0905298180105381));
#62751=CARTESIAN_POINT('Ctrl Pts',(0.674266461046662,-0.0573378540548125,
-0.0813183057876312));
#62752=CARTESIAN_POINT('Ctrl Pts',(0.687066837440891,0.0931886111168982,
-0.0742122038584208));
#62753=CARTESIAN_POINT('Ctrl Pts',(0.647618097050576,0.247660567562773,
-0.0671061019292091));
#62754=CARTESIAN_POINT('Ctrl Pts',(0.564209944071435,0.373617490236885,
-0.0599999999999987));
#62755=CARTESIAN_POINT('',(0.537060862935828,-0.411689834101626,-0.0599999999999987));
#62756=CARTESIAN_POINT('Origin',(0.,0.,-0.0599999999999987));
#62757=CARTESIAN_POINT('Ctrl Pts',(-0.675472231886313,0.000333735468832488,
-0.139182021619022));
#62758=CARTESIAN_POINT('Ctrl Pts',(-0.67535038361465,-0.110730751752114,
-0.133970145738539));
#62759=CARTESIAN_POINT('Ctrl Pts',(-0.622781870731608,-0.33486777276979,
-0.123462737026592));
#62760=CARTESIAN_POINT('Ctrl Pts',(-0.385645525478233,-0.58933640490133,
-0.107659795483182));
#62761=CARTESIAN_POINT('Ctrl Pts',(-0.0580733210265062,-0.703415543027182,
-0.0917731969887855));
#62762=CARTESIAN_POINT('Ctrl Pts',(0.286592368567594,-0.644628272737791,
-0.0758865984943943));
#62763=CARTESIAN_POINT('Ctrl Pts',(0.468570466391673,-0.501037465313089,
-0.065295532831463));
#62764=CARTESIAN_POINT('Ctrl Pts',(0.537060862935828,-0.411689834101626,
-0.0599999999999987));
#62765=CARTESIAN_POINT('Origin',(0.,0.,-12.278617978381));
#62766=CARTESIAN_POINT('',(-0.67742238718478,-0.000195148311967771,-0.378617978381031));
#62767=CARTESIAN_POINT('',(-0.677015512129869,0.000468375588248721,-0.33918202161902));
#62768=CARTESIAN_POINT('',(-0.6767,6.12423655037739E-13,-12.278617978381));
#62769=CARTESIAN_POINT('Ctrl Pts',(-0.67742238718478,-0.000195148311967774,
-0.378617978381031));
#62770=CARTESIAN_POINT('Ctrl Pts',(-0.677483752750961,-0.0241861451275098,
-0.377488483277405));
#62771=CARTESIAN_POINT('Ctrl Pts',(-0.664431426608646,-0.272956126468997,
-0.365767922510851));
#62772=CARTESIAN_POINT('Ctrl Pts',(-0.361005438736672,-0.714251442192837,
-0.343456296081368));
#62773=CARTESIAN_POINT('Ctrl Pts',(0.407198939161548,-0.689652180392618,
-0.311683099092581));
#62774=CARTESIAN_POINT('Ctrl Pts',(0.732226235701414,-0.141797050653159,
-0.285205434935257));
#62775=CARTESIAN_POINT('Ctrl Pts',(0.631232561002846,0.311089138051407,
-0.264023303609399));
#62776=CARTESIAN_POINT('Ctrl Pts',(0.331887985278457,0.668589766575936,
-0.242841172283542));
#62777=CARTESIAN_POINT('Ctrl Pts',(-0.17162922483904,0.726259811006413,
-0.221659040957683));
#62778=CARTESIAN_POINT('Ctrl Pts',(-0.545275419699615,0.445956922224332,
-0.200476909631823));
#62779=CARTESIAN_POINT('Ctrl Pts',(-0.662707531036891,0.197200756547418,
-0.187895066383429));
#62780=CARTESIAN_POINT('Ctrl Pts',(-0.676692715657785,0.0426351440758945,
-0.180608755966498));
#62781=CARTESIAN_POINT('Ctrl Pts',(-0.676577889632261,0.000358669248252046,
-0.178617978381032));
#62782=CARTESIAN_POINT('Ctrl Pts',(-0.677015512129869,0.000468375588248721,
-0.33918202161902));
#62783=CARTESIAN_POINT('Ctrl Pts',(-0.676670902658741,-0.0639964167176895,
-0.33614540588091));
#62784=CARTESIAN_POINT('Ctrl Pts',(-0.650310658710815,-0.241285123438995,
-0.327813257311336));
#62785=CARTESIAN_POINT('Ctrl Pts',(-0.441609192873322,-0.601783375902012,
-0.308890043078835));
#62786=CARTESIAN_POINT('Ctrl Pts',(0.0445634358699717,-0.744932214423158,
-0.287707911752975));
#62787=CARTESIAN_POINT('Ctrl Pts',(0.460736965378437,-0.532845482801779,
-0.266525780427117));
#62788=CARTESIAN_POINT('Ctrl Pts',(0.660672578510412,-0.248825721585754,
-0.250639181932725));
#62789=CARTESIAN_POINT('Ctrl Pts',(0.697646902447653,0.0973571564825142,
-0.234752583438329));
#62790=CARTESIAN_POINT('Ctrl Pts',(0.524957262296379,0.529753299715826,
-0.213570452112473));
#62791=CARTESIAN_POINT('Ctrl Pts',(-0.0512014684653643,0.798955362640304,
-0.187092787955149));
#62792=CARTESIAN_POINT('Ctrl Pts',(-0.593892650520787,0.454934536693656,
-0.160531466846845));
#62793=CARTESIAN_POINT('Ctrl Pts',(-0.675597991784087,0.114963663071067,
-0.144561211401469));
#62794=CARTESIAN_POINT('Ctrl Pts',(-0.675472231886313,0.000333735468832488,
-0.139182021619022));
#62795=CARTESIAN_POINT('Origin',(0.,0.,-12.278617978381));
#62796=CARTESIAN_POINT('',(-0.67666270498899,-2.04219635818603E-5,-0.578617978381031));
#62797=CARTESIAN_POINT('',(-0.67744637891589,-0.00046734321359837,-0.539182021619019));
#62798=CARTESIAN_POINT('',(-0.6767,6.12423655037739E-13,-12.278617978381));
#62799=CARTESIAN_POINT('Ctrl Pts',(-0.675688670684921,-0.000553782676958534,
-0.578617978381031));
#62800=CARTESIAN_POINT('Ctrl Pts',(-0.676237726692527,-0.0910004131681901,
-0.574368210588314));
#62801=CARTESIAN_POINT('Ctrl Pts',(-0.617491434940766,-0.406206780333588,
-0.559527377132667));
#62802=CARTESIAN_POINT('Ctrl Pts',(-0.136084714826095,-0.789249125190363,
-0.534095478014092));
#62803=CARTESIAN_POINT('Ctrl Pts',(0.466303442539805,-0.582082578534946,
-0.50761781385677));
#62804=CARTESIAN_POINT('Ctrl Pts',(0.682503975557423,-0.171523651470232,
-0.486435682530911));
#62805=CARTESIAN_POINT('Ctrl Pts',(0.685775160935683,0.294752233755149,
-0.465253551205053));
#62806=CARTESIAN_POINT('Ctrl Pts',(0.339331867652397,0.664637404300089,
-0.444071419879196));
#62807=CARTESIAN_POINT('Ctrl Pts',(-0.126912670487204,0.692909095187001,
-0.422889288553336));
#62808=CARTESIAN_POINT('Ctrl Pts',(-0.443257737571659,0.549436516930662,
-0.407002690058943));
#62809=CARTESIAN_POINT('Ctrl Pts',(-0.635922507310959,0.289797886016136,
-0.392245586668175));
#62810=CARTESIAN_POINT('Ctrl Pts',(-0.677196045996511,0.0882934140033878,
-0.38278401610887));
#62811=CARTESIAN_POINT('Ctrl Pts',(-0.67742238718478,-0.000195148311967774,
-0.378617978381031));
#62812=CARTESIAN_POINT('Ctrl Pts',(-0.67744637891589,-0.000467343213598401,
-0.539182021619019));
#62813=CARTESIAN_POINT('Ctrl Pts',(-0.677504662911581,-0.018742695883905,
-0.538320666023284));
#62814=CARTESIAN_POINT('Ctrl Pts',(-0.667984865883078,-0.261522904938053,
-0.526868244764619));
#62815=CARTESIAN_POINT('Ctrl Pts',(-0.448265169876774,-0.596613218990799,
-0.510120290674488));
#62816=CARTESIAN_POINT('Ctrl Pts',(0.00622737937602623,-0.704408304798551,
-0.488938159348631));
#62817=CARTESIAN_POINT('Ctrl Pts',(0.342487484376452,-0.61730076227034,
-0.473051560854236));
#62818=CARTESIAN_POINT('Ctrl Pts',(0.594751965918543,-0.377491481115471,
-0.457164962359842));
#62819=CARTESIAN_POINT('Ctrl Pts',(0.743081667418538,0.0640980403615866,
-0.435982831033984));
#62820=CARTESIAN_POINT('Ctrl Pts',(0.478124579859611,0.641776390658052,
-0.409505166876661));
#62821=CARTESIAN_POINT('Ctrl Pts',(-0.282921364094237,0.749257370810349,
-0.377731969887874));
#62822=CARTESIAN_POINT('Ctrl Pts',(-0.649573297565699,0.320753847754227,
-0.354290921468661));
#62823=CARTESIAN_POINT('Ctrl Pts',(-0.677271864692064,0.0484232812524634,
-0.341440938712375));
#62824=CARTESIAN_POINT('Ctrl Pts',(-0.677015512129869,0.000468375588248721,
-0.33918202161902));
#62825=CARTESIAN_POINT('Origin',(0.,0.,-12.278617978381));
#62826=CARTESIAN_POINT('',(-0.6767,5.55100064568364E-13,-0.778617978381028));
#62827=CARTESIAN_POINT('',(-0.676541475852966,-1.19679499782825E-5,-0.73918202161902));
#62828=CARTESIAN_POINT('',(-0.6767,6.12423655037739E-13,-12.278617978381));
#62829=CARTESIAN_POINT('Ctrl Pts',(-0.6767,5.55100064568364E-13,-0.778617978381028));
#62830=CARTESIAN_POINT('Ctrl Pts',(-0.676700000000037,-0.0455605697071119,
-0.776474875121369));
#62831=CARTESIAN_POINT('Ctrl Pts',(-0.672073181934436,-0.0912183166350835,
-0.774327141130771));
#62832=CARTESIAN_POINT('Ctrl Pts',(-0.662913553532106,-0.135898898242169,
-0.772181722505643));
#62833=CARTESIAN_POINT('Ctrl Pts',(-0.623586017172946,-0.327738252473403,
-0.762970210282736));
#62834=CARTESIAN_POINT('Ctrl Pts',(-0.496498716511246,-0.499760850258025,
-0.75375869805983));
#62835=CARTESIAN_POINT('Ctrl Pts',(-0.324683073455861,-0.593720297624442,
-0.744547185836923));
#62836=CARTESIAN_POINT('Ctrl Pts',(-0.152867430400476,-0.68767974499086,
-0.735335673614017));
#62837=CARTESIAN_POINT('Ctrl Pts',(0.0605380174147123,-0.70185969495009,
-0.726124161391109));
#62838=CARTESIAN_POINT('Ctrl Pts',(0.243274753090137,-0.631458854169401,
-0.716912649168203));
#62839=CARTESIAN_POINT('Ctrl Pts',(0.426011488765561,-0.561058013388712,
-0.707701136945296));
#62840=CARTESIAN_POINT('Ctrl Pts',(0.574741480258209,-0.407362386357087,
-0.698489624722388));
#62841=CARTESIAN_POINT('Ctrl Pts',(0.639105148120741,-0.222412903505094,
-0.689278112499482));
#62842=CARTESIAN_POINT('Ctrl Pts',(0.703468815983272,-0.037463420653101,
-0.680066600276575));
#62843=CARTESIAN_POINT('Ctrl Pts',(0.682290436106702,0.175361465964632,
-0.670855088053667));
#62844=CARTESIAN_POINT('Ctrl Pts',(0.582740951575584,0.343999815925508,
-0.661643575830761));
#62845=CARTESIAN_POINT('Ctrl Pts',(0.483191467044466,0.512638165886383,
-0.652432063607854));
#62846=CARTESIAN_POINT('Ctrl Pts',(0.307089337447684,0.634009480823339,
-0.643220551384948));
#62847=CARTESIAN_POINT('Ctrl Pts',(0.114062275375495,0.667017756387463,
-0.634009039162041));
#62848=CARTESIAN_POINT('Ctrl Pts',(-0.0789647866966941,0.700026031951587,
-0.624797526939135));
#62849=CARTESIAN_POINT('Ctrl Pts',(-0.28539077693003,0.644068309569111,
-0.615586014716227));
#62850=CARTESIAN_POINT('Ctrl Pts',(-0.435320404194442,0.518091725172278,
-0.60637450249332));
#62851=CARTESIAN_POINT('Ctrl Pts',(-0.585250031458855,0.392115140775446,
-0.597162990270414));
#62852=CARTESIAN_POINT('Ctrl Pts',(-0.675944547586627,0.198420894907385,
-0.587951478047506));
#62853=CARTESIAN_POINT('Ctrl Pts',(-0.676695030694978,0.00259334392683,
-0.5787399658246));
#62854=CARTESIAN_POINT('Ctrl Pts',(-0.676698343560937,0.0017289001834459,
-0.57869930334341));
#62855=CARTESIAN_POINT('Ctrl Pts',(-0.676699999999999,0.000864381983809313,
-0.578658637658509));
#62856=CARTESIAN_POINT('Ctrl Pts',(-0.6767,6.08156477887935E-13,-0.578617978381031));
#62857=CARTESIAN_POINT('Ctrl Pts',(-0.675495643773846,-9.09241642347361E-5,
-0.739182021619016));
#62858=CARTESIAN_POINT('Ctrl Pts',(-0.675975014802293,-0.0847821003644994,
-0.735200393334189));
#62859=CARTESIAN_POINT('Ctrl Pts',(-0.641566474247868,-0.281988153762673,
-0.725923232217898));
#62860=CARTESIAN_POINT('Ctrl Pts',(-0.451253979159214,-0.540924894803379,
-0.711350538270144));
#62861=CARTESIAN_POINT('Ctrl Pts',(-0.138570312837484,-0.69221098153884,
-0.695463939775748));
#62862=CARTESIAN_POINT('Ctrl Pts',(0.208944432324475,-0.672734836372497,
-0.679577341281356));
#62863=CARTESIAN_POINT('Ctrl Pts',(0.607864107453516,-0.432180412746452,
-0.658395209955497));
#62864=CARTESIAN_POINT('Ctrl Pts',(0.77987753494969,0.179640205882728,-0.631917545798173));
#62865=CARTESIAN_POINT('Ctrl Pts',(0.269393736650696,0.754228245212569,
-0.600144348809387));
#62866=CARTESIAN_POINT('Ctrl Pts',(-0.359594431187155,0.653414779307557,
-0.573666684652064));
#62867=CARTESIAN_POINT('Ctrl Pts',(-0.631463554648116,0.300945820729597,
-0.553345908921941));
#62868=CARTESIAN_POINT('Ctrl Pts',(-0.677146338412084,0.093612445884841,
-0.543616198854748));
#62869=CARTESIAN_POINT('Ctrl Pts',(-0.67744637891589,-0.000467343213598401,
-0.539182021619019));
#62870=CARTESIAN_POINT('Origin',(0.,0.,-12.278617978381));
#62871=CARTESIAN_POINT('',(-0.678025555836318,-0.000211487647944881,-0.978617978381028));
#62872=CARTESIAN_POINT('',(-0.6767,5.52151526765261E-13,-0.939182021619017));
#62873=CARTESIAN_POINT('',(-0.6767,6.12423655037739E-13,-12.278617978381));
#62874=CARTESIAN_POINT('Ctrl Pts',(-0.678025555836318,-0.00021148764794485,
-0.978617978381028));
#62875=CARTESIAN_POINT('Ctrl Pts',(-0.677787583882777,-0.222089071976444,
-0.968127665210128));
#62876=CARTESIAN_POINT('Ctrl Pts',(-0.496832240698866,-0.555074107827601,
-0.952341819207762));
#62877=CARTESIAN_POINT('Ctrl Pts',(-0.0587849258484244,-0.701267695135047,
-0.931260440373935));
#62878=CARTESIAN_POINT('Ctrl Pts',(0.401871301811429,-0.629019792526908,
-0.910078309048076));
#62879=CARTESIAN_POINT('Ctrl Pts',(0.710799778962247,-0.227272191175134,
-0.888896177722219));
#62880=CARTESIAN_POINT('Ctrl Pts',(0.663227825248934,0.237399973442935,
-0.867714046396359));
#62881=CARTESIAN_POINT('Ctrl Pts',(0.470440577277662,0.526349159381354,
-0.851827447901968));
#62882=CARTESIAN_POINT('Ctrl Pts',(0.16104219249472,0.685780831357495,-0.83594084940757));
#62883=CARTESIAN_POINT('Ctrl Pts',(-0.304766616737118,0.680731951966365,
-0.814758718081714));
#62884=CARTESIAN_POINT('Ctrl Pts',(-0.635643959619811,0.363131720955057,
-0.795651094406201));
#62885=CARTESIAN_POINT('Ctrl Pts',(-0.676734292027046,0.0694989861940519,
-0.781839003562151));
#62886=CARTESIAN_POINT('Ctrl Pts',(-0.676179486370995,0.000828682045256053,
-0.77861797838103));
#62887=CARTESIAN_POINT('Ctrl Pts',(-0.6767,5.52151526765261E-13,-0.939182021619017));
#62888=CARTESIAN_POINT('Ctrl Pts',(-0.676700000000007,-0.00844923571080296,
-0.938784581799655));
#62889=CARTESIAN_POINT('Ctrl Pts',(-0.676541534771158,-0.0169092373903444,
-0.93838663555165));
#62890=CARTESIAN_POINT('Ctrl Pts',(-0.676224715602058,-0.0253579180714143,
-0.937988942517967));
#62891=CARTESIAN_POINT('Ctrl Pts',(-0.668886433556761,-0.221049365417898,
-0.92877743029506));
#62892=CARTESIAN_POINT('Ctrl Pts',(-0.571726805262928,-0.411582729340996,
-0.919565918072152));
#62893=CARTESIAN_POINT('Ctrl Pts',(-0.417643822383386,-0.532443919699525,
-0.910354405849246));
#62894=CARTESIAN_POINT('Ctrl Pts',(-0.263560839503844,-0.653305110058055,
-0.901142893626339));
#62895=CARTESIAN_POINT('Ctrl Pts',(-0.0553691191008583,-0.702286368654506,
-0.891931381403432));
#62896=CARTESIAN_POINT('Ctrl Pts',(0.136438176157497,-0.662802771634832,
-0.882719869180525));
#62897=CARTESIAN_POINT('Ctrl Pts',(0.328245471415853,-0.623319174615159,
-0.873508356957618));
#62898=CARTESIAN_POINT('Ctrl Pts',(0.500164618562822,-0.496091964544725,
-0.864296844734711));
#62899=CARTESIAN_POINT('Ctrl Pts',(0.593984251737507,-0.32419993628598,
-0.855085332511804));
#62900=CARTESIAN_POINT('Ctrl Pts',(0.687803884912193,-0.152307908027235,
-0.845873820288897));
#62901=CARTESIAN_POINT('Ctrl Pts',(0.701810211096223,0.0611090054657547,
-0.836662308065991));
#62902=CARTESIAN_POINT('Ctrl Pts',(0.631260725505247,0.243788405045419,
-0.827450795843085));
#62903=CARTESIAN_POINT('Ctrl Pts',(0.560711239914272,0.426467804625083,
-0.818239283620178));
#62904=CARTESIAN_POINT('Ctrl Pts',(0.406894662315832,0.575072705600625,
-0.80902777139727));
#62905=CARTESIAN_POINT('Ctrl Pts',(0.221892876680649,0.639285883841014,
-0.799816259174364));
#62906=CARTESIAN_POINT('Ctrl Pts',(0.036891091045467,0.703499062081403,
-0.790604746951457));
#62907=CARTESIAN_POINT('Ctrl Pts',(-0.175916495162588,0.682147542455185,
-0.781393234728549));
#62908=CARTESIAN_POINT('Ctrl Pts',(-0.344473799393609,0.582460892705538,
-0.772181722505643));
#62909=CARTESIAN_POINT('Ctrl Pts',(-0.51303110362463,0.48277424295589,-0.762970210282736));
#62910=CARTESIAN_POINT('Ctrl Pts',(-0.634259107965074,0.306573428253798,
-0.753758698059829));
#62911=CARTESIAN_POINT('Ctrl Pts',(-0.667110332652752,0.113519575703642,
-0.744547185836922));
#62912=CARTESIAN_POINT('Ctrl Pts',(-0.673488301544418,0.0760387366272504,
-0.742758797764287));
#62913=CARTESIAN_POINT('Ctrl Pts',(-0.676699999999968,0.0379746730511501,
-0.740968295278925));
#62914=CARTESIAN_POINT('Ctrl Pts',(-0.6767,5.66741998541723E-13,-0.739182021619017));
#62915=CARTESIAN_POINT('Origin',(0.,0.,-12.278617978381));
#62916=CARTESIAN_POINT('',(-0.675858962494509,-0.000507684201011625,-1.17861797838103));
#62917=CARTESIAN_POINT('',(-0.676874835700589,0.000126426303653261,-1.13918202161902));
#62918=CARTESIAN_POINT('',(-0.6767,6.12423655037739E-13,-12.278617978381));
#62919=CARTESIAN_POINT('Ctrl Pts',(-0.675858962494509,-0.000507684201011542,
-1.17861797838103));
#62920=CARTESIAN_POINT('Ctrl Pts',(-0.676345794384335,-0.0647735879750859,
-1.17559845818397));
#62921=CARTESIAN_POINT('Ctrl Pts',(-0.653229074319601,-0.241425877431507,
-1.16728340515544));
#62922=CARTESIAN_POINT('Ctrl Pts',(-0.498772672191106,-0.496445232852937,
-1.15367281929545));
#62923=CARTESIAN_POINT('Ctrl Pts',(-0.100894871170555,-0.739585470098981,
-1.13249068796959));
#62924=CARTESIAN_POINT('Ctrl Pts',(0.394639860164164,-0.633362736055885,
-1.11130855664373));
#62925=CARTESIAN_POINT('Ctrl Pts',(0.659187605562879,-0.248398060071516,
-1.09012642531787));
#62926=CARTESIAN_POINT('Ctrl Pts',(0.699298891271897,0.0966376479255593,
-1.07423982682348));
#62927=CARTESIAN_POINT('Ctrl Pts',(0.566686762943658,0.418444798182639,
-1.05835322832909));
#62928=CARTESIAN_POINT('Ctrl Pts',(0.208383162066687,0.716139049954344,
-1.03717109700323));
#62929=CARTESIAN_POINT('Ctrl Pts',(-0.425983270133073,0.677508544252163,
-1.0106934328459));
#62930=CARTESIAN_POINT('Ctrl Pts',(-0.677095589286557,0.228064891222822,
-0.989410549028017));
#62931=CARTESIAN_POINT('Ctrl Pts',(-0.678027841398909,0.00191949921416389,
-0.978718730873058));
#62932=CARTESIAN_POINT('Ctrl Pts',(-0.678025555836318,-0.00021148764794485,
-0.978617978381028));
#62933=CARTESIAN_POINT('Ctrl Pts',(-0.676874835700589,0.00012642630365326,
-1.13918202161902));
#62934=CARTESIAN_POINT('Ctrl Pts',(-0.676728340351803,-0.104284756028837,
-1.13425538078747));
#62935=CARTESIAN_POINT('Ctrl Pts',(-0.624782516817017,-0.321261817775614,
-1.12403320712446));
#62936=CARTESIAN_POINT('Ctrl Pts',(-0.328086109575231,-0.669804587776323,
-1.10321996779852));
#62937=CARTESIAN_POINT('Ctrl Pts',(0.303509663064016,-0.740514320182075,
-1.0767423036412));
#62938=CARTESIAN_POINT('Ctrl Pts',(0.787888271911223,-0.143754323166431,
-1.04496910665241));
#62939=CARTESIAN_POINT('Ctrl Pts',(0.586590198965058,0.460620189913425,
-1.01849144249509));
#62940=CARTESIAN_POINT('Ctrl Pts',(0.178153413511559,0.680803502488938,
-0.99730931116923));
#62941=CARTESIAN_POINT('Ctrl Pts',(-0.288068623095297,0.688609403797382,
-0.976127179843373));
#62942=CARTESIAN_POINT('Ctrl Pts',(-0.629476800536546,0.375015729132091,
-0.956751416659968));
#62943=CARTESIAN_POINT('Ctrl Pts',(-0.677013369793962,0.074595539042017,
-0.942671186308028));
#62944=CARTESIAN_POINT('Ctrl Pts',(-0.676726131492095,0.000143228251020609,
-0.939182021619018));
#62945=CARTESIAN_POINT('Origin',(0.,0.,-12.278617978381));
#62946=CARTESIAN_POINT('',(-0.676309172935686,0.00035385414077456,-1.37861797838103));
#62947=CARTESIAN_POINT('',(-0.676973562981676,-0.000235536917071982,-1.33918202161902));
#62948=CARTESIAN_POINT('',(-0.6767,6.12423655037739E-13,-12.278617978381));
#62949=CARTESIAN_POINT('Ctrl Pts',(-0.676309172935686,0.000353854140774549,
-1.37861797838103));
#62950=CARTESIAN_POINT('Ctrl Pts',(-0.676266745049917,-0.0176411785517731,
-1.37777371832634));
#62951=CARTESIAN_POINT('Ctrl Pts',(-0.670883252141012,-0.148573698829888,
-1.37163392544018));
#62952=CARTESIAN_POINT('Ctrl Pts',(-0.555673590256809,-0.498390713899415,
-1.3549030668911));
#62953=CARTESIAN_POINT('Ctrl Pts',(-0.109218024599217,-0.738214330501128,
-1.33372093556524));
#62954=CARTESIAN_POINT('Ctrl Pts',(0.341625653170807,-0.616053413812982,
-1.31253880423938));
#62955=CARTESIAN_POINT('Ctrl Pts',(0.595557808340173,-0.37903650385649,
-1.29665220574499));
#62956=CARTESIAN_POINT('Ctrl Pts',(0.702804700428006,-0.0479112667122281,
-1.2807656072506));
#62957=CARTESIAN_POINT('Ctrl Pts',(0.622422081552932,0.410937262240509,
-1.25958347592474));
#62958=CARTESIAN_POINT('Ctrl Pts',(0.113906261266067,0.792152092474895,
-1.23310581176742));
#62959=CARTESIAN_POINT('Ctrl Pts',(-0.53775175223377,0.548962917234563,
-1.20435213497569));
#62960=CARTESIAN_POINT('Ctrl Pts',(-0.674638215638227,0.160641167462172,
-1.1861895238469));
#62961=CARTESIAN_POINT('Ctrl Pts',(-0.675858962494509,-0.000507684201011542,
-1.17861797838103));
#62962=CARTESIAN_POINT('Ctrl Pts',(-0.676973562981676,-0.000235536917072003,
-1.33918202161902));
#62963=CARTESIAN_POINT('Ctrl Pts',(-0.677234775375011,-0.058816887218812,
-1.33643064092984));
#62964=CARTESIAN_POINT('Ctrl Pts',(-0.641806312782087,-0.342596601065592,
-1.32308819457774));
#62965=CARTESIAN_POINT('Ctrl Pts',(-0.248041461525952,-0.760890929984079,
-1.29915468256271));
#62966=CARTESIAN_POINT('Ctrl Pts',(0.507461495749466,-0.619609606749274,
-1.26738148557393));
#62967=CARTESIAN_POINT('Ctrl Pts',(0.74527725860231,-0.0286501079923499,
-1.2409038214166));
#62968=CARTESIAN_POINT('Ctrl Pts',(0.576506692556375,0.403574133443626,
-1.21972169009074));
#62969=CARTESIAN_POINT('Ctrl Pts',(0.226209707001196,0.711333684755956,
-1.19853955876488));
#62970=CARTESIAN_POINT('Ctrl Pts',(-0.280199631649522,0.691648133864366,
-1.17735742743902));
#62971=CARTESIAN_POINT('Ctrl Pts',(-0.606835592617558,0.35774356613014,
-1.15617529611317));
#62972=CARTESIAN_POINT('Ctrl Pts',(-0.674911531355438,0.127977621129902,
-1.14521533845032));
#62973=CARTESIAN_POINT('Ctrl Pts',(-0.676885804830273,0.00794442058850271,
-1.13955091361894));
#62974=CARTESIAN_POINT('Ctrl Pts',(-0.676874835700589,0.00012642630365326,
-1.13918202161902));
#62975=CARTESIAN_POINT('Origin',(0.,0.,-12.278617978381));
#62976=CARTESIAN_POINT('',(-0.6767,5.35204042542703E-13,-1.57861797838103));
#62977=CARTESIAN_POINT('',(-0.675366916321589,-0.000162312625430594,-1.53918202161901));
#62978=CARTESIAN_POINT('',(-0.6767,6.12423655037739E-13,-12.278617978381));
#62979=CARTESIAN_POINT('Ctrl Pts',(-0.677053553463528,0.000169628890303121,
-1.57861797838103));
#62980=CARTESIAN_POINT('Ctrl Pts',(-0.675400439898793,-0.195958740493585,
-1.56935791280578));
#62981=CARTESIAN_POINT('Ctrl Pts',(-0.534568406785807,-0.504445956789688,
-1.55480231439907));
#62982=CARTESIAN_POINT('Ctrl Pts',(-0.138419734612189,-0.690702448703422,
-1.5349511831609));
#62983=CARTESIAN_POINT('Ctrl Pts',(0.208558492969346,-0.674433932524933,
-1.5190645846665));
#62984=CARTESIAN_POINT('Ctrl Pts',(0.504655813759805,-0.491479853157888,
-1.50317798617211));
#62985=CARTESIAN_POINT('Ctrl Pts',(0.740425626835783,-0.0897138352053628,
-1.48199585484625));
#62986=CARTESIAN_POINT('Ctrl Pts',(0.599619882655918,0.530033555816679,
-1.45551819068893));
#62987=CARTESIAN_POINT('Ctrl Pts',(-0.123187980897615,0.79136461622102,
-1.42374499370014));
#62988=CARTESIAN_POINT('Ctrl Pts',(-0.611734609152697,0.415005179511451,
-1.39811158959751));
#62989=CARTESIAN_POINT('Ctrl Pts',(-0.676532869522839,0.0952307806240656,
-1.3830692511578));
#62990=CARTESIAN_POINT('Ctrl Pts',(-0.676309172935686,0.000353854140774549,
-1.37861797838103));
#62991=CARTESIAN_POINT('Ctrl Pts',(-0.675366916321589,-0.000162312625430511,
-1.53918202161901));
#62992=CARTESIAN_POINT('Ctrl Pts',(-0.675221364951782,-0.125283662983,-1.53331036824075));
#62993=CARTESIAN_POINT('Ctrl Pts',(-0.582503076894211,-0.476023863715487,
-1.51684764919956));
#62994=CARTESIAN_POINT('Ctrl Pts',(-0.0143232884913037,-0.800767180802928,
-1.48979386449544));
#62995=CARTESIAN_POINT('Ctrl Pts',(0.549496765312817,-0.504293888311659,
-1.46331620033811));
#62996=CARTESIAN_POINT('Ctrl Pts',(0.700662799746577,-0.0656025060371282,
-1.44213406901226));
#62997=CARTESIAN_POINT('Ctrl Pts',(0.632898545584985,0.395734599961226,
-1.4209519376864));
#62998=CARTESIAN_POINT('Ctrl Pts',(0.234174509286621,0.708555766228003,
-1.39976980636054));
#62999=CARTESIAN_POINT('Ctrl Pts',(-0.230938351402798,0.665505351914144,
-1.37858767503468));
#63000=CARTESIAN_POINT('Ctrl Pts',(-0.521748873394984,0.475537472174135,
-1.36270107654029));
#63001=CARTESIAN_POINT('Ctrl Pts',(-0.65605051904258,0.221017565263106,
-1.34956585873506));
#63002=CARTESIAN_POINT('Ctrl Pts',(-0.676732024588713,0.0539335820474626,
-1.34172617376131));
#63003=CARTESIAN_POINT('Ctrl Pts',(-0.676973562981676,-0.000235536917072003,
-1.33918202161902));
#63004=CARTESIAN_POINT('Origin',(0.,0.,-12.278617978381));
#63005=CARTESIAN_POINT('',(-0.6767,4.82147705686052E-13,-1.77861797838102));
#63006=CARTESIAN_POINT('',(-0.677257035716489,0.00088196528073553,-1.73918202161901));
#63007=CARTESIAN_POINT('',(-0.6767,6.12423655037739E-13,-12.278617978381));
#63008=CARTESIAN_POINT('Ctrl Pts',(-0.6767,4.82147705686052E-13,-1.77861797838102));
#63009=CARTESIAN_POINT('Ctrl Pts',(-0.676700000000059,-0.082119756793935,
-1.77475518387258));
#63010=CARTESIAN_POINT('Ctrl Pts',(-0.661576824416428,-0.164280093512661,
-1.7708893545134));
#63011=CARTESIAN_POINT('Ctrl Pts',(-0.632313905337345,-0.241043595884718,
-1.76702504257958));
#63012=CARTESIAN_POINT('Ctrl Pts',(-0.562558735104792,-0.424027773271085,
-1.75781353035667));
#63013=CARTESIAN_POINT('Ctrl Pts',(-0.40938922223103,-0.573299527009233,
-1.74860201813377));
#63014=CARTESIAN_POINT('Ctrl Pts',(-0.224668156292418,-0.638315838396766,
-1.73939050591086));
#63015=CARTESIAN_POINT('Ctrl Pts',(-0.0399470903538051,-0.703332149784298,
-1.73017899368795));
#63016=CARTESIAN_POINT('Ctrl Pts',(0.172951249061904,-0.68290537294406,
-1.72096748146505));
#63017=CARTESIAN_POINT('Ctrl Pts',(0.341940050610126,-0.58395196017202,
-1.71175596924214));
#63018=CARTESIAN_POINT('Ctrl Pts',(0.510928852158348,-0.484998547399981,
-1.70254445701923));
#63019=CARTESIAN_POINT('Ctrl Pts',(0.632921215811054,-0.309326069907138,
-1.69333294479633));
#63020=CARTESIAN_POINT('Ctrl Pts',(0.666610851776377,-0.116416761224374,
-1.68412143257342));
#63021=CARTESIAN_POINT('Ctrl Pts',(0.700300487741701,0.0764925474583901,
-1.67490992035051));
#63022=CARTESIAN_POINT('Ctrl Pts',(0.645071991109655,0.28311483400515,-1.66569840812761));
#63023=CARTESIAN_POINT('Ctrl Pts',(0.519625583913373,0.433488341876326,
-1.6564868959047));
#63024=CARTESIAN_POINT('Ctrl Pts',(0.394179176717091,0.583861849747502,
-1.64727538368179));
#63025=CARTESIAN_POINT('Ctrl Pts',(0.200806374810538,0.67523972245669,-1.63806387145888));
#63026=CARTESIAN_POINT('Ctrl Pts',(0.0049826944822306,0.6766816554006,-1.62885235923598));
#63027=CARTESIAN_POINT('Ctrl Pts',(-0.190840985846077,0.678123588344511,
-1.61964084701307));
#63028=CARTESIAN_POINT('Ctrl Pts',(-0.385538454760861,0.589603241891143,
-1.61042933479017));
#63029=CARTESIAN_POINT('Ctrl Pts',(-0.51318566724868,0.441093369855553,
-1.60121782256726));
#63030=CARTESIAN_POINT('Ctrl Pts',(-0.61757703619451,0.319640276273546,
-1.59368454117185));
#63031=CARTESIAN_POINT('Ctrl Pts',(-0.676699999999874,0.159958743945511,
-1.5861422061894));
#63032=CARTESIAN_POINT('Ctrl Pts',(-0.6767,5.35204119005623E-13,-1.57861797838103));
#63033=CARTESIAN_POINT('Ctrl Pts',(-0.677257035716489,0.000881965280735513,
-1.73918202161901));
#63034=CARTESIAN_POINT('Ctrl Pts',(-0.675585900234077,-0.189916695348646,
-1.73019009555166));
#63035=CARTESIAN_POINT('Ctrl Pts',(-0.491749932536183,-0.609461463096116,
-1.71060710382138));
#63036=CARTESIAN_POINT('Ctrl Pts',(0.0923655176653327,-0.740086232829771,
-1.68572857925962));
#63037=CARTESIAN_POINT('Ctrl Pts',(0.491570810089264,-0.5035773887053,-1.66454644793377));
#63038=CARTESIAN_POINT('Ctrl Pts',(0.738569211247283,-0.10808312915354,
-1.64336431660791));
#63039=CARTESIAN_POINT('Ctrl Pts',(0.637170952451161,0.388461261913037,
-1.62218218528205));
#63040=CARTESIAN_POINT('Ctrl Pts',(0.254797411454479,0.656740568787333,
-1.60100005395619));
#63041=CARTESIAN_POINT('Ctrl Pts',(-0.0898318649340317,0.700205691474415,
-1.5851134554618));
#63042=CARTESIAN_POINT('Ctrl Pts',(-0.412913548481974,0.570729653953337,
-1.56922685696741));
#63043=CARTESIAN_POINT('Ctrl Pts',(-0.630596046941778,0.313852223971835,
-1.55391637901981));
#63044=CARTESIAN_POINT('Ctrl Pts',(-0.675483904992149,0.100405483174212,
-1.54390143390368));
#63045=CARTESIAN_POINT('Ctrl Pts',(-0.675366916321589,-0.000162312625430511,
-1.53918202161901));
#63046=CARTESIAN_POINT('Origin',(0.,0.,-12.278617978381));
#63047=CARTESIAN_POINT('',(-0.6767,4.6755719955438E-13,-1.97861797838102));
#63048=CARTESIAN_POINT('',(-0.677446490839416,-0.000787741955589949,-1.93918202161901));
#63049=CARTESIAN_POINT('',(-0.6767,6.12423655037739E-13,-12.278617978381));
#63050=CARTESIAN_POINT('Ctrl Pts',(-0.676413475060879,-0.000340497908876618,
-1.97861797838102));
#63051=CARTESIAN_POINT('Ctrl Pts',(-0.676278753013238,-0.104907816759115,
-1.97370843309053));
#63052=CARTESIAN_POINT('Ctrl Pts',(-0.626229281881828,-0.321358158604508,
-1.96350335496856));
#63053=CARTESIAN_POINT('Ctrl Pts',(-0.403309811719612,-0.577556172326435,
-1.94800274401514));
#63054=CARTESIAN_POINT('Ctrl Pts',(0.0313217580437868,-0.745182949734803,
-1.92682061268927));
#63055=CARTESIAN_POINT('Ctrl Pts',(0.620103828443481,-0.505915819003228,
-1.90034294853195));
#63056=CARTESIAN_POINT('Ctrl Pts',(0.760987813965571,0.249661333490343,
-1.86856975154317));
#63057=CARTESIAN_POINT('Ctrl Pts',(0.295673986471208,0.684715937160779,
-1.84209208738584));
#63058=CARTESIAN_POINT('Ctrl Pts',(-0.168329559292972,0.683298768632944,
-1.82090995605999));
#63059=CARTESIAN_POINT('Ctrl Pts',(-0.546841497105642,0.485885352754348,
-1.80151709733553));
#63060=CARTESIAN_POINT('Ctrl Pts',(-0.674917444468637,0.186609400672984,
-1.78741977144254));
#63061=CARTESIAN_POINT('Ctrl Pts',(-0.676717196229297,-0.000122736083201944,
-1.77861797838102));
#63062=CARTESIAN_POINT('Ctrl Pts',(-0.677446490839416,-0.000787741955589942,
-1.93918202161901));
#63063=CARTESIAN_POINT('Ctrl Pts',(-0.677732392339807,-0.0330590201563695,
-1.9376608885255));
#63064=CARTESIAN_POINT('Ctrl Pts',(-0.661044596458893,-0.289636215322383,
-1.92554868976905));
#63065=CARTESIAN_POINT('Ctrl Pts',(-0.408696466689488,-0.62387997162377,
-1.90814095818113));
#63066=CARTESIAN_POINT('Ctrl Pts',(0.0486787143220458,-0.702041615945249,
-1.88695882685528));
#63067=CARTESIAN_POINT('Ctrl Pts',(0.492962794513711,-0.560494536846958,
-1.86577669552942));
#63068=CARTESIAN_POINT('Ctrl Pts',(0.737117187516088,-0.116392553554602,
-1.84459456420356));
#63069=CARTESIAN_POINT('Ctrl Pts',(0.619346845481977,0.335617908590315,
-1.8234124328777));
#63070=CARTESIAN_POINT('Ctrl Pts',(0.384810828458858,0.591843223017294,
-1.80752583438331));
#63071=CARTESIAN_POINT('Ctrl Pts',(0.0547443097277555,0.702305486931504,
-1.79163923588892));
#63072=CARTESIAN_POINT('Ctrl Pts',(-0.404864299349843,0.626389320003439,
-1.77045710456306));
#63073=CARTESIAN_POINT('Ctrl Pts',(-0.659871184498933,0.293031979129122,
-1.75297136647309));
#63074=CARTESIAN_POINT('Ctrl Pts',(-0.677554233324596,0.0348139272107488,
-1.74078116121459));
#63075=CARTESIAN_POINT('Ctrl Pts',(-0.677257035716489,0.000881965280735513,
-1.73918202161901));
#63076=CARTESIAN_POINT('Origin',(0.,0.,-12.278617978381));
#63077=CARTESIAN_POINT('',(-0.6767,4.52966762133127E-13,-2.17861797838102));
#63078=CARTESIAN_POINT('',(-0.675328212337249,-8.63283092417122E-5,-2.13918202161901));
#63079=CARTESIAN_POINT('',(-0.6767,6.12423655037739E-13,-12.278617978381));
#63080=CARTESIAN_POINT('Ctrl Pts',(-0.6767,4.91432703676236E-13,-2.17861797838103));
#63081=CARTESIAN_POINT('Ctrl Pts',(-0.676700000000127,-0.17490534537463,
-2.17039068407346));
#63082=CARTESIAN_POINT('Ctrl Pts',(-0.605526598979385,-0.349171323828889,
-2.16214503008812));
#63083=CARTESIAN_POINT('Ctrl Pts',(-0.482847266157599,-0.47411117637547,
-2.15390855594167));
#63084=CARTESIAN_POINT('Ctrl Pts',(-0.345645090360969,-0.613841473393005,
-2.14469704371876));
#63085=CARTESIAN_POINT('Ctrl Pts',(-0.145512713664304,-0.689273482088197,
-2.13548553149585));
#63086=CARTESIAN_POINT('Ctrl Pts',(0.049785573602703,-0.674866124991505,
-2.12627401927295));
#63087=CARTESIAN_POINT('Ctrl Pts',(0.24508386086971,-0.660458767894813,
-2.11706250705004));
#63088=CARTESIAN_POINT('Ctrl Pts',(0.431980566169593,-0.556475222628767,
-2.10785099482713));
#63089=CARTESIAN_POINT('Ctrl Pts',(0.547192962296249,-0.398124040989057,
-2.09863948260423));
#63090=CARTESIAN_POINT('Ctrl Pts',(0.662405358422905,-0.239772859349346,
-2.08942797038132));
#63091=CARTESIAN_POINT('Ctrl Pts',(0.70382887308767,-0.0299466251200073,
-2.08021645815841));
#63092=CARTESIAN_POINT('Ctrl Pts',(0.657437614425613,0.160308056997643,
-2.07100494593551));
#63093=CARTESIAN_POINT('Ctrl Pts',(0.611046355763555,0.350562739115292,
-2.0617934337126));
#63094=CARTESIAN_POINT('Ctrl Pts',(0.477687747842733,0.517770507569595,
-2.05258192148969));
#63095=CARTESIAN_POINT('Ctrl Pts',(0.302516660526142,0.60531525679113,-2.04337040926679));
#63096=CARTESIAN_POINT('Ctrl Pts',(0.127345573209552,0.692860006012664,
-2.03415889704388));
#63097=CARTESIAN_POINT('Ctrl Pts',(-0.0864381623341533,0.699142565604636,
-2.02494738482097));
#63098=CARTESIAN_POINT('Ctrl Pts',(-0.266447941986903,0.622035677602937,
-2.01573587259807));
#63099=CARTESIAN_POINT('Ctrl Pts',(-0.446457721639652,0.544928789601237,
-2.00652436037516));
#63100=CARTESIAN_POINT('Ctrl Pts',(-0.589405326367021,0.385840957128872,
-1.99731284815225));
#63101=CARTESIAN_POINT('Ctrl Pts',(-0.646889077497289,0.198638897033553,
-1.98810133592935));
#63102=CARTESIAN_POINT('Ctrl Pts',(-0.666615804662001,0.134396673943352,
-1.98494021674657));
#63103=CARTESIAN_POINT('Ctrl Pts',(-0.676699999999954,0.0671595727141406,
-1.98177706748205));
#63104=CARTESIAN_POINT('Ctrl Pts',(-0.6767,4.6755723390959E-13,-1.97861797838102));
#63105=CARTESIAN_POINT('Ctrl Pts',(-0.675328212337249,-8.63283092416567E-5,
-2.13918202161901));
#63106=CARTESIAN_POINT('Ctrl Pts',(-0.675444524571566,-0.0990680295131166,
-2.1345406158364));
#63107=CARTESIAN_POINT('Ctrl Pts',(-0.63166980646997,-0.310842263830983,
-2.12460367722233));
#63108=CARTESIAN_POINT('Ctrl Pts',(-0.417365872073619,-0.566601956028473,
-2.10937120577679));
#63109=CARTESIAN_POINT('Ctrl Pts',(0.0128942183109048,-0.74632444804134,
-2.08818907445093));
#63110=CARTESIAN_POINT('Ctrl Pts',(0.486476949341432,-0.565887932734067,
-2.06700694312507));
#63111=CARTESIAN_POINT('Ctrl Pts',(0.689323544065248,-0.145130793329111,
-2.04582481179921));
#63112=CARTESIAN_POINT('Ctrl Pts',(0.676430423898524,0.201989247127572,
-2.02993821330482));
#63113=CARTESIAN_POINT('Ctrl Pts',(0.496364768725477,0.499851930865303,
-2.01405161481042));
#63114=CARTESIAN_POINT('Ctrl Pts',(0.0969107931718748,0.739518072307371,
-1.99286948348457));
#63115=CARTESIAN_POINT('Ctrl Pts',(-0.488495455026634,0.612489083801584,
-1.96791295242076));
#63116=CARTESIAN_POINT('Ctrl Pts',(-0.675741769969761,0.19163349880046,
-1.94825195418842));
#63117=CARTESIAN_POINT('Ctrl Pts',(-0.677446490839416,-0.000787741955589942,
-1.93918202161901));
#63118=CARTESIAN_POINT('Origin',(0.,0.,-12.278617978381));
#63119=CARTESIAN_POINT('',(-0.677485359766029,-0.000107376913780513,-2.37861797838102));
#63120=CARTESIAN_POINT('',(-0.676795338809115,0.000510576453991912,-2.33918202161901));
#63121=CARTESIAN_POINT('',(-0.6767,6.12423655037739E-13,-12.278617978381));
#63122=CARTESIAN_POINT('Ctrl Pts',(-0.677485359766029,-0.000107376913780525,
-2.37861797838102));
#63123=CARTESIAN_POINT('Ctrl Pts',(-0.677488765774498,-0.0119719264639521,
-2.37805895337527));
#63124=CARTESIAN_POINT('Ctrl Pts',(-0.670999253114086,-0.248539305774364,
-2.36690886270659));
#63125=CARTESIAN_POINT('Ctrl Pts',(-0.398867864803067,-0.693818420334465,
-2.34516770637498));
#63126=CARTESIAN_POINT('Ctrl Pts',(0.369549690352763,-0.710539415377113,
-2.31339450938619));
#63127=CARTESIAN_POINT('Ctrl Pts',(0.723546655452461,-0.180939929980367,
-2.28691684522887));
#63128=CARTESIAN_POINT('Ctrl Pts',(0.647040070382234,0.276715006941831,
-2.26573471390301));
#63129=CARTESIAN_POINT('Ctrl Pts',(0.36733345238644,0.649794257721565,-2.24455258257715));
#63130=CARTESIAN_POINT('Ctrl Pts',(-0.132342674989519,0.734421126487522,
-2.22337045125129));
#63131=CARTESIAN_POINT('Ctrl Pts',(-0.520533786771069,0.474630880163505,
-2.20218831992543));
#63132=CARTESIAN_POINT('Ctrl Pts',(-0.657056894194546,0.221529119030303,
-2.18903600657917));
#63133=CARTESIAN_POINT('Ctrl Pts',(-0.676586384573887,0.0548096435792028,
-2.18117922606436));
#63134=CARTESIAN_POINT('Ctrl Pts',(-0.676477391207069,0.000385350982612692,
-2.17861797838103));
#63135=CARTESIAN_POINT('Ctrl Pts',(-0.676795338809115,0.000510576453991895,
-2.33918202161901));
#63136=CARTESIAN_POINT('Ctrl Pts',(-0.676521639134244,-0.0519039108123045,
-2.33671587597878));
#63137=CARTESIAN_POINT('Ctrl Pts',(-0.656639741323987,-0.217177799902405,
-2.32895419750708));
#63138=CARTESIAN_POINT('Ctrl Pts',(-0.473307084952599,-0.57718874377774,
-2.31060145337244));
#63139=CARTESIAN_POINT('Ctrl Pts',(0.0044593387890197,-0.746236617268379,
-2.28941932204658));
#63140=CARTESIAN_POINT('Ctrl Pts',(0.431445304074627,-0.5568526242795,-2.26823719072073));
#63141=CARTESIAN_POINT('Ctrl Pts',(0.646327285527458,-0.283934524694336,
-2.25235059222633));
#63142=CARTESIAN_POINT('Ctrl Pts',(0.701905026833796,0.0596596155461771,
-2.23646399373194));
#63143=CARTESIAN_POINT('Ctrl Pts',(0.552593332470904,0.500918446467205,
-2.21528186240608));
#63144=CARTESIAN_POINT('Ctrl Pts',(-0.00803857589287147,0.800259305016558,
-2.18880419824876));
#63145=CARTESIAN_POINT('Ctrl Pts',(-0.580828746386521,0.479835670177724,
-2.16167240704258));
#63146=CARTESIAN_POINT('Ctrl Pts',(-0.675179115648332,0.126794940884012,
-2.14513168149933));
#63147=CARTESIAN_POINT('Ctrl Pts',(-0.675328212337249,-8.63283092416567E-5,
-2.13918202161901));
#63148=CARTESIAN_POINT('Origin',(0.,0.,-12.278617978381));
#63149=CARTESIAN_POINT('',(-0.67667083393025,-2.5222838540107E-5,-2.57861797838102));
#63150=CARTESIAN_POINT('',(-0.677533761904701,-0.000330077543184093,-2.53918202161901));
#63151=CARTESIAN_POINT('',(-0.6767,6.12423655037739E-13,-12.278617978381));
#63152=CARTESIAN_POINT('Ctrl Pts',(-0.675978983105548,-0.000623535949907557,
-2.57861797838102));
#63153=CARTESIAN_POINT('Ctrl Pts',(-0.67660824076582,-0.0788507797028598,
-2.57493868068618));
#63154=CARTESIAN_POINT('Ctrl Pts',(-0.628107327354101,-0.381596062206871,
-2.56066831732841));
#63155=CARTESIAN_POINT('Ctrl Pts',(-0.178302031962507,-0.780795504496738,
-2.53580688830771));
#63156=CARTESIAN_POINT('Ctrl Pts',(0.434348713906479,-0.606300433453199,
-2.50932922415038));
#63157=CARTESIAN_POINT('Ctrl Pts',(0.672300129659377,-0.207953320259739,
-2.48814709282452));
#63158=CARTESIAN_POINT('Ctrl Pts',(0.70062407108951,0.257473015323963,-2.46696496149866));
#63159=CARTESIAN_POINT('Ctrl Pts',(0.374558924196536,0.645441389251823,
-2.44578283017281));
#63160=CARTESIAN_POINT('Ctrl Pts',(-0.0894926216029255,0.698728106099681,
-2.42460069884695));
#63161=CARTESIAN_POINT('Ctrl Pts',(-0.413090643562724,0.572463007129391,
-2.40871410035255));
#63162=CARTESIAN_POINT('Ctrl Pts',(-0.627406575776416,0.313931316160718,
-2.39338652686391));
#63163=CARTESIAN_POINT('Ctrl Pts',(-0.677456501332862,0.100418594580537,
-2.38335448620674));
#63164=CARTESIAN_POINT('Ctrl Pts',(-0.677485359766029,-0.000107376913780525,
-2.37861797838102));
#63165=CARTESIAN_POINT('Ctrl Pts',(-0.6775337619047,-0.000330077543184071,
-2.53918202161901));
#63166=CARTESIAN_POINT('Ctrl Pts',(-0.677535144161109,-0.00649456504868987,
-2.53889113612115));
#63167=CARTESIAN_POINT('Ctrl Pts',(-0.674213842716546,-0.23704730980286,
-2.52800918496036));
#63168=CARTESIAN_POINT('Ctrl Pts',(-0.47967921519751,-0.571661460273545,
-2.51183170096809));
#63169=CARTESIAN_POINT('Ctrl Pts',(-0.0316362470218281,-0.703725119240024,
-2.49064956964224));
#63170=CARTESIAN_POINT('Ctrl Pts',(0.308819018868513,-0.634813821459323,
-2.47476297114784));
#63171=CARTESIAN_POINT('Ctrl Pts',(0.573606362075548,-0.408907908713105,
-2.45887637265346));
#63172=CARTESIAN_POINT('Ctrl Pts',(0.745452333195922,0.0240728069648603,
-2.43769424132759));
#63173=CARTESIAN_POINT('Ctrl Pts',(0.511922871354516,0.615154084561029,
-2.41121657717027));
#63174=CARTESIAN_POINT('Ctrl Pts',(-0.242248341456588,0.763379967975192,
-2.37944338018148));
#63175=CARTESIAN_POINT('Ctrl Pts',(-0.640867055936252,0.345262845662194,
-2.3554318616644));
#63176=CARTESIAN_POINT('Ctrl Pts',(-0.677109352037566,0.0606452564527683,
-2.34201140881024));
#63177=CARTESIAN_POINT('Ctrl Pts',(-0.676795338809115,0.000510576453991895,
-2.33918202161901));
#63178=CARTESIAN_POINT('Origin',(0.,0.,-12.278617978381));
#63179=CARTESIAN_POINT('',(-0.676628694961864,5.74670372185009E-5,-2.77861797838102));
#63180=CARTESIAN_POINT('',(-0.6767,4.20837301638721E-13,-2.73918202161901));
#63181=CARTESIAN_POINT('',(-0.6767,6.12423655037739E-13,-12.278617978381));
#63182=CARTESIAN_POINT('Ctrl Pts',(-0.6767,4.0919534680374E-13,-2.77861797838102));
#63183=CARTESIAN_POINT('Ctrl Pts',(-0.676700000000072,-0.118639299394314,
-2.77303735744305));
#63184=CARTESIAN_POINT('Ctrl Pts',(-0.644770474758931,-0.237238798212155,
-2.76745156789602));
#63185=CARTESIAN_POINT('Ctrl Pts',(-0.585155688320175,-0.339876022141225,
-2.76186836265352));
#63186=CARTESIAN_POINT('Ctrl Pts',(-0.4867995810135,-0.509213168401033,
-2.75265685043061));
#63187=CARTESIAN_POINT('Ctrl Pts',(-0.311558945829397,-0.631825059824009,
-2.74344533820771));
#63188=CARTESIAN_POINT('Ctrl Pts',(-0.118769795641856,-0.666195636163426,
-2.7342338259848));
#63189=CARTESIAN_POINT('Ctrl Pts',(0.0740193545456853,-0.700566212502843,
-2.72502231376189));
#63190=CARTESIAN_POINT('Ctrl Pts',(0.280835361332882,-0.646067630185082,
-2.71581080153898));
#63191=CARTESIAN_POINT('Ctrl Pts',(0.431650875022103,-0.52115296419828,
-2.70659928931608));
#63192=CARTESIAN_POINT('Ctrl Pts',(0.582466388711323,-0.396238298211477,
-2.69738777709317));
#63193=CARTESIAN_POINT('Ctrl Pts',(0.67452647874404,-0.203189351150853,
-2.68817626487027));
#63194=CARTESIAN_POINT('Ctrl Pts',(0.676659843546144,-0.0073719829156555,
-2.67896475264736));
#63195=CARTESIAN_POINT('Ctrl Pts',(0.678793208348247,0.188445385319542,
-2.66975324042445));
#63196=CARTESIAN_POINT('Ctrl Pts',(0.590960877977311,0.383454200196352,
-2.66054172820154));
#63197=CARTESIAN_POINT('Ctrl Pts',(0.442902645833232,0.511624995786878,
-2.65133021597864));
#63198=CARTESIAN_POINT('Ctrl Pts',(0.294844413689154,0.639795791377403,
-2.64211870375573));
#63199=CARTESIAN_POINT('Ctrl Pts',(0.0892648433688601,0.698787285721679,
-2.63290719153282));
#63200=CARTESIAN_POINT('Ctrl Pts',(-0.104227369528373,0.668625115772057,
-2.62369567930992));
#63201=CARTESIAN_POINT('Ctrl Pts',(-0.297719582425605,0.638462945822435,
-2.61448416708701));
#63202=CARTESIAN_POINT('Ctrl Pts',(-0.475589936726069,0.51969808065148,
-2.6052726548641));
#63203=CARTESIAN_POINT('Ctrl Pts',(-0.577612003658916,0.352543987651375,
-2.5960611426412));
#63204=CARTESIAN_POINT('Ctrl Pts',(-0.642009235753148,0.247034843933341,
-2.59024675455447));
#63205=CARTESIAN_POINT('Ctrl Pts',(-0.676699999999923,0.123541506275678,
-2.58442919203574));
#63206=CARTESIAN_POINT('Ctrl Pts',(-0.6767,4.23785818580202E-13,-2.57861797838102));
#63207=CARTESIAN_POINT('Ctrl Pts',(-0.675745563573596,-0.000158715524651409,
-2.73918202161901));
#63208=CARTESIAN_POINT('Ctrl Pts',(-0.676298042296179,-0.072673869664635,
-2.73577086343205));
#63209=CARTESIAN_POINT('Ctrl Pts',(-0.648898766616171,-0.257625310384307,
-2.72706417241364));
#63210=CARTESIAN_POINT('Ctrl Pts',(-0.479671017962049,-0.51589302195539,
-2.71306194856376));
#63211=CARTESIAN_POINT('Ctrl Pts',(-0.17556924533772,-0.683764004918535,
-2.69717535006935));
#63212=CARTESIAN_POINT('Ctrl Pts',(0.172489975910581,-0.682991321051767,
-2.68128875157497));
#63213=CARTESIAN_POINT('Ctrl Pts',(0.583760512301853,-0.464222301682604,
-2.6601066202491));
#63214=CARTESIAN_POINT('Ctrl Pts',(0.78840439834167,0.137470282764965,-2.63362895609179));
#63215=CARTESIAN_POINT('Ctrl Pts',(0.309536410753203,0.738661251767208,
-2.601855759103));
#63216=CARTESIAN_POINT('Ctrl Pts',(-0.323960533014889,0.671795053514425,
-2.57537809494567));
#63217=CARTESIAN_POINT('Ctrl Pts',(-0.622531331628934,0.324975084275381,
-2.55448684911768));
#63218=CARTESIAN_POINT('Ctrl Pts',(-0.677509980362131,0.105729131953435,
-2.54418666895261));
#63219=CARTESIAN_POINT('Ctrl Pts',(-0.6775337619047,-0.000330077543184071,
-2.53918202161901));
#63220=CARTESIAN_POINT('Origin',(0.,0.,-12.278617978381));
#63221=CARTESIAN_POINT('',(-0.677908152078298,4.26345795243129E-5,-2.97861797838102));
#63222=CARTESIAN_POINT('',(-0.6767,4.06246809000637E-13,-2.93918202161901));
#63223=CARTESIAN_POINT('',(-0.6767,6.12423655037739E-13,-12.278617978381));
#63224=CARTESIAN_POINT('Ctrl Pts',(-0.677908152078298,4.26345795242825E-5,
-2.97861797838102));
#63225=CARTESIAN_POINT('Ctrl Pts',(-0.676769184190078,-0.209797877091866,
-2.96869813530799));
#63226=CARTESIAN_POINT('Ctrl Pts',(-0.514319791207873,-0.532159781908597,
-2.95348275940349));
#63227=CARTESIAN_POINT('Ctrl Pts',(-0.0963858541361063,-0.697095269579071,
-2.93297185066755));
#63228=CARTESIAN_POINT('Ctrl Pts',(0.367487293040394,-0.649707266439206,
-2.91178971934168));
#63229=CARTESIAN_POINT('Ctrl Pts',(0.697559134358486,-0.265141903002185,
-2.89060758801583));
#63230=CARTESIAN_POINT('Ctrl Pts',(0.675027237917631,0.201415301415524,
-2.86942545668997));
#63231=CARTESIAN_POINT('Ctrl Pts',(0.498046596364184,0.500307267767271,
-2.85353885819557));
#63232=CARTESIAN_POINT('Ctrl Pts',(0.197663098653,0.676135515893496,-2.83765225970118));
#63233=CARTESIAN_POINT('Ctrl Pts',(-0.267743933191193,0.696126330016126,
-2.81647012837532));
#63234=CARTESIAN_POINT('Ctrl Pts',(-0.625584717941753,0.387828683972334,
-2.79679203460194));
#63235=CARTESIAN_POINT('Ctrl Pts',(-0.676382811519772,0.0816008323186632,
-2.78240947366002));
#63236=CARTESIAN_POINT('Ctrl Pts',(-0.675875234839626,0.000664704922657085,
-2.77861797838102));
#63237=CARTESIAN_POINT('Ctrl Pts',(-0.6767,4.44712750543746E-13,-2.93918202161901));
#63238=CARTESIAN_POINT('Ctrl Pts',(-0.676700000000054,-0.0815064203030644,
-2.93534807757142));
#63239=CARTESIAN_POINT('Ctrl Pts',(-0.66180401409219,-0.163055071082539,
-2.9315110623169));
#63240=CARTESIAN_POINT('Ctrl Pts',(-0.63296657669995,-0.239324471754867,
-2.92767558266584));
#63241=CARTESIAN_POINT('Ctrl Pts',(-0.563708900689919,-0.422497524526358,
-2.91846407044293));
#63242=CARTESIAN_POINT('Ctrl Pts',(-0.410945580703484,-0.572184946191539,
-2.90925255822003));
#63243=CARTESIAN_POINT('Ctrl Pts',(-0.226401870485963,-0.637702973993737,
-2.90004104599712));
#63244=CARTESIAN_POINT('Ctrl Pts',(-0.0418581602684427,-0.703221001795936,
-2.89082953377421));
#63245=CARTESIAN_POINT('Ctrl Pts',(0.171094900330045,-0.683372825058906,
-2.88161802155131));
#63246=CARTESIAN_POINT('Ctrl Pts',(0.340351971518003,-0.584878983622944,
-2.8724065093284));
#63247=CARTESIAN_POINT('Ctrl Pts',(0.509609042705961,-0.486385142186983,
-2.86319499710549));
#63248=CARTESIAN_POINT('Ctrl Pts',(0.632078324003079,-0.311044812323557,
-2.85398348488259));
#63249=CARTESIAN_POINT('Ctrl Pts',(0.666292042571853,-0.118227763259854,
-2.84477197265968));
#63250=CARTESIAN_POINT('Ctrl Pts',(0.700505761140627,0.0745892858038498,
-2.83556046043677));
#63251=CARTESIAN_POINT('Ctrl Pts',(0.645838938711248,0.281360886038317,
-2.82634894821387));
#63252=CARTESIAN_POINT('Ctrl Pts',(0.52080161592607,0.432074723686534,-2.81713743599096));
#63253=CARTESIAN_POINT('Ctrl Pts',(0.395764293140892,0.582788561334751,
-2.80792592376805));
#63254=CARTESIAN_POINT('Ctrl Pts',(0.202640513153508,0.674691563143353,
-2.79871441154515));
#63255=CARTESIAN_POINT('Ctrl Pts',(0.0068214740930863,0.67666561719301,
-2.78950289932224));
#63256=CARTESIAN_POINT('Ctrl Pts',(-0.188997564967335,0.678639671242668,
-2.78029138709933));
#63257=CARTESIAN_POINT('Ctrl Pts',(-0.383934858047051,0.590648717703111,
-2.77107987487643));
#63258=CARTESIAN_POINT('Ctrl Pts',(-0.511985156308387,0.442486259357142,
-2.76186836265352));
#63259=CARTESIAN_POINT('Ctrl Pts',(-0.617106974370762,0.320853532206972,
-2.75430624897535));
#63260=CARTESIAN_POINT('Ctrl Pts',(-0.6766999999999,0.160570324119808,-2.74673501727365));
#63261=CARTESIAN_POINT('Ctrl Pts',(-0.6767,4.20837280777099E-13,-2.73918202161901));
#63262=CARTESIAN_POINT('Origin',(0.,0.,-12.278617978381));
#63263=CARTESIAN_POINT('',(-0.676187862115932,-0.000564937425030058,-3.17861797838102));
#63264=CARTESIAN_POINT('',(-0.67679285177372,0.000237387877347908,-3.13918202161901));
#63265=CARTESIAN_POINT('',(-0.6767,6.12423655037739E-13,-12.278617978381));
#63266=CARTESIAN_POINT('Ctrl Pts',(-0.676187862115932,-0.000564937425030061,
-3.17861797838102));
#63267=CARTESIAN_POINT('Ctrl Pts',(-0.676644491535547,-0.0526279803465272,
-3.17616892828183));
#63268=CARTESIAN_POINT('Ctrl Pts',(-0.659369213156443,-0.216993979854592,
-3.16842434535117));
#63269=CARTESIAN_POINT('Ctrl Pts',(-0.524730724624935,-0.468923996380709,
-3.15538422958906));
#63270=CARTESIAN_POINT('Ctrl Pts',(-0.140494133246507,-0.733094701340396,
-3.1342020982632));
#63271=CARTESIAN_POINT('Ctrl Pts',(0.360032912737676,-0.653655319262541,
-3.11301996693734));
#63272=CARTESIAN_POINT('Ctrl Pts',(0.644886244911881,-0.283463625000574,
-3.09183783561148));
#63273=CARTESIAN_POINT('Ctrl Pts',(0.703481663861427,0.0589179339543426,
-3.07595123711709));
#63274=CARTESIAN_POINT('Ctrl Pts',(0.588354962968238,0.38738659498273,-3.06006463862269));
#63275=CARTESIAN_POINT('Ctrl Pts',(0.246567099391958,0.703905779632369,
-3.03888250729684));
#63276=CARTESIAN_POINT('Ctrl Pts',(-0.388958651052195,0.699421719522368,
-3.01240484313951));
#63277=CARTESIAN_POINT('Ctrl Pts',(-0.671229579838026,0.252454363145372,
-2.99055148922376));
#63278=CARTESIAN_POINT('Ctrl Pts',(-0.677985219928073,0.0142414168257241,
-2.97928920097093));
#63279=CARTESIAN_POINT('Ctrl Pts',(-0.677908152078298,4.26345795242825E-5,
-2.97861797838102));
#63280=CARTESIAN_POINT('Ctrl Pts',(-0.67679285177372,0.000237387877347905,
-3.13918202161901));
#63281=CARTESIAN_POINT('Ctrl Pts',(-0.676567324318828,-0.0921345146587963,
-3.13482585088534));
#63282=CARTESIAN_POINT('Ctrl Pts',(-0.633537174009138,-0.297198424375294,
-3.1251741473202));
#63283=CARTESIAN_POINT('Ctrl Pts',(-0.363607076602154,-0.651205478284122,
-3.10493137809214));
#63284=CARTESIAN_POINT('Ctrl Pts',(0.263276112884758,-0.755754763367232,
-3.0784537139348));
#63285=CARTESIAN_POINT('Ctrl Pts',(0.779024453182575,-0.18588742772943,
-3.04668051694603));
#63286=CARTESIAN_POINT('Ctrl Pts',(0.610496128531625,0.428431439002367,
-3.0202028527887));
#63287=CARTESIAN_POINT('Ctrl Pts',(0.214482113777081,0.670245828496365,
-2.99902072146284));
#63288=CARTESIAN_POINT('Ctrl Pts',(-0.250646737033531,0.703095054615309,
-2.97783859013698));
#63289=CARTESIAN_POINT('Ctrl Pts',(-0.618947531810959,0.399622239638097,
-2.9578923568557));
#63290=CARTESIAN_POINT('Ctrl Pts',(-0.676858577889835,0.0866323387819684,
-2.94324165640589));
#63291=CARTESIAN_POINT('Ctrl Pts',(-0.676596105090679,3.86521990314997E-6,
-2.93918202161901));
#63292=CARTESIAN_POINT('Origin',(0.,0.,-12.278617978381));
#63293=CARTESIAN_POINT('',(-0.6767,3.65423945443422E-13,-3.37861797838102));
#63294=CARTESIAN_POINT('',(-0.677150171393189,-0.000258134096645546,-3.33918202161901));
#63295=CARTESIAN_POINT('',(-0.6767,6.12423655037739E-13,-12.278617978381));
#63296=CARTESIAN_POINT('Ctrl Pts',(-0.67623262201224,0.000222076779409647,
-3.37861797838102));
#63297=CARTESIAN_POINT('Ctrl Pts',(-0.676226890528276,-0.00561783417541074,
-3.3783441884242));
#63298=CARTESIAN_POINT('Ctrl Pts',(-0.674616485481495,-0.124427520960238,
-3.37277486563592));
#63299=CARTESIAN_POINT('Ctrl Pts',(-0.581653969262653,-0.467808831309393,
-3.35661447718471));
#63300=CARTESIAN_POINT('Ctrl Pts',(-0.148731575015875,-0.731278259794368,
-3.33543234585885));
#63301=CARTESIAN_POINT('Ctrl Pts',(0.308025509003036,-0.633522044903279,
-3.314250214533));
#63302=CARTESIAN_POINT('Ctrl Pts',(0.5743279309632,-0.410493851410992,-3.2983636160386));
#63303=CARTESIAN_POINT('Ctrl Pts',(0.699214400400128,-0.0856105057499347,
-3.2824770175442));
#63304=CARTESIAN_POINT('Ctrl Pts',(0.643606290730907,0.376894711602609,
-3.26129488621835));
#63305=CARTESIAN_POINT('Ctrl Pts',(0.156311633013567,0.784886136552685,
-3.23481722206102));
#63306=CARTESIAN_POINT('Ctrl Pts',(-0.520643055030093,0.572945154878293,
-3.20549307517143));
#63307=CARTESIAN_POINT('Ctrl Pts',(-0.674669769920679,0.172521805840283,
-3.18675999394476));
#63308=CARTESIAN_POINT('Ctrl Pts',(-0.676187862115932,-0.000564937425030061,
-3.17861797838102));
#63309=CARTESIAN_POINT('Ctrl Pts',(-0.677150171393189,-0.000258134096645515,
-3.33918202161901));
#63310=CARTESIAN_POINT('Ctrl Pts',(-0.677354841532161,-0.0466576125141528,
-3.33700111102771));
#63311=CARTESIAN_POINT('Ctrl Pts',(-0.650453642473587,-0.318071380082664,
-3.32422913477348));
#63312=CARTESIAN_POINT('Ctrl Pts',(-0.28857304180409,-0.746461769625146,
-3.30086609285632));
#63313=CARTESIAN_POINT('Ctrl Pts',(0.473430607192205,-0.645985057580972,
-3.26909289586753));
#63314=CARTESIAN_POINT('Ctrl Pts',(0.742660672680755,-0.0686596397537776,
-3.24261523171021));
#63315=CARTESIAN_POINT('Ctrl Pts',(0.597361558428951,0.372009699145598,
-3.22143310038435));
#63316=CARTESIAN_POINT('Ctrl Pts',(0.264109646042611,0.698149366165507,
-3.2002509690585));
#63317=CARTESIAN_POINT('Ctrl Pts',(-0.242625816165684,0.705706516892486,
-3.17906883773263));
#63318=CARTESIAN_POINT('Ctrl Pts',(-0.586733693445035,0.38983774644249,
-3.15788670640678));
#63319=CARTESIAN_POINT('Ctrl Pts',(-0.671239753740077,0.152310487815706,
-3.14635627864606));
#63320=CARTESIAN_POINT('Ctrl Pts',(-0.676841484381597,0.0201564106724313,
-3.1401213837168));
#63321=CARTESIAN_POINT('Ctrl Pts',(-0.67679285177372,0.000237387877347905,
-3.13918202161901));
#63322=CARTESIAN_POINT('Origin',(0.,0.,-12.278617978381));
#63323=CARTESIAN_POINT('',(-0.6767,3.5083345969789E-13,-3.57861797838102));
#63324=CARTESIAN_POINT('',(-0.6765227315498,-4.29419654870256E-5,-3.53918202161901));
#63325=CARTESIAN_POINT('',(-0.6767,6.12423655037739E-13,-12.278617978381));
#63326=CARTESIAN_POINT('Ctrl Pts',(-0.6767,3.5083345969789E-13,-3.57861797838102));
#63327=CARTESIAN_POINT('Ctrl Pts',(-0.676700000000056,-0.10872516508436,
-3.57350370397235));
#63328=CARTESIAN_POINT('Ctrl Pts',(-0.649982596219497,-0.217427540192554,
-3.56838594349128));
#63329=CARTESIAN_POINT('Ctrl Pts',(-0.599548926342118,-0.313789698559424,
-3.56326992604641));
#63330=CARTESIAN_POINT('Ctrl Pts',(-0.508741893033908,-0.487292077937056,
-3.55405841382351));
#63331=CARTESIAN_POINT('Ctrl Pts',(-0.339068136092228,-0.617498730391311,
-3.5448469016006));
#63332=CARTESIAN_POINT('Ctrl Pts',(-0.147978738227961,-0.660322029794903,
-3.53563538937769));
#63333=CARTESIAN_POINT('Ctrl Pts',(0.0431106596363064,-0.703145329198496,
-3.52642387715479));
#63334=CARTESIAN_POINT('Ctrl Pts',(0.252125089209894,-0.657803027006444,
-3.51721236493188));
#63335=CARTESIAN_POINT('Ctrl Pts',(0.408292820688247,-0.539647906115122,
-3.50800085270897));
#63336=CARTESIAN_POINT('Ctrl Pts',(0.564460552166599,-0.421492785223799,
-3.49878934048607));
#63337=CARTESIAN_POINT('Ctrl Pts',(0.664928886611912,-0.232683172354559,
-3.48957782826316));
#63338=CARTESIAN_POINT('Ctrl Pts',(0.675679513260744,-0.0371495001275096,
-3.48036631604025));
#63339=CARTESIAN_POINT('Ctrl Pts',(0.686430139909577,0.15838417209954,-3.47115480381734));
#63340=CARTESIAN_POINT('Ctrl Pts',(0.607266678236122,0.357070111395513,
-3.46194329159444));
#63341=CARTESIAN_POINT('Ctrl Pts',(0.464993665761435,0.491633787286577,
-3.45273177937153));
#63342=CARTESIAN_POINT('Ctrl Pts',(0.322720653286747,0.626197463177641,
-3.44352026714862));
#63343=CARTESIAN_POINT('Ctrl Pts',(0.119936975630301,0.694180815655831,
-3.43430875492572));
#63344=CARTESIAN_POINT('Ctrl Pts',(-0.0746953534265867,0.672564862430738,
-3.42509724270281));
#63345=CARTESIAN_POINT('Ctrl Pts',(-0.269327682483474,0.650948909205645,
-3.4158857304799));
#63346=CARTESIAN_POINT('Ctrl Pts',(-0.452253335389412,0.540128506539963,
-3.406674218257));
#63347=CARTESIAN_POINT('Ctrl Pts',(-0.561534172714542,0.377627147956546,
-3.39746270603409));
#63348=CARTESIAN_POINT('Ctrl Pts',(-0.6360556905449,0.266813137124048,-3.39118113014973));
#63349=CARTESIAN_POINT('Ctrl Pts',(-0.676699999999928,0.133441673612206,
-3.38489488157883));
#63350=CARTESIAN_POINT('Ctrl Pts',(-0.6767,3.65423931474353E-13,-3.37861797838102));
#63351=CARTESIAN_POINT('Ctrl Pts',(-0.67538587901915,-0.000318336047294726,
-3.53918202161901));
#63352=CARTESIAN_POINT('Ctrl Pts',(-0.675554870863147,-0.113267255406579,
-3.53388083833862));
#63353=CARTESIAN_POINT('Ctrl Pts',(-0.595647073307492,-0.451514156200299,
-3.51798858939529));
#63354=CARTESIAN_POINT('Ctrl Pts',(-0.0573355312236082,-0.798840329041782,
-3.49150527478905));
#63355=CARTESIAN_POINT('Ctrl Pts',(0.521602160227078,-0.533094932750431,
-3.46502761063172));
#63356=CARTESIAN_POINT('Ctrl Pts',(0.696124873969488,-0.103161075934814,
-3.44384547930587));
#63357=CARTESIAN_POINT('Ctrl Pts',(0.653250630478223,0.361151016044349,
-3.42266334798001));
#63358=CARTESIAN_POINT('Ctrl Pts',(0.271913654699282,0.69494743617245,-3.40148121665415));
#63359=CARTESIAN_POINT('Ctrl Pts',(-0.194840623075141,0.676954228271529,
-3.38029908532829));
#63360=CARTESIAN_POINT('Ctrl Pts',(-0.495439723982,0.50288890843937,-3.36441248683389));
#63361=CARTESIAN_POINT('Ctrl Pts',(-0.649643514150033,0.245229588638644,
-3.3507067989308));
#63362=CARTESIAN_POINT('Ctrl Pts',(-0.676857875978016,0.0660063189202375,
-3.34229664385917));
#63363=CARTESIAN_POINT('Ctrl Pts',(-0.677150171393189,-0.000258134096645515,
-3.33918202161901));
#63364=CARTESIAN_POINT('Origin',(0.,0.,-12.278617978381));
#63365=CARTESIAN_POINT('',(-0.6767,3.36242987921428E-13,-3.77861797838102));
#63366=CARTESIAN_POINT('',(-0.6767,3.47884921894787E-13,-3.73918202161901));
#63367=CARTESIAN_POINT('',(-0.6767,6.12423655037739E-13,-12.278617978381));
#63368=CARTESIAN_POINT('Ctrl Pts',(-0.6767,3.36242987921428E-13,-3.77861797838102));
#63369=CARTESIAN_POINT('Ctrl Pts',(-0.676700000000077,-0.155057398273079,
-3.77132430277937));
#63370=CARTESIAN_POINT('Ctrl Pts',(-0.62127275025801,-0.309905500528333,
-3.76401378127864));
#63371=CARTESIAN_POINT('Ctrl Pts',(-0.522673846984314,-0.429808026540475,
-3.75671168272746));
#63372=CARTESIAN_POINT('Ctrl Pts',(-0.398292479586412,-0.581063665748294,
-3.74750017050455));
#63373=CARTESIAN_POINT('Ctrl Pts',(-0.205569794218462,-0.673804825341075,
-3.73828865828164));
#63374=CARTESIAN_POINT('Ctrl Pts',(-0.00976117943853978,-0.676629595403548,
-3.72907714605874));
#63375=CARTESIAN_POINT('Ctrl Pts',(0.186047435341383,-0.67945436546602,
-3.71986563383583));
#63376=CARTESIAN_POINT('Ctrl Pts',(0.38136516489873,-0.592311146231187,
-3.71065412161292));
#63377=CARTESIAN_POINT('Ctrl Pts',(0.510057945616593,-0.444706399901531,
-3.70144260939002));
#63378=CARTESIAN_POINT('Ctrl Pts',(0.638750726334456,-0.297101653571876,
-3.69223109716711));
#63379=CARTESIAN_POINT('Ctrl Pts',(0.698467741207415,-0.0917316599683544,
-3.6830195849442));
#63380=CARTESIAN_POINT('Ctrl Pts',(0.668988967866939,0.101865847428509,
-3.67380807272129));
#63381=CARTESIAN_POINT('Ctrl Pts',(0.639510194526462,0.295463354825373,
-3.66459656049839));
#63382=CARTESIAN_POINT('Ctrl Pts',(0.521374118513707,0.473751951438718,
-3.65538504827548));
#63383=CARTESIAN_POINT('Ctrl Pts',(0.354581300884681,0.576363592763221,
-3.64617353605258));
#63384=CARTESIAN_POINT('Ctrl Pts',(0.187788483255655,0.678975234087723,
-3.63696202382967));
#63385=CARTESIAN_POINT('Ctrl Pts',(-0.024614289760632,0.704035524449951,
-3.62775051160676));
#63386=CARTESIAN_POINT('Ctrl Pts',(-0.210708004284066,0.6430591162021,-3.61853899938385));
#63387=CARTESIAN_POINT('Ctrl Pts',(-0.3968017188075,0.582082707954249,-3.60932748716095));
#63388=CARTESIAN_POINT('Ctrl Pts',(-0.553187021228165,0.436183450502936,
-3.60011597493804));
#63389=CARTESIAN_POINT('Ctrl Pts',(-0.626912264184211,0.254762444279815,
-3.59090446271513));
#63390=CARTESIAN_POINT('Ctrl Pts',(-0.659690958955441,0.174101553251996,
-3.5868089679371));
#63391=CARTESIAN_POINT('Ctrl Pts',(-0.676699999999955,0.0870371046709928,
-3.58271207781673));
#63392=CARTESIAN_POINT('Ctrl Pts',(-0.6767,3.5083345969789E-13,-3.57861797838102));
#63393=CARTESIAN_POINT('Ctrl Pts',(-0.6767,3.47884921894787E-13,-3.73918202161901));
#63394=CARTESIAN_POINT('Ctrl Pts',(-0.676700000000037,-0.0715671495154181,
-3.73581560648426));
#63395=CARTESIAN_POINT('Ctrl Pts',(-0.665239533861194,-0.143202031285933,
-3.73244543791216));
#63396=CARTESIAN_POINT('Ctrl Pts',(-0.642887478847484,-0.211231104577724,
-3.72907714605874));
#63397=CARTESIAN_POINT('Ctrl Pts',(-0.581759691551794,-0.39727514927755,
-3.71986563383583));
#63398=CARTESIAN_POINT('Ctrl Pts',(-0.435733252864803,-0.553541701496641,
-3.71065412161292));
#63399=CARTESIAN_POINT('Ctrl Pts',(-0.254252326446219,-0.627119322375483,
-3.70144260939002));
#63400=CARTESIAN_POINT('Ctrl Pts',(-0.0727714000276362,-0.700696943254326,
-3.69223109716711));
#63401=CARTESIAN_POINT('Ctrl Pts',(0.140848921810412,-0.690241598407965,
-3.6830195849442));
#63402=CARTESIAN_POINT('Ctrl Pts',(0.314277366395853,-0.599293439786626,
-3.67380807272129));
#63403=CARTESIAN_POINT('Ctrl Pts',(0.487705810981295,-0.508345281165287,
-3.66459656049839));
#63404=CARTESIAN_POINT('Ctrl Pts',(0.617774379810403,-0.338565648874499,
-3.65538504827548));
#63405=CARTESIAN_POINT('Ctrl Pts',(0.660442201504015,-0.147441474736689,
-3.64617353605257));
#63406=CARTESIAN_POINT('Ctrl Pts',(0.703110023197628,0.0436826994011212,
-3.63696202382967));
#63407=CARTESIAN_POINT('Ctrl Pts',(0.657597689305156,0.252660170918286,
-3.62775051160676));
#63408=CARTESIAN_POINT('Ctrl Pts',(0.539315555004391,0.408731723909835,
-3.61853899938385));
#63409=CARTESIAN_POINT('Ctrl Pts',(0.421033420703626,0.564803276901384,
-3.60932748716095));
#63410=CARTESIAN_POINT('Ctrl Pts',(0.232142132856037,0.665117969311451,
-3.60011597493804));
#63411=CARTESIAN_POINT('Ctrl Pts',(0.0365997790121158,0.675709513160992,
-3.59090446271513));
#63412=CARTESIAN_POINT('Ctrl Pts',(-0.158942574831805,0.686301057010532,
-3.58169295049223));
#63413=CARTESIAN_POINT('Ctrl Pts',(-0.357564043797021,0.606975977721903,
-3.57248143826932));
#63414=CARTESIAN_POINT('Ctrl Pts',(-0.492011926892181,0.464593536110699,
-3.56326992604641));
#63415=CARTESIAN_POINT('Ctrl Pts',(-0.609204691775011,0.340484538489852,
-3.55524062457061));
#63416=CARTESIAN_POINT('Ctrl Pts',(-0.676699999999909,0.170493761108641,
-3.5472018013875));
#63417=CARTESIAN_POINT('Ctrl Pts',(-0.6767,3.6247539367125E-13,-3.53918202161901));
#63418=CARTESIAN_POINT('Origin',(0.,0.,-12.278617978381));
#63419=CARTESIAN_POINT('',(-0.6767,3.60118402112364E-13,-3.97861797838102));
#63420=CARTESIAN_POINT('',(-0.67777021896946,-0.000635695144750592,-3.93918202161901));
#63421=CARTESIAN_POINT('',(-0.6767,6.12423655037739E-13,-12.278617978381));
#63422=CARTESIAN_POINT('Ctrl Pts',(-0.676398488294932,-0.000408318744697735,
-3.97861797838102));
#63423=CARTESIAN_POINT('Ctrl Pts',(-0.67634238392664,-0.0927455508296921,
-3.97427890318839));
#63424=CARTESIAN_POINT('Ctrl Pts',(-0.634908478920628,-0.297096589374643,
-3.9646442951643));
#63425=CARTESIAN_POINT('Ctrl Pts',(-0.433764682453468,-0.555047868816476,
-3.94971415430875));
#63426=CARTESIAN_POINT('Ctrl Pts',(-0.00876936604903183,-0.745789366591879,
-3.92853202298289));
#63427=CARTESIAN_POINT('Ctrl Pts',(0.592020032873446,-0.538508917887617,
-3.90205435882556));
#63428=CARTESIAN_POINT('Ctrl Pts',(0.773304882718845,0.208405356954825,
-3.87028116183678));
#63429=CARTESIAN_POINT('Ctrl Pts',(0.332043120165925,0.667837096325308,
-3.84380349767945));
#63430=CARTESIAN_POINT('Ctrl Pts',(-0.13136609001657,0.691357359215059,
-3.82262136635359));
#63431=CARTESIAN_POINT('Ctrl Pts',(-0.531370482730002,0.50936984768987,
-3.80265803753127));
#63432=CARTESIAN_POINT('Ctrl Pts',(-0.67533931475917,0.198712628292847,
-3.78799024154041));
#63433=CARTESIAN_POINT('Ctrl Pts',(-0.677056267769222,-2.7870685577195E-5,
-3.77861797838102));
#63434=CARTESIAN_POINT('Ctrl Pts',(-0.67777021896946,-0.000635695144750609,
-3.93918202161901));
#63435=CARTESIAN_POINT('Ctrl Pts',(-0.677903959863105,-0.0207744172333184,
-3.93823135862336));
#63436=CARTESIAN_POINT('Ctrl Pts',(-0.667985189522564,-0.265075498201874,
-3.92668962996479));
#63437=CARTESIAN_POINT('Ctrl Pts',(-0.441632977912428,-0.601015252466975,
-3.90985236847475));
#63438=CARTESIAN_POINT('Ctrl Pts',(0.0108809088601417,-0.703643129412517,
-3.88867023714889));
#63439=CARTESIAN_POINT('Ctrl Pts',(0.462129679432592,-0.586176255061214,
-3.86748810582303));
#63440=CARTESIAN_POINT('Ctrl Pts',(0.729797145596839,-0.15583677657501,
-3.84630597449717));
#63441=CARTESIAN_POINT('Ctrl Pts',(0.636487863470664,0.301849457891777,
-3.82512384317132));
#63442=CARTESIAN_POINT('Ctrl Pts',(0.416060211528914,0.570308403158517,
-3.80923724467692));
#63443=CARTESIAN_POINT('Ctrl Pts',(0.0924068473382293,0.698348703003505,
-3.79335064618252));
#63444=CARTESIAN_POINT('Ctrl Pts',(-0.370617326288914,0.647241437607997,
-3.77216851485667));
#63445=CARTESIAN_POINT('Ctrl Pts',(-0.65206223079829,0.317656845722991,
-3.75411230666883));
#63446=CARTESIAN_POINT('Ctrl Pts',(-0.67730862690677,0.0470558304535615,
-3.74135163131245));
#63447=CARTESIAN_POINT('Ctrl Pts',(-0.676873778127171,0.000939313808043477,
-3.739182021619));
#63448=CARTESIAN_POINT('Origin',(0.,0.,-12.278617978381));
#63449=CARTESIAN_POINT('',(-0.6767,3.07062044368503E-13,-4.17861797838102));
#63450=CARTESIAN_POINT('',(-0.675428755222163,-0.000265590320332854,-4.13918202161901));
#63451=CARTESIAN_POINT('',(-0.6767,6.12423655037739E-13,-12.278617978381));
#63452=CARTESIAN_POINT('Ctrl Pts',(-0.6767,3.26295015140058E-13,-4.17861797838102));
#63453=CARTESIAN_POINT('Ctrl Pts',(-0.676700000000025,-0.0523060661812641,
-4.17615757672992));
#63454=CARTESIAN_POINT('Ctrl Pts',(-0.670596734023588,-0.10470939197741,
-4.17369248129918));
#63455=CARTESIAN_POINT('Ctrl Pts',(-0.658553289072125,-0.15566134861386,
-4.17122973275826));
#63456=CARTESIAN_POINT('Ctrl Pts',(-0.613506732944653,-0.346238893799521,
-4.16201822053536));
#63457=CARTESIAN_POINT('Ctrl Pts',(-0.481332242759297,-0.514384248425477,
-4.15280670831245));
#63458=CARTESIAN_POINT('Ctrl Pts',(-0.306783749263979,-0.603163842738883,
-4.14359519608954));
#63459=CARTESIAN_POINT('Ctrl Pts',(-0.132235255768667,-0.691943437052286,
-4.13438368386664));
#63460=CARTESIAN_POINT('Ctrl Pts',(0.0814987827214579,-0.699735543875582,
-4.12517217164373));
#63461=CARTESIAN_POINT('Ctrl Pts',(0.262048589378461,-0.623901776568042,
-4.11596065942082));
#63462=CARTESIAN_POINT('Ctrl Pts',(0.442598396035471,-0.548068009260499,
-4.10674914719792));
#63463=CARTESIAN_POINT('Ctrl Pts',(0.586665887210476,-0.389993614988096,
-4.09753763497501));
#63464=CARTESIAN_POINT('Ctrl Pts',(0.645470193659864,-0.203202163120125,
-4.0883261227521));
#63465=CARTESIAN_POINT('Ctrl Pts',(0.704274500109252,-0.0164107112521548,
-4.0791146105292));
#63466=CARTESIAN_POINT('Ctrl Pts',(0.676741449973327,0.195685699109407,
-4.06990309830629));
#63467=CARTESIAN_POINT('Ctrl Pts',(0.572193660780889,0.361271787664308,
-4.06069158608338));
#63468=CARTESIAN_POINT('Ctrl Pts',(0.467645871588451,0.526857876219209,
-4.05148007386048));
#63469=CARTESIAN_POINT('Ctrl Pts',(0.287993106415111,0.642908899926974,
-4.04226856163757));
#63470=CARTESIAN_POINT('Ctrl Pts',(0.0940653136114567,0.67013029089512,
-4.03305704941466));
#63471=CARTESIAN_POINT('Ctrl Pts',(-0.0998624791921981,0.697351681863266,
-4.02384553719176));
#63472=CARTESIAN_POINT('Ctrl Pts',(-0.304522841761762,0.63524618990851,
-4.01463402496885));
#63473=CARTESIAN_POINT('Ctrl Pts',(-0.450618319796951,0.504842569385123,
-4.00542251274594));
#63474=CARTESIAN_POINT('Ctrl Pts',(-0.592325825462736,0.378355616861474,
-3.99648766795763));
#63475=CARTESIAN_POINT('Ctrl Pts',(-0.676699999999899,0.189857389572419,
-3.98754859520765));
#63476=CARTESIAN_POINT('Ctrl Pts',(-0.6767,3.60118457688074E-13,-3.97861797838102));
#63477=CARTESIAN_POINT('Ctrl Pts',(-0.675428755222163,-0.00026559032033293,
-4.13918202161901));
#63478=CARTESIAN_POINT('Ctrl Pts',(-0.675756229953581,-0.0870463508529104,
-4.13511108593427));
#63479=CARTESIAN_POINT('Ctrl Pts',(-0.639962042678306,-0.286443286036591,
-4.12574461741807));
#63480=CARTESIAN_POINT('Ctrl Pts',(-0.447211755898116,-0.54335411393822,
-4.1110826160704));
#63481=CARTESIAN_POINT('Ctrl Pts',(-0.027231621354319,-0.745938926057937,
-4.08990048474455));
#63482=CARTESIAN_POINT('Ctrl Pts',(0.455363367272391,-0.591213310405756,
-4.06871835341868));
#63483=CARTESIAN_POINT('Ctrl Pts',(0.680528182180706,-0.181965075860278,
-4.04753622209283));
#63484=CARTESIAN_POINT('Ctrl Pts',(0.686307798878026,0.165346241353982,
-4.03164962359843));
#63485=CARTESIAN_POINT('Ctrl Pts',(0.522509375349723,0.472455171517164,
-4.01576302510404));
#63486=CARTESIAN_POINT('Ctrl Pts',(0.136512190381233,0.733241503857858,
-3.99458089377818));
#63487=CARTESIAN_POINT('Ctrl Pts',(-0.468392871864562,0.635675212224839,
-3.9690538926165));
#63488=CARTESIAN_POINT('Ctrl Pts',(-0.676413990659613,0.20358534956571,
-3.94882242428629));
#63489=CARTESIAN_POINT('Ctrl Pts',(-0.67777021896946,-0.000635695144750609,
-3.93918202161901));
#63490=CARTESIAN_POINT('Origin',(0.,0.,-12.278617978381));
#63491=CARTESIAN_POINT('',(-0.677441199567872,5.70499087820638E-6,-4.37861797838101));
#63492=CARTESIAN_POINT('',(-0.676588893509693,0.000498966854468069,-4.33918202161901));
#63493=CARTESIAN_POINT('',(-0.6767,6.12423655037739E-13,-12.278617978381));
#63494=CARTESIAN_POINT('Ctrl Pts',(-0.677441199567871,5.70499087820063E-6,
-4.37861797838102));
#63495=CARTESIAN_POINT('Ctrl Pts',(-0.676753222916443,-0.224413153492785,
-4.36803835781021));
#63496=CARTESIAN_POINT('Ctrl Pts',(-0.435300975903498,-0.67140171353152,
-4.34686767157647));
#63497=CARTESIAN_POINT('Ctrl Pts',(0.33083155171032,-0.729372140157004,
-4.3151059196798));
#63498=CARTESIAN_POINT('Ctrl Pts',(0.712777470420673,-0.219561605337653,
-4.28862825552248));
#63499=CARTESIAN_POINT('Ctrl Pts',(0.660975650409514,0.241543448084987,
-4.26744612419662));
#63500=CARTESIAN_POINT('Ctrl Pts',(0.401722358340205,0.629114925446567,
-4.24626399287076));
#63501=CARTESIAN_POINT('Ctrl Pts',(-0.0926839103114625,0.74047192210371,
-4.2250818615449));
#63502=CARTESIAN_POINT('Ctrl Pts',(-0.494275113109166,0.50191832815303,
-4.20389973021904));
#63503=CARTESIAN_POINT('Ctrl Pts',(-0.650705510793311,0.245875025282787,
-4.1901769467749));
#63504=CARTESIAN_POINT('Ctrl Pts',(-0.676474114823456,0.0669674968791263,
-4.18174969616223));
#63505=CARTESIAN_POINT('Ctrl Pts',(-0.676399342971297,0.000375592675570233,
-4.17861797838102));
#63506=CARTESIAN_POINT('Ctrl Pts',(-0.676588893509694,0.000498966854468048,
-4.33918202161901));
#63507=CARTESIAN_POINT('Ctrl Pts',(-0.676405822493527,-0.0398360353532038,
-4.33728634607665));
#63508=CARTESIAN_POINT('Ctrl Pts',(-0.662272900657128,-0.193056914041967,
-4.33009513770282));
#63509=CARTESIAN_POINT('Ctrl Pts',(-0.503641062853606,-0.550919342933017,
-4.31231286366604));
#63510=CARTESIAN_POINT('Ctrl Pts',(-0.0356495923251104,-0.745397934811761,
-4.29113073234021));
#63511=CARTESIAN_POINT('Ctrl Pts',(0.400896797976255,-0.579233677324962,
-4.26994860101433));
#63512=CARTESIAN_POINT('Ctrl Pts',(0.630134791455414,-0.318257629803494,
-4.25406200251995));
#63513=CARTESIAN_POINT('Ctrl Pts',(0.704096847355287,0.0218532827285811,
-4.23817540402554));
#63514=CARTESIAN_POINT('Ctrl Pts',(0.578714001944864,0.47049844320186,-4.21699327269969));
#63515=CARTESIAN_POINT('Ctrl Pts',(0.0349786870852126,0.799534905690655,
-4.19051560854237));
#63516=CARTESIAN_POINT('Ctrl Pts',(-0.566591317156505,0.504275578643712,
-4.16281334723832));
#63517=CARTESIAN_POINT('Ctrl Pts',(-0.674904262088699,0.138725020708031,
-4.1457021515972));
#63518=CARTESIAN_POINT('Ctrl Pts',(-0.675428755222163,-0.00026559032033293,
-4.13918202161901));
#63519=CARTESIAN_POINT('Origin',(0.,0.,-12.278617978381));
#63520=CARTESIAN_POINT('',(-0.6767,2.77881016808035E-13,-4.57861797838101));
#63521=CARTESIAN_POINT('',(-0.677483499338122,-0.000155519670934575,-4.539182021619));
#63522=CARTESIAN_POINT('',(-0.6767,6.12423655037739E-13,-12.278617978381));
#63523=CARTESIAN_POINT('Ctrl Pts',(-0.676332918879227,-0.000635712003939359,
-4.57861797838102));
#63524=CARTESIAN_POINT('Ctrl Pts',(-0.676955652671927,-0.0666551245079565,
-4.57550915078405));
#63525=CARTESIAN_POINT('Ctrl Pts',(-0.637892478859078,-0.356991836088987,
-4.56180925752415));
#63526=CARTESIAN_POINT('Ctrl Pts',(-0.220004051678502,-0.770085353509153,
-4.5375182986013));
#63527=CARTESIAN_POINT('Ctrl Pts',(0.401138704855467,-0.628766061699122,
-4.51104063444399));
#63528=CARTESIAN_POINT('Ctrl Pts',(0.660153306932357,-0.243781990912655,
-4.48985850311813));
#63529=CARTESIAN_POINT('Ctrl Pts',(0.713448163538854,0.21944967658462,-4.46867637179228));
#63530=CARTESIAN_POINT('Ctrl Pts',(0.408703467624615,0.624380052697233,
-4.44749424046641));
#63531=CARTESIAN_POINT('Ctrl Pts',(-0.0518139061167167,0.702527732340824,
-4.42631210914056));
#63532=CARTESIAN_POINT('Ctrl Pts',(-0.381729763931295,0.593835130031606,
-4.41042551064616));
#63533=CARTESIAN_POINT('Ctrl Pts',(-0.617941327913625,0.338198834530834,
-4.39453891215177));
#63534=CARTESIAN_POINT('Ctrl Pts',(-0.67772194426544,0.112822645438229,
-4.38393640139672));
#63535=CARTESIAN_POINT('Ctrl Pts',(-0.677441943824823,0.000248482554735446,
-4.37862942347313));
#63536=CARTESIAN_POINT('Ctrl Pts',(-0.677441199567871,5.70499087820063E-6,
-4.37861797838102));
#63537=CARTESIAN_POINT('Ctrl Pts',(-0.677483499338121,-0.000155519670934546,
-4.539182021619));
#63538=CARTESIAN_POINT('Ctrl Pts',(-0.67666748440995,-0.218510581706608,
-4.52887054055609));
#63539=CARTESIAN_POINT('Ctrl Pts',(-0.503895417062598,-0.547116013156695,
-4.5132635266617));
#63540=CARTESIAN_POINT('Ctrl Pts',(-0.0694084667398682,-0.701008102891709,
-4.49236097993585));
#63541=CARTESIAN_POINT('Ctrl Pts',(0.274258103338072,-0.650492326691175,
-4.47647438144146));
#63542=CARTESIAN_POINT('Ctrl Pts',(0.550802926396446,-0.439142428711666,
-4.46058778294706));
#63543=CARTESIAN_POINT('Ctrl Pts',(0.745668804766385,-0.0160223188298255,
-4.4394056516212));
#63544=CARTESIAN_POINT('Ctrl Pts',(0.544241292482002,0.586754624630679,
-4.41292798746388));
#63545=CARTESIAN_POINT('Ctrl Pts',(-0.200874523336002,0.775295208497259,
-4.3811547904751));
#63546=CARTESIAN_POINT('Ctrl Pts',(-0.63137729592835,0.369793488861541,
-4.35657280186013));
#63547=CARTESIAN_POINT('Ctrl Pts',(-0.676917227823677,0.0728390103888557,
-4.34258187890811));
#63548=CARTESIAN_POINT('Ctrl Pts',(-0.676588893509694,0.000498966854468048,
-4.33918202161901));
#63549=CARTESIAN_POINT('Origin',(0.,0.,-12.278617978381));
#63550=CARTESIAN_POINT('',(-0.676672460315546,1.17798547158296E-5,-4.77861797838102));
#63551=CARTESIAN_POINT('',(-0.6767,2.94165516598333E-13,-4.739182021619));
#63552=CARTESIAN_POINT('',(-0.6767,6.12423655037739E-13,-12.278617978381));
#63553=CARTESIAN_POINT('Ctrl Pts',(-0.6767,2.8252359981067E-13,-4.77861797838101));
#63554=CARTESIAN_POINT('Ctrl Pts',(-0.67670000000008,-0.191713242581063,
-4.76960006491478));
#63555=CARTESIAN_POINT('Ctrl Pts',(-0.590610559833386,-0.381943871873007,
-4.76057599466127));
#63556=CARTESIAN_POINT('Ctrl Pts',(-0.446504609572047,-0.508484536275111,
-4.75155500280139));
#63557=CARTESIAN_POINT('Ctrl Pts',(-0.299355189325865,-0.637697697637065,
-4.74234349057849));
#63558=CARTESIAN_POINT('Ctrl Pts',(-0.0941973328990827,-0.698139488514034,
-4.73313197835558));
#63559=CARTESIAN_POINT('Ctrl Pts',(0.0995030553114643,-0.669344479310679,
-4.72392046613267));
#63560=CARTESIAN_POINT('Ctrl Pts',(0.293203443522011,-0.640549470107323,
-4.71470895390977));
#63561=CARTESIAN_POINT('Ctrl Pts',(0.471908059626845,-0.523043656119796,
-4.70549744168686));
#63562=CARTESIAN_POINT('Ctrl Pts',(0.575107996027578,-0.356614193359074,
-4.69628592946395));
#63563=CARTESIAN_POINT('Ctrl Pts',(0.678307932428311,-0.190184730598352,
-4.68707441724105));
#63564=CARTESIAN_POINT('Ctrl Pts',(0.704118047129442,0.0221282320703506,
-4.67786290501814));
#63565=CARTESIAN_POINT('Ctrl Pts',(0.6437991039568,0.208436090311686,-4.66865139279523));
#63566=CARTESIAN_POINT('Ctrl Pts',(0.583480160784159,0.394743948553022,
-4.65943988057233));
#63567=CARTESIAN_POINT('Ctrl Pts',(0.438133999301458,0.551643437017108,
-4.65022836834942));
#63568=CARTESIAN_POINT('Ctrl Pts',(0.256974443116801,0.626008806315702,
-4.64101685612651));
#63569=CARTESIAN_POINT('Ctrl Pts',(0.0758148869321448,0.700374175614296,
-4.63180534390361));
#63570=CARTESIAN_POINT('Ctrl Pts',(-0.137848842077393,0.690847001647876,
-4.6225938316807));
#63571=CARTESIAN_POINT('Ctrl Pts',(-0.311670773686952,0.600653160175968,
-4.61338231945779));
#63572=CARTESIAN_POINT('Ctrl Pts',(-0.485492705296511,0.51045931870406,
-4.60417080723489));
#63573=CARTESIAN_POINT('Ctrl Pts',(-0.616297653217761,0.341246370803001,
-4.59495929501198));
#63574=CARTESIAN_POINT('Ctrl Pts',(-0.659795410069959,0.150309370468427,
-4.58574778278907));
#63575=CARTESIAN_POINT('Ctrl Pts',(-0.671017979214619,0.101046975264696,
-4.58337118131972));
#63576=CARTESIAN_POINT('Ctrl Pts',(-0.676699999999979,0.0504745568557825,
-4.58099222848414));
#63577=CARTESIAN_POINT('Ctrl Pts',(-0.6767,2.77881100815578E-13,-4.57861797838101));
#63578=CARTESIAN_POINT('Ctrl Pts',(-0.676059626651951,-0.000187573017024642,
-4.739182021619));
#63579=CARTESIAN_POINT('Ctrl Pts',(-0.676604188211727,-0.0605326678519595,
-4.73634133352992));
#63580=CARTESIAN_POINT('Ctrl Pts',(-0.655486634525628,-0.233258944214111,
-4.72820511260937));
#63581=CARTESIAN_POINT('Ctrl Pts',(-0.506701789827963,-0.489370199092825,
-4.71477335885737));
#63582=CARTESIAN_POINT('Ctrl Pts',(-0.212060776109364,-0.673340925212919,
-4.69888676036297));
#63583=CARTESIAN_POINT('Ctrl Pts',(0.13553701687756,-0.691273935193279,
-4.68300016186857));
#63584=CARTESIAN_POINT('Ctrl Pts',(0.557969828113902,-0.494922571739213,
-4.66181803054273));
#63585=CARTESIAN_POINT('Ctrl Pts',(0.794652742927993,0.0949030669946144,
-4.63534036638539));
#63586=CARTESIAN_POINT('Ctrl Pts',(0.348784514783706,0.720959497261372,
-4.6035671693966));
#63587=CARTESIAN_POINT('Ctrl Pts',(-0.287390379613016,0.68823381970347,
-4.57708950523929));
#63588=CARTESIAN_POINT('Ctrl Pts',(-0.608578462087337,0.353361434271592,
-4.55590737391342));
#63589=CARTESIAN_POINT('Ctrl Pts',(-0.676285382095685,0.123841442227276,
-4.54503672365049));
#63590=CARTESIAN_POINT('Ctrl Pts',(-0.677505624695856,0.00576494047506343,
-4.53946160621901));
#63591=CARTESIAN_POINT('Ctrl Pts',(-0.677483499338121,-0.000155519670934546,
-4.539182021619));
#63592=CARTESIAN_POINT('Origin',(0.,0.,-12.278617978381));
#63593=CARTESIAN_POINT('',(-0.677644860324165,0.000269891732193889,-4.97861797838101));
#63594=CARTESIAN_POINT('',(-0.6767,2.60342091236013E-13,-4.939182021619));
#63595=CARTESIAN_POINT('',(-0.6767,6.12423655037739E-13,-12.278617978381));
#63596=CARTESIAN_POINT('Ctrl Pts',(-0.677644860324165,0.000269891732193914,
-4.97861797838101));
#63597=CARTESIAN_POINT('Ctrl Pts',(-0.675978634032105,-0.197648105273453,
-4.96926860540586));
#63598=CARTESIAN_POINT('Ctrl Pts',(-0.530813983809632,-0.508956833739578,
-4.95462369959923));
#63599=CARTESIAN_POINT('Ctrl Pts',(-0.133708223738798,-0.690908212899286,
-4.93468326096116));
#63600=CARTESIAN_POINT('Ctrl Pts',(0.332041232394348,-0.668517062310377,
-4.91350112963529));
#63601=CARTESIAN_POINT('Ctrl Pts',(0.682302518044435,-0.302245344918345,
-4.89231899830944));
#63602=CARTESIAN_POINT('Ctrl Pts',(0.684875796890799,0.164848531713828,
-4.87113686698358));
#63603=CARTESIAN_POINT('Ctrl Pts',(0.524213242357612,0.472819469636789,
-4.85525026848919));
#63604=CARTESIAN_POINT('Ctrl Pts',(0.23371275114266,0.664536143768718,-4.83936366999479));
#63605=CARTESIAN_POINT('Ctrl Pts',(-0.229947459772284,0.709508877214857,
-4.81818153866894));
#63606=CARTESIAN_POINT('Ctrl Pts',(-0.614678118223211,0.412519780986417,
-4.79793297479767));
#63607=CARTESIAN_POINT('Ctrl Pts',(-0.676025351084611,0.0936457920984287,
-4.78297994375788));
#63608=CARTESIAN_POINT('Ctrl Pts',(-0.675657090930862,0.000446095054207521,
-4.77861797838102));
#63609=CARTESIAN_POINT('Ctrl Pts',(-0.6767,2.60342091236013E-13,-4.939182021619));
#63610=CARTESIAN_POINT('Ctrl Pts',(-0.676700000000059,-0.154446373905746,
-4.93191708771927));
#63611=CARTESIAN_POINT('Ctrl Pts',(-0.6217245569102,-0.30869061553757,-4.92463548908214));
#63612=CARTESIAN_POINT('Ctrl Pts',(-0.523839866944655,-0.428386138663947,
-4.91736222281372));
#63613=CARTESIAN_POINT('Ctrl Pts',(-0.399869977107543,-0.579979210279085,
-4.90815071059081));
#63614=CARTESIAN_POINT('Ctrl Pts',(-0.207400015820569,-0.673243727327307,
-4.8989391983679));
#63615=CARTESIAN_POINT('Ctrl Pts',(-0.0115997999403209,-0.676600572451239,
-4.889727686145));
#63616=CARTESIAN_POINT('Ctrl Pts',(0.184200415939927,-0.679957417575171,
-4.88051617392209));
#63617=CARTESIAN_POINT('Ctrl Pts',(0.379754225200688,-0.593345271650633,
-4.87130466169918));
#63618=CARTESIAN_POINT('Ctrl Pts',(0.508847628265527,-0.446090776870076,
-4.86209314947628));
#63619=CARTESIAN_POINT('Ctrl Pts',(0.637941031330366,-0.29883628208952,
-4.85288163725337));
#63620=CARTESIAN_POINT('Ctrl Pts',(0.698215893069096,-0.0936293202670115,
-4.84367012503046));
#63621=CARTESIAN_POINT('Ctrl Pts',(0.669263305648498,0.100047577244257,
-4.83445861280756));
#63622=CARTESIAN_POINT('Ctrl Pts',(0.640310718227899,0.293724474755526,
-4.82524710058465));
#63623=CARTESIAN_POINT('Ctrl Pts',(0.522659555408253,0.472333433168122,
-4.81603558836174));
#63624=CARTESIAN_POINT('Ctrl Pts',(0.356146187928414,0.575397934323768,
-4.80682407613883));
#63625=CARTESIAN_POINT('Ctrl Pts',(0.189632820448575,0.678462435479413,
-4.79761256391593));
#63626=CARTESIAN_POINT('Ctrl Pts',(-0.0227010701478788,0.704099811363474,
-4.78840105169302));
#63627=CARTESIAN_POINT('Ctrl Pts',(-0.208959793384939,0.643629314705696,
-4.77918953947011));
#63628=CARTESIAN_POINT('Ctrl Pts',(-0.395218516621998,0.583158818047918,
-4.76997802724721));
#63629=CARTESIAN_POINT('Ctrl Pts',(-0.551999704693553,0.437685056823018,
-4.7607665150243));
#63630=CARTESIAN_POINT('Ctrl Pts',(-0.62621766440955,0.256465059572349,
-4.75155500280139));
#63631=CARTESIAN_POINT('Ctrl Pts',(-0.659447728295543,0.175326314865503,
-4.7474306757406));
#63632=CARTESIAN_POINT('Ctrl Pts',(-0.676699999999962,0.087650303709258,
-4.74330496505));
#63633=CARTESIAN_POINT('Ctrl Pts',(-0.6767,2.9416553378403E-13,-4.739182021619));
#63634=CARTESIAN_POINT('Origin',(0.,0.,-12.278617978381));
#63635=CARTESIAN_POINT('',(-0.676546632405414,-0.000558781037866288,-5.17861797838101));
#63636=CARTESIAN_POINT('',(-0.676681193656348,0.000319961310848924,-5.139182021619));
#63637=CARTESIAN_POINT('',(-0.6767,6.12423655037739E-13,-12.278617978381));
#63638=CARTESIAN_POINT('Ctrl Pts',(-0.676546632405414,-0.000558781037866309,
-5.17861797838101));
#63639=CARTESIAN_POINT('Ctrl Pts',(-0.676910944207348,-0.0404440489505496,
-5.1767393983797));
#63640=CARTESIAN_POINT('Ctrl Pts',(-0.664788307948526,-0.192568022435409,
-5.16956528554692));
#63641=CARTESIAN_POINT('Ctrl Pts',(-0.549172285849032,-0.440047552208631,
-5.15709563988267));
#63642=CARTESIAN_POINT('Ctrl Pts',(-0.179687362077751,-0.724485261766983,
-5.1359135085568));
#63643=CARTESIAN_POINT('Ctrl Pts',(0.324385456870523,-0.67205881440986,
-5.11473137723096));
#63644=CARTESIAN_POINT('Ctrl Pts',(0.628721139150488,-0.317709969564103,
-5.09354924590509));
#63645=CARTESIAN_POINT('Ctrl Pts',(0.705631348411274,0.0210279449736901,
-5.0776626474107));
#63646=CARTESIAN_POINT('Ctrl Pts',(0.608322795378933,0.355208830188862,
-5.0617760489163));
#63647=CARTESIAN_POINT('Ctrl Pts',(0.284038448676206,0.689638195560499,
-5.04059391759044));
#63648=CARTESIAN_POINT('Ctrl Pts',(-0.350809927077043,0.719313540142401,
-5.01411625343312));
#63649=CARTESIAN_POINT('Ctrl Pts',(-0.664677743479125,0.276906197068003,
-4.99169242941949));
#63650=CARTESIAN_POINT('Ctrl Pts',(-0.677866152276955,0.0265554330528713,
-4.97985967106879));
#63651=CARTESIAN_POINT('Ctrl Pts',(-0.677644860324165,0.000269891732193914,
-4.97861797838101));
#63652=CARTESIAN_POINT('Ctrl Pts',(-0.676681193656349,0.000319961310848927,
-5.139182021619));
#63653=CARTESIAN_POINT('Ctrl Pts',(-0.676458674215642,-0.0800116306119912,
-5.1353963209832));
#63654=CARTESIAN_POINT('Ctrl Pts',(-0.641533144143856,-0.273093713028534,
-5.12631508751594));
#63655=CARTESIAN_POINT('Ctrl Pts',(-0.398077205723047,-0.630724360863014,
-5.10664278838574));
#63656=CARTESIAN_POINT('Ctrl Pts',(0.222281684997194,-0.768811047320993,
-5.08016512422842));
#63657=CARTESIAN_POINT('Ctrl Pts',(0.767909224957921,-0.227483310747878,
-5.04839192723964));
#63658=CARTESIAN_POINT('Ctrl Pts',(0.632637701696453,0.39500450537932,-5.0219142630823));
#63659=CARTESIAN_POINT('Ctrl Pts',(0.250190952797296,0.657751119258226,
-5.00073213175645));
#63660=CARTESIAN_POINT('Ctrl Pts',(-0.212500472627088,0.715548734708769,
-4.97955000043058));
#63661=CARTESIAN_POINT('Ctrl Pts',(-0.607562341949752,0.424205965160257,
-4.95903329705144));
#63662=CARTESIAN_POINT('Ctrl Pts',(-0.676723613838758,0.098630709613695,
-4.94381212650376));
#63663=CARTESIAN_POINT('Ctrl Pts',(-0.676504186696694,-0.000135632411926398,
-4.939182021619));
#63664=CARTESIAN_POINT('Origin',(0.,0.,-12.278617978381));
#63665=CARTESIAN_POINT('',(-0.6767,2.19519227014769E-13,-5.37861797838101));
#63666=CARTESIAN_POINT('',(-0.677314241554135,-0.00024113045791524,-5.339182021619));
#63667=CARTESIAN_POINT('',(-0.6767,6.12423655037739E-13,-12.278617978381));
#63668=CARTESIAN_POINT('Ctrl Pts',(-0.676213525726746,6.46560819233264E-5,
-5.37861797838101));
#63669=CARTESIAN_POINT('Ctrl Pts',(-0.67625358434725,-0.106616645045719,
-5.3736191256906));
#63670=CARTESIAN_POINT('Ctrl Pts',(-0.600096841340238,-0.439885678167944,
-5.35802920733728));
#63671=CARTESIAN_POINT('Ctrl Pts',(-0.187815285885199,-0.722228768117197,
-5.33714375615245));
#63672=CARTESIAN_POINT('Ctrl Pts',(0.273535159807509,-0.649159773727578,
-5.31596162482661));
#63673=CARTESIAN_POINT('Ctrl Pts',(0.551438224564908,-0.44076485660649,
-5.3000750263322));
#63674=CARTESIAN_POINT('Ctrl Pts',(0.693603344904396,-0.123062327230168,
-5.28418842783782));
#63675=CARTESIAN_POINT('Ctrl Pts',(0.662930453897055,0.341762921281637,
-5.26300629651195));
#63676=CARTESIAN_POINT('Ctrl Pts',(0.198265258367223,0.775351830664549,
-5.23652863235464));
#63677=CARTESIAN_POINT('Ctrl Pts',(-0.502472826500339,0.596687001070201,
-5.20663401536716));
#63678=CARTESIAN_POINT('Ctrl Pts',(-0.67485702570861,0.184421270147124,
-5.18733046404262));
#63679=CARTESIAN_POINT('Ctrl Pts',(-0.676546632405414,-0.000558781037866309,
-5.17861797838101));
#63680=CARTESIAN_POINT('Ctrl Pts',(-0.677314241554135,-0.000241130457915198,
-5.339182021619));
#63681=CARTESIAN_POINT('Ctrl Pts',(-0.677442214828523,-0.0344734714592605,
-5.33757158112557));
#63682=CARTESIAN_POINT('Ctrl Pts',(-0.658345400178551,-0.293576636578878,
-5.32537007496922));
#63683=CARTESIAN_POINT('Ctrl Pts',(-0.328270635324783,-0.729875307140714,
-5.30257750314993));
#63684=CARTESIAN_POINT('Ctrl Pts',(0.438031486668258,-0.670493587687057,
-5.27080430616114));
#63685=CARTESIAN_POINT('Ctrl Pts',(0.737897769931333,-0.108470742618401,
-5.24432664200382));
#63686=CARTESIAN_POINT('Ctrl Pts',(0.616490027294739,0.339370143052669,
-5.22314451067796));
#63687=CARTESIAN_POINT('Ctrl Pts',(0.301246298432971,0.682947370072152,
-5.2019623793521));
#63688=CARTESIAN_POINT('Ctrl Pts',(-0.204350803094626,0.717725381973961,
-5.18078024802625));
#63689=CARTESIAN_POINT('Ctrl Pts',(-0.564936112187733,0.420805281242191,
-5.15959811670039));
#63690=CARTESIAN_POINT('Ctrl Pts',(-0.666891133314686,0.176652537412118,
-5.14749721884179));
#63691=CARTESIAN_POINT('Ctrl Pts',(-0.676769939980493,0.0323582114215476,
-5.14069185381466));
#63692=CARTESIAN_POINT('Ctrl Pts',(-0.676681193656349,0.000319961310848927,
-5.139182021619));
#63693=CARTESIAN_POINT('Origin',(0.,0.,-12.278617978381));
#63694=CARTESIAN_POINT('',(-0.6767,2.04928741933266E-13,-5.57861797838101));
#63695=CARTESIAN_POINT('',(-0.676473652988121,-8.72929341335908E-5,-5.539182021619));
#63696=CARTESIAN_POINT('',(-0.6767,6.12423655037739E-13,-12.278617978381));
#63697=CARTESIAN_POINT('Ctrl Pts',(-0.6767,2.04928741933266E-13,-5.57861797838101));
#63698=CARTESIAN_POINT('Ctrl Pts',(-0.676700000000055,-0.181681376406979,
-5.57007194938059));
#63699=CARTESIAN_POINT('Ctrl Pts',(-0.599682817833766,-0.362452229318455,
-5.56151037025653));
#63700=CARTESIAN_POINT('Ctrl Pts',(-0.468453904192104,-0.488337823281358,
-5.55295656619429));
#63701=CARTESIAN_POINT('Ctrl Pts',(-0.327134704779409,-0.623902851313269,
-5.54374505397138));
#63702=CARTESIAN_POINT('Ctrl Pts',(-0.124836170252917,-0.693316532000011,
-5.53453354174847));
#63703=CARTESIAN_POINT('Ctrl Pts',(0.0699439537792119,-0.673075577724918,
-5.52532202952557));
#63704=CARTESIAN_POINT('Ctrl Pts',(0.264724077811341,-0.652834623449824,
-5.51611051730266));
#63705=CARTESIAN_POINT('Ctrl Pts',(0.448427764043003,-0.543308773519562,
-5.50689900507975));
#63706=CARTESIAN_POINT('Ctrl Pts',(0.558853433030084,-0.381583189344721,
-5.49768749285685));
#63707=CARTESIAN_POINT('Ctrl Pts',(0.669279102017165,-0.21985760516988,
-5.48847598063394));
#63708=CARTESIAN_POINT('Ctrl Pts',(0.704409620094189,-0.00888651037799307,
-5.47926446841103));
#63709=CARTESIAN_POINT('Ctrl Pts',(0.652349887299333,0.17989584358886,-5.47005295618813));
#63710=CARTESIAN_POINT('Ctrl Pts',(0.600290154504477,0.368678197555713,
-5.46084144396522));
#63711=CARTESIAN_POINT('Ctrl Pts',(0.461991140305252,0.531823344003806,
-5.45162993174231));
#63712=CARTESIAN_POINT('Ctrl Pts',(0.284280522987371,0.614090770367074,
-5.44241841951941));
#63713=CARTESIAN_POINT('Ctrl Pts',(0.106569905669491,0.696358196730342,
-5.4332069072965));
#63714=CARTESIAN_POINT('Ctrl Pts',(-0.107306094280518,0.696245132893723,
-5.42399539507359));
#63715=CARTESIAN_POINT('Ctrl Pts',(-0.284929632262066,0.613789861971509,
-5.41478388285069));
#63716=CARTESIAN_POINT('Ctrl Pts',(-0.462553170243613,0.531334591049295,
-5.40557237062778));
#63717=CARTESIAN_POINT('Ctrl Pts',(-0.600679616438922,0.36804331449264,
-5.39636085840487));
#63718=CARTESIAN_POINT('Ctrl Pts',(-0.652539723629315,0.179206024133614,
-5.38714934618197));
#63719=CARTESIAN_POINT('Ctrl Pts',(-0.668550039052439,0.120907945975067,
-5.38430555691498));
#63720=CARTESIAN_POINT('Ctrl Pts',(-0.67669999999998,0.0604092412225694,
-5.38145954165838));
#63721=CARTESIAN_POINT('Ctrl Pts',(-0.6767,2.19519213709729E-13,-5.37861797838101));
#63722=CARTESIAN_POINT('Ctrl Pts',(-0.675509068550524,-0.000459294334369663,
-5.539182021619));
#63723=CARTESIAN_POINT('Ctrl Pts',(-0.675920327415641,-0.101206008316284,
-5.53445130843648));
#63724=CARTESIAN_POINT('Ctrl Pts',(-0.607873754724515,-0.426945848796192,
-5.51912952959103));
#63725=CARTESIAN_POINT('Ctrl Pts',(-0.100182069364385,-0.794604796709607,
-5.49321668508265));
#63726=CARTESIAN_POINT('Ctrl Pts',(0.492200104289347,-0.56035531426314,
-5.46673902092533));
#63727=CARTESIAN_POINT('Ctrl Pts',(0.689575122107159,-0.140421506011553,
-5.44555688959948));
#63728=CARTESIAN_POINT('Ctrl Pts',(0.671714796398658,0.325523691904682,
-5.42437475827361));
#63729=CARTESIAN_POINT('Ctrl Pts',(0.308866959837698,0.679330682531593,
-5.40319262694776));
#63730=CARTESIAN_POINT('Ctrl Pts',(-0.158179798246442,0.686446681763176,
-5.3820104956219));
#63731=CARTESIAN_POINT('Ctrl Pts',(-0.467698735375229,0.528786977202589,
-5.36612389712751));
#63732=CARTESIAN_POINT('Ctrl Pts',(-0.642511679277089,0.269422734927641,
-5.35184773912654));
#63733=CARTESIAN_POINT('Ctrl Pts',(-0.677021406559707,0.078091063778343,
-5.34286711395704));
#63734=CARTESIAN_POINT('Ctrl Pts',(-0.677314241554135,-0.000241130457915198,
-5.339182021619));
#63735=CARTESIAN_POINT('Origin',(0.,0.,-12.278617978381));
#63736=CARTESIAN_POINT('',(-0.6767,1.90338270156804E-13,-5.77861797838101));
#63737=CARTESIAN_POINT('',(-0.676682641762153,7.35447311691314E-5,-5.739182021619));
#63738=CARTESIAN_POINT('',(-0.6767,6.12423655037739E-13,-12.278617978381));
#63739=CARTESIAN_POINT('Ctrl Pts',(-0.6767,1.90338270156804E-13,-5.77861797838101));
#63740=CARTESIAN_POINT('Ctrl Pts',(-0.676700000000009,-0.0324523956795152,
-5.77709146465629));
#63741=CARTESIAN_POINT('Ctrl Pts',(-0.674355800339294,-0.0649836093856385,
-5.77556123248971));
#63742=CARTESIAN_POINT('Ctrl Pts',(-0.669691645670928,-0.0971390226354201,
-5.77403285954405));
#63743=CARTESIAN_POINT('Ctrl Pts',(-0.641580759607818,-0.290939876691033,
-5.76482134732115));
#63744=CARTESIAN_POINT('Ctrl Pts',(-0.524706672654737,-0.470058284279229,
-5.75560983509824));
#63745=CARTESIAN_POINT('Ctrl Pts',(-0.358642639729406,-0.573845229106179,
-5.74639832287533));
#63746=CARTESIAN_POINT('Ctrl Pts',(-0.192578606804075,-0.67763217393313,
-5.73718681065243));
#63747=CARTESIAN_POINT('Ctrl Pts',(0.0196418984952844,-0.704191791184361,
-5.72797529842952));
#63748=CARTESIAN_POINT('Ctrl Pts',(0.206161577652617,-0.64453106511617,
-5.71876378620661));
#63749=CARTESIAN_POINT('Ctrl Pts',(0.392681256809949,-0.584870339047978,
-5.70955227398371));
#63750=CARTESIAN_POINT('Ctrl Pts',(0.550092975165776,-0.440079085643937,
-5.7003407617608));
#63751=CARTESIAN_POINT('Ctrl Pts',(0.625097543653214,-0.259183238112958,
-5.69112924953789));
#63752=CARTESIAN_POINT('Ctrl Pts',(0.700102112140652,-0.0782873905819796,
-5.68191773731498));
#63753=CARTESIAN_POINT('Ctrl Pts',(0.691329430478235,0.13540864633611,-5.67270622509208));
#63754=CARTESIAN_POINT('Ctrl Pts',(0.601749905338556,0.309547963044565,
-5.66349471286917));
#63755=CARTESIAN_POINT('Ctrl Pts',(0.512170380198877,0.483687279753019,
-5.65428320064626));
#63756=CARTESIAN_POINT('Ctrl Pts',(0.343420351008757,0.615088892324483,
-5.64507168842336));
#63757=CARTESIAN_POINT('Ctrl Pts',(0.15263812871983,0.659260564314982,-5.63586017620045));
#63758=CARTESIAN_POINT('Ctrl Pts',(-0.0381440935690977,0.703432236305481,
-5.62664866397754));
#63759=CARTESIAN_POINT('Ctrl Pts',(-0.247473510886337,0.659567088594882,
-5.61743715175464));
#63760=CARTESIAN_POINT('Ctrl Pts',(-0.404471739415305,0.542517743501867,
-5.60822563953173));
#63761=CARTESIAN_POINT('Ctrl Pts',(-0.561469967944274,0.425468398408852,
-5.59901412730882));
#63762=CARTESIAN_POINT('Ctrl Pts',(-0.663269138148019,0.237372983568734,
-5.58980261508592));
#63763=CARTESIAN_POINT('Ctrl Pts',(-0.675400321815768,0.0419201060489659,
-5.58059110286301));
#63764=CARTESIAN_POINT('Ctrl Pts',(-0.676266496478922,0.0279646392961009,
-5.57993339470234));
#63765=CARTESIAN_POINT('Ctrl Pts',(-0.676699999999996,0.0139696120037695,
-5.57927508871157));
#63766=CARTESIAN_POINT('Ctrl Pts',(-0.6767,2.04928741933266E-13,-5.57861797838101));
#63767=CARTESIAN_POINT('Ctrl Pts',(-0.6767,2.01980204130163E-13,-5.739182021619));
#63768=CARTESIAN_POINT('Ctrl Pts',(-0.676700000000043,-0.144550082451763,
-5.73238259494645));
#63769=CARTESIAN_POINT('Ctrl Pts',(-0.628766694107548,-0.288982634149047,
-5.72556986467741));
#63770=CARTESIAN_POINT('Ctrl Pts',(-0.542188500137206,-0.404912978699086,
-5.71876378620661));
#63771=CARTESIAN_POINT('Ctrl Pts',(-0.425011465605937,-0.561815928086265,
-5.7095522739837));
#63772=CARTESIAN_POINT('Ctrl Pts',(-0.236833292830468,-0.663462036860449,
-5.7003407617608));
#63773=CARTESIAN_POINT('Ctrl Pts',(-0.0413706104950007,-0.67543420300372,
-5.69112924953789));
#63774=CARTESIAN_POINT('Ctrl Pts',(0.154092071840467,-0.687406369146992,
-5.68191773731498));
#63775=CARTESIAN_POINT('Ctrl Pts',(0.353268768211662,-0.609485898404675,
-5.67270622509208));
#63776=CARTESIAN_POINT('Ctrl Pts',(0.488718779104662,-0.468056454875316,
-5.66349471286917));
#63777=CARTESIAN_POINT('Ctrl Pts',(0.624168789997662,-0.326627011345958,
-5.65428320064626));
#63778=CARTESIAN_POINT('Ctrl Pts',(0.693417864819581,-0.124272071267007,
-5.64507168842336));
#63779=CARTESIAN_POINT('Ctrl Pts',(0.673018451061671,0.0704915209833714,
-5.63586017620045));
#63780=CARTESIAN_POINT('Ctrl Pts',(0.652619037303762,0.265255113233749,
-5.62664866397754));
#63781=CARTESIAN_POINT('Ctrl Pts',(0.542943768834802,0.448869632333708,
-5.61743715175464));
#63782=CARTESIAN_POINT('Ctrl Pts',(0.381128399785082,0.559163690592713,
-5.60822563953173));
#63783=CARTESIAN_POINT('Ctrl Pts',(0.219313030735361,0.669457748851717,
-5.59901412730882));
#63784=CARTESIAN_POINT('Ctrl Pts',(0.0083134248229402,0.704416616723123,
-5.58980261508592));
#63785=CARTESIAN_POINT('Ctrl Pts',(-0.180426512720538,0.652203314548083,
-5.58059110286301));
#63786=CARTESIAN_POINT('Ctrl Pts',(-0.369166450264015,0.599990012373043,
-5.5713795906401));
#63787=CARTESIAN_POINT('Ctrl Pts',(-0.53219902756101,0.461558314854205,
-5.56216807841719));
#63788=CARTESIAN_POINT('Ctrl Pts',(-0.614321847660544,0.283780826496322,
-5.55295656619429));
#63789=CARTESIAN_POINT('Ctrl Pts',(-0.655256293555913,0.195166931238217,
-5.54836505133586));
#63790=CARTESIAN_POINT('Ctrl Pts',(-0.676699999999966,0.0975831743075417,
-5.5437721929072));
#63791=CARTESIAN_POINT('Ctrl Pts',(-0.6767,2.3580364667818E-13,-5.539182021619));
#63792=CARTESIAN_POINT('Origin',(0.,0.,-12.278617978381));
#63793=CARTESIAN_POINT('',(-0.675992408981733,-0.00051856590770552,-5.97861797838101));
#63794=CARTESIAN_POINT('',(-0.677862131410808,-0.000317623256960498,-5.939182021619));
#63795=CARTESIAN_POINT('',(-0.6767,6.12423655037739E-13,-12.278617978381));
#63796=CARTESIAN_POINT('Ctrl Pts',(-0.675992408981733,-0.000518565907705555,
-5.97861797838101));
#63797=CARTESIAN_POINT('Ctrl Pts',(-0.676480548855683,-0.0808249889540484,
-5.97484937328625));
#63798=CARTESIAN_POINT('Ctrl Pts',(-0.625946858428093,-0.386173097447615,
-5.96048970252857));
#63799=CARTESIAN_POINT('Ctrl Pts',(-0.172598743972036,-0.781008560151051,
-5.93553896610797));
#63800=CARTESIAN_POINT('Ctrl Pts',(0.562958377491915,-0.568642748947718,
-5.90376576911917));
#63801=CARTESIAN_POINT('Ctrl Pts',(0.78296431633078,0.166020846752831,-5.87199257213039));
#63802=CARTESIAN_POINT('Ctrl Pts',(0.367652295433943,0.649277541756489,
-5.84551490797305));
#63803=CARTESIAN_POINT('Ctrl Pts',(-0.094108426135513,0.697311105773554,
-5.82433277664721));
#63804=CARTESIAN_POINT('Ctrl Pts',(-0.51485447745632,0.532696085594891,
-5.803798977727));
#63805=CARTESIAN_POINT('Ctrl Pts',(-0.675957546053224,0.210905853308733,
-5.78856071163828));
#63806=CARTESIAN_POINT('Ctrl Pts',(-0.677343470085779,8.23098365132415E-5,
-5.77861797838101));
#63807=CARTESIAN_POINT('Ctrl Pts',(-0.677862131410808,-0.000317623256960531,
-5.939182021619));
#63808=CARTESIAN_POINT('Ctrl Pts',(-0.677882831941353,-0.00835939249928384,
-5.93880182872123));
#63809=CARTESIAN_POINT('Ctrl Pts',(-0.673999656496432,-0.240380536296751,
-5.92783057016052));
#63810=CARTESIAN_POINT('Ctrl Pts',(-0.473532610433715,-0.576625011097358,
-5.91156377876836));
#63811=CARTESIAN_POINT('Ctrl Pts',(-0.0268458389766041,-0.703120526676957,
-5.8903816474425));
#63812=CARTESIAN_POINT('Ctrl Pts',(0.429873304441071,-0.610241380137162,
-5.86919951611663));
#63813=CARTESIAN_POINT('Ctrl Pts',(0.72041369487452,-0.194790217664389,
-5.84801738479079));
#63814=CARTESIAN_POINT('Ctrl Pts',(0.651769364779252,0.267190941228426,
-5.82683525346492));
#63815=CARTESIAN_POINT('Ctrl Pts',(0.446117917906169,0.547134871850125,
-5.81094865497054));
#63816=CARTESIAN_POINT('Ctrl Pts',(0.129797396400296,0.692369309990026,
-5.79506205647613));
#63817=CARTESIAN_POINT('Ctrl Pts',(-0.335295695534132,0.666226148989499,
-5.77387992515028));
#63818=CARTESIAN_POINT('Ctrl Pts',(-0.643488391291915,0.342319004679031,
-5.75525324686457));
#63819=CARTESIAN_POINT('Ctrl Pts',(-0.67701347904639,0.0592534314261598,
-5.74192210141032));
#63820=CARTESIAN_POINT('Ctrl Pts',(-0.676484660513756,0.000912367068930366,
-5.739182021619));
#63821=CARTESIAN_POINT('Origin',(0.,0.,-12.278617978381));
#63822=CARTESIAN_POINT('',(-0.676704782873988,0.000128481712317595,-6.17861797838101));
#63823=CARTESIAN_POINT('',(-0.676556184750891,-0.000492135516488926,-6.139182021619));
#63824=CARTESIAN_POINT('',(-0.6767,6.12423655037739E-13,-12.278617978381));
#63825=CARTESIAN_POINT('Ctrl Pts',(-0.676704782873988,0.000128481712317646,
-6.17861797838101));
#63826=CARTESIAN_POINT('Ctrl Pts',(-0.676580798701789,-0.0338241820643936,
-6.17702463342863));
#63827=CARTESIAN_POINT('Ctrl Pts',(-0.665162410638196,-0.180638294760152,
-6.17013575564478));
#63828=CARTESIAN_POINT('Ctrl Pts',(-0.562221864267348,-0.426947701728367,
-6.15795134502947));
#63829=CARTESIAN_POINT('Ctrl Pts',(-0.289550464019102,-0.642148606418798,
-6.14206474653509));
#63830=CARTESIAN_POINT('Ctrl Pts',(0.169783162631269,-0.726713697646756,
-6.1208826152092));
#63831=CARTESIAN_POINT('Ctrl Pts',(0.595024636138863,-0.450700878954778,
-6.09970048388339));
#63832=CARTESIAN_POINT('Ctrl Pts',(0.70362826836473,0.00253654546368757,
-6.07851835255749));
#63833=CARTESIAN_POINT('Ctrl Pts',(0.592641591588357,0.453327123043412,
-6.05733622123166));
#63834=CARTESIAN_POINT('Ctrl Pts',(0.0569329064749938,0.798344967018745,
-6.03085855707431));
#63835=CARTESIAN_POINT('Ctrl Pts',(-0.557831024569953,0.517353749803968,
-6.0028539651803));
#63836=CARTESIAN_POINT('Ctrl Pts',(-0.675108709321502,0.144863449673475,
-5.98544043894919));
#63837=CARTESIAN_POINT('Ctrl Pts',(-0.675992408981733,-0.000518565907705555,
-5.97861797838101));
#63838=CARTESIAN_POINT('Ctrl Pts',(-0.676556184750892,-0.000492135516488929,
-6.139182021619));
#63839=CARTESIAN_POINT('Ctrl Pts',(-0.676915433003454,-0.0750118267480244,
-6.13568155603213));
#63840=CARTESIAN_POINT('Ctrl Pts',(-0.629822248076123,-0.374271290200019,
-6.12159002478234));
#63841=CARTESIAN_POINT('Ctrl Pts',(-0.192973643036106,-0.776760719460778,
-6.09690742786962));
#63842=CARTESIAN_POINT('Ctrl Pts',(0.548852666849259,-0.58226923395591,
-6.06513423088083));
#63843=CARTESIAN_POINT('Ctrl Pts',(0.786505655010167,0.145511346935457,
-6.03336103389204));
#63844=CARTESIAN_POINT('Ctrl Pts',(0.303954112232331,0.739849035349103,
-6.00158783690326));
#63845=CARTESIAN_POINT('Ctrl Pts',(-0.448015488347003,0.657740779645327,
-5.97019483281224));
#63846=CARTESIAN_POINT('Ctrl Pts',(-0.67730617551369,0.215660852461966,
-5.94939289438415));
#63847=CARTESIAN_POINT('Ctrl Pts',(-0.677862131410808,-0.000317623256960531,
-5.939182021619));
#63848=CARTESIAN_POINT('Origin',(0.,0.,-12.278617978381));
#63849=CARTESIAN_POINT('',(-0.6767,1.4656678648528E-13,-6.37861797838101));
#63850=CARTESIAN_POINT('',(-0.675457068551241,0.00029468390945811,-6.339182021619));
#63851=CARTESIAN_POINT('',(-0.6767,6.12423655037739E-13,-12.278617978381));
#63852=CARTESIAN_POINT('Ctrl Pts',(-0.676875242892834,9.14395672268094E-5,
-6.37861797838101));
#63853=CARTESIAN_POINT('Ctrl Pts',(-0.67674179299303,-0.0997811966725849,
-6.37390436073954));
#63854=CARTESIAN_POINT('Ctrl Pts',(-0.628299285756436,-0.311940683515031,
-6.3638952102666));
#63855=CARTESIAN_POINT('Ctrl Pts',(-0.340972135963656,-0.663797545482861,
-6.34329499413074));
#63856=CARTESIAN_POINT('Ctrl Pts',(0.161643869936548,-0.728723180265365,
-6.32211286280486));
#63857=CARTESIAN_POINT('Ctrl Pts',(0.538076797651925,-0.453547551601197,
-6.30093073147902));
#63858=CARTESIAN_POINT('Ctrl Pts',(0.744851349578635,-0.038160346185337,
-6.27974860015315));
#63859=CARTESIAN_POINT('Ctrl Pts',(0.560874095982173,0.57170878506611,-6.25327093599583));
#63860=CARTESIAN_POINT('Ctrl Pts',(-0.178950953192254,0.780037574273926,
-6.22149773900705));
#63861=CARTESIAN_POINT('Ctrl Pts',(-0.625642030755787,0.383504116506336,
-6.1966134198021));
#63862=CARTESIAN_POINT('Ctrl Pts',(-0.676992864057429,0.079018580249279,
-6.18232016626009));
#63863=CARTESIAN_POINT('Ctrl Pts',(-0.676704782873988,0.000128481712317646,
-6.17861797838101));
#63864=CARTESIAN_POINT('Ctrl Pts',(-0.675457068551241,0.000294683909458103,
-6.339182021619));
#63865=CARTESIAN_POINT('Ctrl Pts',(-0.674863684696936,-0.140825266627321,
-6.33256128334304));
#63866=CARTESIAN_POINT('Ctrl Pts',(-0.563978321160066,-0.508573136181875,
-6.31534947940416));
#63867=CARTESIAN_POINT('Ctrl Pts',(0.042556028366106,-0.799168971730803,
-6.28754660980234));
#63868=CARTESIAN_POINT('Ctrl Pts',(0.58315304606446,-0.46498710724797,-6.26106894564502));
#63869=CARTESIAN_POINT('Ctrl Pts',(0.704267131783399,-0.0151800071787377,
-6.23988681431916));
#63870=CARTESIAN_POINT('Ctrl Pts',(0.627100262560229,0.324226811612303,
-6.22400021582477));
#63871=CARTESIAN_POINT('Ctrl Pts',(0.395365052280528,0.582992949678207,
-6.20811361733038));
#63872=CARTESIAN_POINT('Ctrl Pts',(-0.0426668885056882,0.745062854587275,
-6.18693148600451));
#63873=CARTESIAN_POINT('Ctrl Pts',(-0.508936057342763,0.546049163939659,
-6.16574935467866));
#63874=CARTESIAN_POINT('Ctrl Pts',(-0.663119369583067,0.188858374715681,
-6.14806768893966));
#63875=CARTESIAN_POINT('Ctrl Pts',(-0.676371959322915,0.0377221686919021,
-6.1409770888636));
#63876=CARTESIAN_POINT('Ctrl Pts',(-0.676556184750892,-0.000492135516488929,
-6.139182021619));
#63877=CARTESIAN_POINT('Origin',(0.,0.,-12.278617978381));
#63878=CARTESIAN_POINT('',(-0.6767,1.31976383050954E-13,-6.57861797838101));
#63879=CARTESIAN_POINT('',(-0.677816872487775,0.000601865446929958,-6.539182021619));
#63880=CARTESIAN_POINT('',(-0.6767,6.12423655037739E-13,-12.278617978381));
#63881=CARTESIAN_POINT('Ctrl Pts',(-0.6767,1.31976383050954E-13,-6.57861797838101));
#63882=CARTESIAN_POINT('Ctrl Pts',(-0.676700000000005,-0.0225339661634695,
-6.57755801322587));
#63883=CARTESIAN_POINT('Ctrl Pts',(-0.675570903631601,-0.0451197667652925,
-6.57649560808497));
#63884=CARTESIAN_POINT('Ctrl Pts',(-0.673318349535998,-0.0675669310988747,
-6.57543442293695));
#63885=CARTESIAN_POINT('Ctrl Pts',(-0.653765277554997,-0.262417310426306,
-6.56622291071404));
#63886=CARTESIAN_POINT('Ctrl Pts',(-0.544888756309662,-0.446506580237345,
-6.55701139849113));
#63887=CARTESIAN_POINT('Ctrl Pts',(-0.383554086245299,-0.557502603513682,
-6.54779988626823));
#63888=CARTESIAN_POINT('Ctrl Pts',(-0.222219416180937,-0.668498626790019,
-6.53858837404532));
#63889=CARTESIAN_POINT('Ctrl Pts',(-0.0113736801396104,-0.704373851266513,
-6.52937686182241));
#63890=CARTESIAN_POINT('Ctrl Pts',(0.177591316576043,-0.652981021375651,
-6.52016534959951));
#63891=CARTESIAN_POINT('Ctrl Pts',(0.366556313291696,-0.601588191484788,
-6.5109538373766));
#63892=CARTESIAN_POINT('Ctrl Pts',(0.530188767672756,-0.463866094451386,
-6.50174232515369));
#63893=CARTESIAN_POINT('Ctrl Pts',(0.613083165983457,-0.286447065943606,
-6.49253081293079));
#63894=CARTESIAN_POINT('Ctrl Pts',(0.695977564294159,-0.109028037435825,
-6.48331930070788));
#63895=CARTESIAN_POINT('Ctrl Pts',(0.696619683591181,0.104847028480835,
-6.47410778848497));
#63896=CARTESIAN_POINT('Ctrl Pts',(0.614792103988806,0.282760603466992,
-6.46489627626207));
#63897=CARTESIAN_POINT('Ctrl Pts',(0.53296452438643,0.460674178453149,-6.45568476403916));
#63898=CARTESIAN_POINT('Ctrl Pts',(0.370161981366855,0.59937633461666,-6.44647325181625));
#63899=CARTESIAN_POINT('Ctrl Pts',(0.181508982886692,0.651902890875197,
-6.43726173959334));
#63900=CARTESIAN_POINT('Ctrl Pts',(-0.00714401559347194,0.704429447133734,
-6.42805022737044));
#63901=CARTESIAN_POINT('Ctrl Pts',(-0.218201365763082,0.669820906606433,
-6.41883871514753));
#63902=CARTESIAN_POINT('Ctrl Pts',(-0.380199610338631,0.559795629045416,
-6.40962720292462));
#63903=CARTESIAN_POINT('Ctrl Pts',(-0.542197854914179,0.4497703514844,-6.40041569070172));
#63904=CARTESIAN_POINT('Ctrl Pts',(-0.652177789610297,0.266338156648583,
-6.39120417847881));
#63905=CARTESIAN_POINT('Ctrl Pts',(-0.672900501122695,0.0716086977177066,
-6.3819926662559));
#63906=CARTESIAN_POINT('Ctrl Pts',(-0.675431127350092,0.047828630339819,
-6.3808677702976));
#63907=CARTESIAN_POINT('Ctrl Pts',(-0.676699999999995,0.0238863472897277,
-6.37974155758702));
#63908=CARTESIAN_POINT('Ctrl Pts',(-0.6767,1.46566854827417E-13,-6.37861797838101));
#63909=CARTESIAN_POINT('Ctrl Pts',(-0.677816872487775,0.000601865446929938,
-6.539182021619));
#63910=CARTESIAN_POINT('Ctrl Pts',(-0.67655614108913,-0.205703460295888,
-6.52944101065395));
#63911=CARTESIAN_POINT('Ctrl Pts',(-0.464731990145984,-0.639726014582718,
-6.50910893402597));
#63912=CARTESIAN_POINT('Ctrl Pts',(0.143458633831261,-0.731914130435804,
-6.48348132456653));
#63913=CARTESIAN_POINT('Ctrl Pts',(0.526965677843967,-0.467479525104637,
-6.46229919324067));
#63914=CARTESIAN_POINT('Ctrl Pts',(0.687844780422188,-0.158831240600472,
-6.44641259474628));
#63915=CARTESIAN_POINT('Ctrl Pts',(0.678772152266887,0.188409603808886,
-6.43052599625188));
#63916=CARTESIAN_POINT('Ctrl Pts',(0.449737145934374,0.595504557883058,
-6.40934386492603));
#63917=CARTESIAN_POINT('Ctrl Pts',(-0.0343035843211689,0.745647019873919,
-6.38816173360018));
#63918=CARTESIAN_POINT('Ctrl Pts',(-0.452343460848582,0.539089431506795,
-6.36697960227431));
#63919=CARTESIAN_POINT('Ctrl Pts',(-0.641343804359365,0.282137405713559,
-6.35241820922441));
#63920=CARTESIAN_POINT('Ctrl Pts',(-0.675812909255033,0.0849215610206185,
-6.34315234900597));
#63921=CARTESIAN_POINT('Ctrl Pts',(-0.675457068551241,0.000294683909458103,
-6.339182021619));
#63922=CARTESIAN_POINT('Origin',(0.,0.,-12.278617978381));
#63923=CARTESIAN_POINT('',(-0.676558247700131,-7.87320039269999E-6,-6.77861797838101));
#63924=CARTESIAN_POINT('',(-0.676709423551057,-8.49736032138343E-5,-6.739182021619));
#63925=CARTESIAN_POINT('',(-0.6767,6.12423655037739E-13,-12.278617978381));
#63926=CARTESIAN_POINT('Ctrl Pts',(-0.6767,1.17385911274492E-13,-6.77861797838101));
#63927=CARTESIAN_POINT('Ctrl Pts',(-0.676700000000012,-0.0689923121809674,
-6.77537267986794));
#63928=CARTESIAN_POINT('Ctrl Pts',(-0.666054446306332,-0.138058240211869,
-6.77212344587233));
#63929=CARTESIAN_POINT('Ctrl Pts',(-0.645254990554443,-0.203884494664468,
-6.76887617961799));
#63930=CARTESIAN_POINT('Ctrl Pts',(-0.586253225413585,-0.390613669295004,
-6.75966466739508));
#63931=CARTESIAN_POINT('Ctrl Pts',(-0.442018685279904,-0.548535655004635,
-6.75045315517218));
#63932=CARTESIAN_POINT('Ctrl Pts',(-0.261388801730013,-0.624178487557964,
-6.74124164294927));
#63933=CARTESIAN_POINT('Ctrl Pts',(-0.0807589181801233,-0.699821320111294,
-6.73203013072636));
#63934=CARTESIAN_POINT('Ctrl Pts',(0.132966762381217,-0.691803240126696,
-6.72281861850346));
#63935=CARTESIAN_POINT('Ctrl Pts',(0.30742129309852,-0.602839148156151,
-6.71360710628055));
#63936=CARTESIAN_POINT('Ctrl Pts',(0.481875823815823,-0.513875056185606,
-6.70439559405764));
#63937=CARTESIAN_POINT('Ctrl Pts',(0.613872462781772,-0.345590049605281,
-6.69518408183474));
#63938=CARTESIAN_POINT('Ctrl Pts',(0.658717499198191,-0.154964983948248,
-6.68597256961183));
#63939=CARTESIAN_POINT('Ctrl Pts',(0.703562535614611,0.0356600817087843,
-6.67676105738892));
#63940=CARTESIAN_POINT('Ctrl Pts',(0.660436790086757,0.245143079135101,
-6.66754954516601));
#63941=CARTESIAN_POINT('Ctrl Pts',(0.543942525321295,0.402553622697762,
-6.65833803294311));
#63942=CARTESIAN_POINT('Ctrl Pts',(0.427448260555833,0.559964166260423,
-6.6491265207202));
#63943=CARTESIAN_POINT('Ctrl Pts',(0.239713464596202,0.662426854708672,
-6.63991500849729));
#63944=CARTESIAN_POINT('Ctrl Pts',(0.0443046399162912,0.675248094319331,
-6.63070349627439));
#63945=CARTESIAN_POINT('Ctrl Pts',(-0.151104184763619,0.68806933392999,
-6.62149198405148));
#63946=CARTESIAN_POINT('Ctrl Pts',(-0.350617526451464,0.611014920515853,
-6.61228047182857));
#63947=CARTESIAN_POINT('Ctrl Pts',(-0.486680698424695,0.470175273468152,
-6.60306895960567));
#63948=CARTESIAN_POINT('Ctrl Pts',(-0.607069113224888,0.345560643343055,
-6.59491863253078));
#63949=CARTESIAN_POINT('Ctrl Pts',(-0.676699999999966,0.173069887823577,
-6.58675893542178));
#63950=CARTESIAN_POINT('Ctrl Pts',(-0.6767,1.31976383050954E-13,-6.57861797838101));
#63951=CARTESIAN_POINT('Ctrl Pts',(-0.676804323507533,-0.000940701036842954,
-6.73918202161899));
#63952=CARTESIAN_POINT('Ctrl Pts',(-0.6772597637176,-0.0492104853983123,
-6.73691180362778));
#63953=CARTESIAN_POINT('Ctrl Pts',(-0.650606445369866,-0.322003920915775,
-6.72405051997364));
#63954=CARTESIAN_POINT('Ctrl Pts',(-0.36446354353643,-0.650726522050533,
-6.70589370348805));
#63955=CARTESIAN_POINT('Ctrl Pts',(0.0990244122389695,-0.697441110221215,
-6.68471157216218));
#63956=CARTESIAN_POINT('Ctrl Pts',(0.421449152886381,-0.566337695957096,
-6.6688249736678));
#63957=CARTESIAN_POINT('Ctrl Pts',(0.639321376606824,-0.295800731727484,
-6.6529383751734));
#63958=CARTESIAN_POINT('Ctrl Pts',(0.72828669883045,0.162749683301894,-6.63175624384754));
#63959=CARTESIAN_POINT('Ctrl Pts',(0.456550800284682,0.590531801388853,
-6.61057411252168));
#63960=CARTESIAN_POINT('Ctrl Pts',(0.00420849966872835,0.703714670097329,
-6.58939198119583));
#63961=CARTESIAN_POINT('Ctrl Pts',(-0.447311932305929,0.59680068373128,
-6.56820984986996));
#63962=CARTESIAN_POINT('Ctrl Pts',(-0.66913515988933,0.260749856922413,
-6.55147319667769));
#63963=CARTESIAN_POINT('Ctrl Pts',(-0.67792689090907,0.0186052135567966,
-6.54003207631688));
#63964=CARTESIAN_POINT('Ctrl Pts',(-0.677816872487775,0.000601865446929938,
-6.539182021619));
#63965=CARTESIAN_POINT('Origin',(0.,0.,-12.278617978381));
#63966=CARTESIAN_POINT('',(-0.677117923044813,0.000572801869896454,-6.97861797838101));
#63967=CARTESIAN_POINT('',(-0.676424852156372,7.29842916120558E-5,-6.939182021619));
#63968=CARTESIAN_POINT('',(-0.6767,6.12423655037739E-13,-12.278617978381));
#63969=CARTESIAN_POINT('Ctrl Pts',(-0.677117923044813,0.000572801869896465,
-6.978617978381));
#63970=CARTESIAN_POINT('Ctrl Pts',(-0.676704078716193,-0.0735018107475405,
-6.97513460833519));
#63971=CARTESIAN_POINT('Ctrl Pts',(-0.64466818210056,-0.260791847049063,
-6.9663557054579));
#63972=CARTESIAN_POINT('Ctrl Pts',(-0.416626705641162,-0.618612325309093,
-6.9469857369177));
#63973=CARTESIAN_POINT('Ctrl Pts',(0.200815735222948,-0.77531043778035,
-6.92050807276037));
#63974=CARTESIAN_POINT('Ctrl Pts',(0.760672052637908,-0.248711886132582,
-6.88873487577159));
#63975=CARTESIAN_POINT('Ctrl Pts',(0.644101608620266,0.376047601873901,
-6.86225721161426));
#63976=CARTESIAN_POINT('Ctrl Pts',(0.268310163838186,0.651336773415186,
-6.8410750802884));
#63977=CARTESIAN_POINT('Ctrl Pts',(-0.07606725508181,0.701834415681397,
-6.825188481794));
#63978=CARTESIAN_POINT('Ctrl Pts',(-0.401035133744832,0.579137908513486,
-6.80930188329962));
#63979=CARTESIAN_POINT('Ctrl Pts',(-0.627635862151523,0.322555973188607,
-6.79377838216195));
#63980=CARTESIAN_POINT('Ctrl Pts',(-0.675440530384168,0.104886329948958,
-6.78355041385574));
#63981=CARTESIAN_POINT('Ctrl Pts',(-0.675270388616731,-7.94034175511452E-5,
-6.778617978381));
#63982=CARTESIAN_POINT('Ctrl Pts',(-0.6767,1.14437373471389E-13,-6.939182021619));
#63983=CARTESIAN_POINT('Ctrl Pts',(-0.676700000000005,-0.0318401568288711,
-6.93768430672372));
#63984=CARTESIAN_POINT('Ctrl Pts',(-0.674443556279103,-0.063757730454072,
-6.93618294029321));
#63985=CARTESIAN_POINT('Ctrl Pts',(-0.669953136301276,-0.095318860463623,
-6.93468339963031));
#63986=CARTESIAN_POINT('Ctrl Pts',(-0.642368983676898,-0.289195386819788,
-6.92547188740741));
#63987=CARTESIAN_POINT('Ctrl Pts',(-0.525982060165414,-0.468630723845636,
-6.9162603751845));
#63988=CARTESIAN_POINT('Ctrl Pts',(-0.36020066843924,-0.572868543782886,
-6.90704886296159));
#63989=CARTESIAN_POINT('Ctrl Pts',(-0.194419276713066,-0.677106363720137,
-6.89783735073869));
#63990=CARTESIAN_POINT('Ctrl Pts',(0.0177282726055708,-0.704242565667796,
-6.88862583851578));
#63991=CARTESIAN_POINT('Ctrl Pts',(0.204409383701599,-0.645088903837861,
-6.87941432629287));
#63992=CARTESIAN_POINT('Ctrl Pts',(0.391090494797627,-0.585935242007925,
-6.87020281406997));
#63993=CARTESIAN_POINT('Ctrl Pts',(0.548895084151931,-0.441572269896767,
-6.86099130184706));
#63994=CARTESIAN_POINT('Ctrl Pts',(0.624390937622713,-0.260880905806902,
-6.85177978962415));
#63995=CARTESIAN_POINT('Ctrl Pts',(0.699886791093495,-0.0801895417170372,
-6.84256827740125));
#63996=CARTESIAN_POINT('Ctrl Pts',(0.691694834150018,0.13352954488845,-6.83335676517834));
#63997=CARTESIAN_POINT('Ctrl Pts',(0.602588841619969,0.307911639849981,
-6.82414525295543));
#63998=CARTESIAN_POINT('Ctrl Pts',(0.513482849089919,0.482293734811513,
-6.81493374073253));
#63999=CARTESIAN_POINT('Ctrl Pts',(0.345090510431523,0.614153419397832,
-6.80572222850962));
#64000=CARTESIAN_POINT('Ctrl Pts',(0.15442902353395,0.658843355199361,-6.79651071628671));
#64001=CARTESIAN_POINT('Ctrl Pts',(-0.0362324633636222,0.703533291000889,
-6.7872992040638));
#64002=CARTESIAN_POINT('Ctrl Pts',(-0.245680305890116,0.660237131828919,
-6.7780876918409));
#64003=CARTESIAN_POINT('Ctrl Pts',(-0.402996021768146,0.543614841996655,
-6.76887617961799));
#64004=CARTESIAN_POINT('Ctrl Pts',(-0.560311737646177,0.42699255216439,
-6.75966466739508));
#64005=CARTESIAN_POINT('Ctrl Pts',(-0.662621657831973,0.239174458335219,
-6.75045315517218));
#64006=CARTESIAN_POINT('Ctrl Pts',(-0.675283915529609,0.0437552674200567,
-6.74124164294927));
#64007=CARTESIAN_POINT('Ctrl Pts',(-0.676227642444813,0.0291905385527463,
-6.74055510250584));
#64008=CARTESIAN_POINT('Ctrl Pts',(-0.676699999999997,0.0145816535338437,
-6.73986792149733));
#64009=CARTESIAN_POINT('Ctrl Pts',(-0.6767,1.29027845247851E-13,-6.739182021619));
#64010=CARTESIAN_POINT('Origin',(0.,0.,-12.278617978381));
#64011=CARTESIAN_POINT('',(-0.677341240022379,-0.00028442510368357,-7.17861797838101));
#64012=CARTESIAN_POINT('',(-0.677180734722105,0.000258105871726116,-7.13918202161899));
#64013=CARTESIAN_POINT('',(-0.6767,6.12423655037739E-13,-12.278617978381));
#64014=CARTESIAN_POINT('Ctrl Pts',(-0.677341240022379,-0.000284425103683573,
-7.17861797838101));
#64015=CARTESIAN_POINT('Ctrl Pts',(-0.677448645608267,-0.0280058869623878,
-7.17730986847756));
#64016=CARTESIAN_POINT('Ctrl Pts',(-0.662413805830168,-0.279976094954333,
-7.16541069291119));
#64017=CARTESIAN_POINT('Ctrl Pts',(-0.348839181256874,-0.720933048253655,
-7.14292045168188));
#64018=CARTESIAN_POINT('Ctrl Pts',(0.418773010672415,-0.681988811858619,
-7.1111472546931));
#64019=CARTESIAN_POINT('Ctrl Pts',(0.7343636570957,-0.130340708297302,-7.08466959053577));
#64020=CARTESIAN_POINT('Ctrl Pts',(0.626147981225155,0.322751672388126,
-7.06348745920991));
#64021=CARTESIAN_POINT('Ctrl Pts',(0.396356446240715,0.58417406811166,-7.04760086071553));
#64022=CARTESIAN_POINT('Ctrl Pts',(0.069241032314998,0.70102466077804,-7.03171426222112));
#64023=CARTESIAN_POINT('Ctrl Pts',(-0.393074702260597,0.634335284449263,
-7.01053213089527));
#64024=CARTESIAN_POINT('Ctrl Pts',(-0.656026752865113,0.302421633265633,
-6.99283336961523));
#64025=CARTESIAN_POINT('Ctrl Pts',(-0.677333218371325,0.0391088329492429,
-6.98043014116665));
#64026=CARTESIAN_POINT('Ctrl Pts',(-0.677117923044813,0.000572801869896465,
-6.978617978381));
#64027=CARTESIAN_POINT('Ctrl Pts',(-0.677180734722105,0.000258105871726134,
-7.13918202161899));
#64028=CARTESIAN_POINT('Ctrl Pts',(-0.676883705358868,-0.0681365544791201,
-7.13596679108107));
#64029=CARTESIAN_POINT('Ctrl Pts',(-0.648438885871331,-0.249497900513073,
-7.12745602771168));
#64030=CARTESIAN_POINT('Ctrl Pts',(-0.49064907573534,-0.507564044048387,
-7.11364973151081));
#64031=CARTESIAN_POINT('Ctrl Pts',(-0.188413006671554,-0.678771268169181,
-7.09776313301643));
#64032=CARTESIAN_POINT('Ctrl Pts',(0.278490899227765,-0.692337918723144,
-7.07658100169056));
#64033=CARTESIAN_POINT('Ctrl Pts',(0.656645685556425,-0.354940679903258,
-7.05539887036471));
#64034=CARTESIAN_POINT('Ctrl Pts',(0.695115409901483,0.109757071136956,
-7.03421673903885));
#64035=CARTESIAN_POINT('Ctrl Pts',(0.516523923338716,0.538016781798218,
-7.01303460771299));
#64036=CARTESIAN_POINT('Ctrl Pts',(-0.0649075310191635,0.798260763698985,
-6.98655694355567));
#64037=CARTESIAN_POINT('Ctrl Pts',(-0.597869132640885,0.447184752523441,
-6.96017423724718));
#64038=CARTESIAN_POINT('Ctrl Pts',(-0.675617621543642,0.111143512104154,
-6.94438259660162));
#64039=CARTESIAN_POINT('Ctrl Pts',(-0.675400146481493,0.000344792410071813,
-6.939182021619));
#64040=CARTESIAN_POINT('Origin',(0.,0.,-12.278617978381));
#64041=CARTESIAN_POINT('',(-0.675588369597491,-0.000390811426926173,-7.37861797838101));
#64042=CARTESIAN_POINT('',(-0.676774544010776,-0.000254207991752908,-7.339182021619));
#64043=CARTESIAN_POINT('',(-0.6767,6.12423655037739E-13,-12.278617978381));
#64044=CARTESIAN_POINT('Ctrl Pts',(-0.675588369597491,-0.000390811426926201,
-7.37861797838101));
#64045=CARTESIAN_POINT('Ctrl Pts',(-0.676146181321002,-0.0947607935846297,
-7.37418959578847));
#64046=CARTESIAN_POINT('Ctrl Pts',(-0.614211218569264,-0.414290428991899,
-7.35917014753301));
#64047=CARTESIAN_POINT('Ctrl Pts',(-0.122302166900868,-0.790899332367473,
-7.3335596336146));
#64048=CARTESIAN_POINT('Ctrl Pts',(0.475348861974375,-0.574736583594672,
-7.30708196945728));
#64049=CARTESIAN_POINT('Ctrl Pts',(0.686178318089926,-0.159340052105395,
-7.28589983813143));
#64050=CARTESIAN_POINT('Ctrl Pts',(0.680265741730897,0.18866980404402,-7.27001323963702));
#64051=CARTESIAN_POINT('Ctrl Pts',(0.50658489163482,0.489491208442347,-7.25412664114265));
#64052=CARTESIAN_POINT('Ctrl Pts',(0.111040555138311,0.737942389193872,
-7.23294450981677));
#64053=CARTESIAN_POINT('Ctrl Pts',(-0.385978182755204,0.638895363144113,
-7.21176237849093));
#64054=CARTESIAN_POINT('Ctrl Pts',(-0.638174968181164,0.281410096762473,
-7.1918883570685));
#64055=CARTESIAN_POINT('Ctrl Pts',(-0.677013842840659,0.0842170317865397,
-7.18260540130902));
#64056=CARTESIAN_POINT('Ctrl Pts',(-0.677341240022379,-0.000284425103683573,
-7.17861797838101));
#64057=CARTESIAN_POINT('Ctrl Pts',(-0.676774544010776,-0.00025420799175294,
-7.339182021619));
#64058=CARTESIAN_POINT('Ctrl Pts',(-0.676830719503838,-0.0223091699601035,
-7.33814205122344));
#64059=CARTESIAN_POINT('Ctrl Pts',(-0.670522348189875,-0.156602863542262,
-7.33180654799642));
#64060=CARTESIAN_POINT('Ctrl Pts',(-0.583010888431519,-0.39538361061797,
-7.32017551193793));
#64061=CARTESIAN_POINT('Ctrl Pts',(-0.235923423345702,-0.707975361839259,
-7.29899338061208));
#64062=CARTESIAN_POINT('Ctrl Pts',(0.270717601992387,-0.695613702123204,
-7.27781124928622));
#64063=CARTESIAN_POINT('Ctrl Pts',(0.600862087662645,-0.366328813167557,
-7.25662911796036));
#64064=CARTESIAN_POINT('Ctrl Pts',(0.741976258067605,0.0756984368513641,
-7.23544698663451));
#64065=CARTESIAN_POINT('Ctrl Pts',(0.467284115457725,0.650445070613317,
-7.20896932247717));
#64066=CARTESIAN_POINT('Ctrl Pts',(-0.295637994600642,0.743691972604572,
-7.1771961254884));
#64067=CARTESIAN_POINT('Ctrl Pts',(-0.651899538900863,0.313748973069414,
-7.15393369186899));
#64068=CARTESIAN_POINT('Ctrl Pts',(-0.677372917166972,0.0445104750611548,
-7.14126232391253));
#64069=CARTESIAN_POINT('Ctrl Pts',(-0.677180734722105,0.000258105871726134,
-7.13918202161899));
#64070=CARTESIAN_POINT('Origin',(0.,0.,-12.278617978381));
#64071=CARTESIAN_POINT('',(-0.676392201347069,0.0008047333580961,-7.578617978381));
#64072=CARTESIAN_POINT('',(-0.6767,7.06659665679343E-14,-7.53918202161899));
#64073=CARTESIAN_POINT('',(-0.6767,6.12423655037739E-13,-12.278617978381));
#64074=CARTESIAN_POINT('Ctrl Pts',(-0.676392201347069,0.000804733358096152,
-7.578617978381));
#64075=CARTESIAN_POINT('Ctrl Pts',(-0.674918865337116,-0.160046296534286,
-7.57106932309937));
#64076=CARTESIAN_POINT('Ctrl Pts',(-0.536787257819588,-0.549167815545202,
-7.55292960215482));
#64077=CARTESIAN_POINT('Ctrl Pts',(-0.00975058277995205,-0.745777183371727,
-7.5294943483788));
#64078=CARTESIAN_POINT('Ctrl Pts',(0.419849643624006,-0.565646721170082,
-7.50831221705293));
#64079=CARTESIAN_POINT('Ctrl Pts',(0.640628155804832,-0.296569284182963,
-7.49242561855854));
#64080=CARTESIAN_POINT('Ctrl Pts',(0.702987671893402,0.0451467467366845,
-7.47653902006416));
#64081=CARTESIAN_POINT('Ctrl Pts',(0.562342884997569,0.490570539624217,
-7.45535688873828));
#64082=CARTESIAN_POINT('Ctrl Pts',(0.119401435125199,0.736824090200709,
-7.43417475741245));
#64083=CARTESIAN_POINT('Ctrl Pts',(-0.332123683053873,0.620423973506661,
-7.41299262608657));
#64084=CARTESIAN_POINT('Ctrl Pts',(-0.605606017960123,0.375687041846724,
-7.39623887735325));
#64085=CARTESIAN_POINT('Ctrl Pts',(-0.674812100430787,0.130937563943502,
-7.3847806614514));
#64086=CARTESIAN_POINT('Ctrl Pts',(-0.675588369597491,-0.000390811426926201,
-7.37861797838101));
#64087=CARTESIAN_POINT('Ctrl Pts',(-0.676577157036262,2.11996792289677E-5,
-7.53918202161899));
#64088=CARTESIAN_POINT('Ctrl Pts',(-0.676832809338945,-0.0887511003222832,
-7.53502177853434));
#64089=CARTESIAN_POINT('Ctrl Pts',(-0.617002632935423,-0.403960088726185,
-7.52027046978677));
#64090=CARTESIAN_POINT('Ctrl Pts',(-0.243968745432271,-0.705440071063631,
-7.50022362820774));
#64091=CARTESIAN_POINT('Ctrl Pts',(0.22082772031363,-0.66818198545617,-7.47904149688187));
#64092=CARTESIAN_POINT('Ctrl Pts',(0.614531056354557,-0.422623475038358,
-7.45785936555602));
#64093=CARTESIAN_POINT('Ctrl Pts',(0.777226853872599,0.193265755020321,
-7.43138170139868));
#64094=CARTESIAN_POINT('Ctrl Pts',(0.256098235933003,0.758217163825756,
-7.39960850440991));
#64095=CARTESIAN_POINT('Ctrl Pts',(-0.369765439283066,0.64772849328574,
-7.37313084025257));
#64096=CARTESIAN_POINT('Ctrl Pts',(-0.635001886562817,0.292949972624209,
-7.35298867932228));
#64097=CARTESIAN_POINT('Ctrl Pts',(-0.67654467369993,0.0899947722476126,
-7.34343758405491));
#64098=CARTESIAN_POINT('Ctrl Pts',(-0.676774544010776,-0.00025420799175294,
-7.339182021619));
#64099=CARTESIAN_POINT('Origin',(0.,0.,-12.278617978381));
#64100=CARTESIAN_POINT('',(-0.677890574183207,-0.000373347607181736,-7.778617978381));
#64101=CARTESIAN_POINT('',(-0.67644239189479,4.75998292377457E-5,-7.73918202161899));
#64102=CARTESIAN_POINT('',(-0.6767,6.12423655037739E-13,-12.278617978381));
#64103=CARTESIAN_POINT('Ctrl Pts',(-0.677890574183207,-0.00037334760718182,
-7.778617978381));
#64104=CARTESIAN_POINT('Ctrl Pts',(-0.677891800033195,-0.00201980826256494,
-7.77854011607321));
#64105=CARTESIAN_POINT('Ctrl Pts',(-0.677156403482296,-0.227613571077705,
-7.76787118810249));
#64106=CARTESIAN_POINT('Ctrl Pts',(-0.490212471272208,-0.562112456819458,
-7.75190672730032));
#64107=CARTESIAN_POINT('Ctrl Pts',(-0.0461672328563757,-0.702921420239883,
-7.73072459597445));
#64108=CARTESIAN_POINT('Ctrl Pts',(0.296296052364626,-0.640754573673755,
-7.71483799748007));
#64109=CARTESIAN_POINT('Ctrl Pts',(0.565036603409811,-0.420670336941072,
-7.69895139898565));
#64110=CARTESIAN_POINT('Ctrl Pts',(0.746184610028158,0.00987433095006524,
-7.67776926765981));
#64111=CARTESIAN_POINT('Ctrl Pts',(0.56799153737738,0.484305746484325,-7.65658713633396));
#64112=CARTESIAN_POINT('Ctrl Pts',(0.148491341379806,0.687882525786409,
-7.63540500500808));
#64113=CARTESIAN_POINT('Ctrl Pts',(-0.315358990972195,0.675875526773047,
-7.61422287368224));
#64114=CARTESIAN_POINT('Ctrl Pts',(-0.638876986888255,0.355359411367687,
-7.59529386480653));
#64115=CARTESIAN_POINT('Ctrl Pts',(-0.67698601476212,0.0656341400444222,
-7.5816603887623));
#64116=CARTESIAN_POINT('Ctrl Pts',(-0.676392201347069,0.000804733358096152,
-7.578617978381));
#64117=CARTESIAN_POINT('Ctrl Pts',(-0.6767,5.60754863655395E-14,-7.73918202161899));
#64118=CARTESIAN_POINT('Ctrl Pts',(-0.676700000000002,-0.021921959043459,
-7.73815084439303));
#64119=CARTESIAN_POINT('Ctrl Pts',(-0.675631472587797,-0.0438938715230559,
-7.73711731588847));
#64120=CARTESIAN_POINT('Ctrl Pts',(-0.673499468305582,-0.0657370229938853,
-7.73608496302321));
#64121=CARTESIAN_POINT('Ctrl Pts',(-0.654475950121291,-0.260639815954453,
-7.7268734508003));
#64122=CARTESIAN_POINT('Ctrl Pts',(-0.54610007048813,-0.445024264462959,
-7.71766193857739));
#64123=CARTESIAN_POINT('Ctrl Pts',(-0.385067613933398,-0.556458284779407,
-7.70845042635449));
#64124=CARTESIAN_POINT('Ctrl Pts',(-0.224035157378667,-0.667892305095855,
-7.69923891413158));
#64125=CARTESIAN_POINT('Ctrl Pts',(-0.0132876862431723,-0.704340344110886,
-7.69002740190867));
#64126=CARTESIAN_POINT('Ctrl Pts',(0.175816266406146,-0.65346119277812,
-7.68081588968577));
#64127=CARTESIAN_POINT('Ctrl Pts',(0.364920219055463,-0.602582041445354,
-7.67160437746286));
#64128=CARTESIAN_POINT('Ctrl Pts',(0.528926311916782,-0.465305103679348,
-7.66239286523995));
#64129=CARTESIAN_POINT('Ctrl Pts',(0.612302518258926,-0.288111985404596,
-7.65318135301705));
#64130=CARTESIAN_POINT('Ctrl Pts',(0.695678724601069,-0.110918867129844,
-7.64396984079414));
#64131=CARTESIAN_POINT('Ctrl Pts',(0.696902020345894,0.10295366426577,-7.63475832857123));
#64132=CARTESIAN_POINT('Ctrl Pts',(0.615558200808584,0.281088938624948,
-7.62554681634833));
#64133=CARTESIAN_POINT('Ctrl Pts',(0.534214381271273,0.459224212984125,
-7.61633530412542));
#64134=CARTESIAN_POINT('Ctrl Pts',(0.371789345141617,0.598368252656427,
-7.60712379190251));
#64135=CARTESIAN_POINT('Ctrl Pts',(0.183279777547595,0.651407255979011,
-7.5979122796796));
#64136=CARTESIAN_POINT('Ctrl Pts',(-0.00522979004642629,0.704446259301594,
-7.5887007674567));
#64137=CARTESIAN_POINT('Ctrl Pts',(-0.216380405370042,0.6704113685789,-7.57948925523379));
#64138=CARTESIAN_POINT('Ctrl Pts',(-0.378677031806715,0.560826707265316,
-7.57027774301088));
#64139=CARTESIAN_POINT('Ctrl Pts',(-0.540973658243388,0.451242045951731,
-7.56106623078798));
#64140=CARTESIAN_POINT('Ctrl Pts',(-0.651451640998797,0.26810938511718,
-7.55185471856507));
#64141=CARTESIAN_POINT('Ctrl Pts',(-0.672703429020755,0.0734369565254355,
-7.54264320634216));
#64142=CARTESIAN_POINT('Ctrl Pts',(-0.675365183944437,0.0490545236320713,
-7.54148947810111));
#64143=CARTESIAN_POINT('Ctrl Pts',(-0.676699999999998,0.0244983809836534,
-7.54033439000418));
#64144=CARTESIAN_POINT('Ctrl Pts',(-0.6767,7.06659581420018E-14,-7.53918202161899));
#64145=CARTESIAN_POINT('Origin',(0.,0.,-12.278617978381));
#64146=CARTESIAN_POINT('',(-0.675799427295481,-0.000196415820169861,-7.978617978381));
#64147=CARTESIAN_POINT('',(-0.677536114604909,0.000301369397225656,-7.93918202161899));
#64148=CARTESIAN_POINT('',(-0.6767,6.12423655037739E-13,-12.278617978381));
#64149=CARTESIAN_POINT('Ctrl Pts',(-0.67579942729548,-0.000196415820169965,
-7.978617978381));
#64150=CARTESIAN_POINT('Ctrl Pts',(-0.676291431262014,-0.0682707116028679,
-7.97541984338411));
#64151=CARTESIAN_POINT('Ctrl Pts',(-0.651210353376953,-0.248880751939011,
-7.96692617555577));
#64152=CARTESIAN_POINT('Ctrl Pts',(-0.490226125422572,-0.505873781070776,
-7.95313697489597));
#64153=CARTESIAN_POINT('Ctrl Pts',(-0.188959895740458,-0.680185218989984,
-7.93725037640156));
#64154=CARTESIAN_POINT('Ctrl Pts',(0.158343748144318,-0.68640888178885,
-7.92136377790718));
#64155=CARTESIAN_POINT('Ctrl Pts',(0.57512722912829,-0.475518290888796,
-7.9001816465813));
#64156=CARTESIAN_POINT('Ctrl Pts',(0.746434431978506,0.00144269434815235,
-7.87899951525548));
#64157=CARTESIAN_POINT('Ctrl Pts',(0.558481156467344,0.428171514253297,
-7.85781738392959));
#64158=CARTESIAN_POINT('Ctrl Pts',(0.197165933085699,0.719294526399437,
-7.83663525260375));
#64159=CARTESIAN_POINT('Ctrl Pts',(-0.436112882427935,0.670670210164639,
-7.81023545075422));
#64160=CARTESIAN_POINT('Ctrl Pts',(-0.67772505622498,0.221936729982677,
-7.78913118173614));
#64161=CARTESIAN_POINT('Ctrl Pts',(-0.677890574183207,-0.00037334760718182,
-7.778617978381));
#64162=CARTESIAN_POINT('Ctrl Pts',(-0.677536114604909,0.000301369397225706,
-7.93918202161899));
#64163=CARTESIAN_POINT('Ctrl Pts',(-0.677582832650084,-0.107871171142427,
-7.93407676598763));
#64164=CARTESIAN_POINT('Ctrl Pts',(-0.620875575886241,-0.329206785654903,
-7.92367597752479));
#64165=CARTESIAN_POINT('Ctrl Pts',(-0.317576031167041,-0.674836636013439,
-7.90268412339904));
#64166=CARTESIAN_POINT('Ctrl Pts',(0.316526456894863,-0.73569303145392,
-7.87620645924171));
#64167=CARTESIAN_POINT('Ctrl Pts',(0.789672444363271,-0.129988478648325,
-7.84443326225293));
#64168=CARTESIAN_POINT('Ctrl Pts',(0.579332529080104,0.469736630306881,
-7.81795559809561));
#64169=CARTESIAN_POINT('Ctrl Pts',(0.166006120765101,0.684596161463233,
-7.79677346676974));
#64170=CARTESIAN_POINT('Ctrl Pts',(-0.182044780093774,0.68206852468891,
-7.78088686827537));
#64171=CARTESIAN_POINT('Ctrl Pts',(-0.484541134815908,0.511321605495331,
-7.76500026978095));
#64172=CARTESIAN_POINT('Ctrl Pts',(-0.650114110956395,0.253328034721966,
-7.75109865422884));
#64173=CARTESIAN_POINT('Ctrl Pts',(-0.676353652975621,0.0705349586336249,
-7.74249257150818));
#64174=CARTESIAN_POINT('Ctrl Pts',(-0.675796937800043,0.000166864340071023,
-7.73918202161899));
#64175=CARTESIAN_POINT('Origin',(0.,0.,-12.278617978381));
#64176=CARTESIAN_POINT('',(-0.676581765607971,3.46312420244521E-5,-8.178617978381));
#64177=CARTESIAN_POINT('',(-0.676757248046547,-0.000512325571017325,-8.139182021619));
#64178=CARTESIAN_POINT('',(-0.6767,6.12423655037739E-13,-12.278617978381));
#64179=CARTESIAN_POINT('Ctrl Pts',(-0.676581765607971,3.46312420244597E-5,
-8.178617978381));
#64180=CARTESIAN_POINT('Ctrl Pts',(-0.676517670152724,-0.0217651188480246,
-8.17759510352649));
#64181=CARTESIAN_POINT('Ctrl Pts',(-0.66971641899371,-0.156406801086305,
-8.17127669584052));
#64182=CARTESIAN_POINT('Ctrl Pts',(-0.584343046747153,-0.396107280984521,
-8.15966275532308));
#64183=CARTESIAN_POINT('Ctrl Pts',(-0.323660302086688,-0.625678754975878,
-8.14377615682868));
#64184=CARTESIAN_POINT('Ctrl Pts',(0.130528774517201,-0.734745679590988,
-8.12259402550284));
#64185=CARTESIAN_POINT('Ctrl Pts',(0.569859400741034,-0.482106529718409,
-8.10141189417698));
#64186=CARTESIAN_POINT('Ctrl Pts',(0.702847075744717,-0.0351857338159052,
-8.08022976285111));
#64187=CARTESIAN_POINT('Ctrl Pts',(0.615915117961009,0.420603837767584,
-8.05904763152526));
#64188=CARTESIAN_POINT('Ctrl Pts',(0.100242323565696,0.794597200479857,
-8.03256996736792));
#64189=CARTESIAN_POINT('Ctrl Pts',(-0.542739842833042,0.540862840079443,
-8.00399490537604));
#64190=CARTESIAN_POINT('Ctrl Pts',(-0.674662092187505,0.157166719054403,
-7.98601090904705));
#64191=CARTESIAN_POINT('Ctrl Pts',(-0.67579942729548,-0.000196415820169965,
-7.978617978381));
#64192=CARTESIAN_POINT('Ctrl Pts',(-0.676757248046547,-0.000512325571017335,
-8.139182021619));
#64193=CARTESIAN_POINT('Ctrl Pts',(-0.677077249127755,-0.0627978904691677,
-8.13625202613001));
#64194=CARTESIAN_POINT('Ctrl Pts',(-0.639251224563342,-0.349588008735834,
-8.12273096497808));
#64195=CARTESIAN_POINT('Ctrl Pts',(-0.234999107869971,-0.765642641017721,
-8.09861883816322));
#64196=CARTESIAN_POINT('Ctrl Pts',(0.517732728409698,-0.610272394838091,
-8.06684564117445));
#64197=CARTESIAN_POINT('Ctrl Pts',(0.745647079045141,-0.0170033706618007,
-8.04036797701711));
#64198=CARTESIAN_POINT('Ctrl Pts',(0.569703324557914,0.414328442674807,
-8.01918584569126));
#64199=CARTESIAN_POINT('Ctrl Pts',(0.302785852511827,0.637713495113113,
-8.00329924719686));
#64200=CARTESIAN_POINT('Ctrl Pts',(-0.0383075228840123,0.70339350954178,
-7.98741264870248));
#64201=CARTESIAN_POINT('Ctrl Pts',(-0.485078126151442,0.567087459025494,
-7.96623051737661));
#64202=CARTESIAN_POINT('Ctrl Pts',(-0.675241177176038,0.232736134400955,
-7.95015364168212));
#64203=CARTESIAN_POINT('Ctrl Pts',(-0.677534373383808,0.00433305157491817,
-7.93937229881909));
#64204=CARTESIAN_POINT('Ctrl Pts',(-0.677536114604909,0.000301369397225706,
-7.93918202161899));
#64205=CARTESIAN_POINT('Origin',(0.,0.,-12.278617978381));
#64206=CARTESIAN_POINT('',(-0.6767,3.91279890432639E-14,-8.378617978381));
#64207=CARTESIAN_POINT('',(-0.675338277625542,0.000119265976971927,-8.33918202161899));
#64208=CARTESIAN_POINT('',(-0.6767,6.12423655037739E-13,-12.278617978381));
#64209=CARTESIAN_POINT('Ctrl Pts',(-0.676800963596304,0.00021576680758149,
-8.378617978381));
#64210=CARTESIAN_POINT('Ctrl Pts',(-0.676608873861011,-0.0875972287274319,
-8.3744748308374));
#64211=CARTESIAN_POINT('Ctrl Pts',(-0.636733335774834,-0.287882668666046,
-8.36503615046233));
#64212=CARTESIAN_POINT('Ctrl Pts',(-0.376151562716211,-0.644514527780979,
-8.34500640442435));
#64213=CARTESIAN_POINT('Ctrl Pts',(0.122248771729135,-0.736357033252738,
-8.32382427309847));
#64214=CARTESIAN_POINT('Ctrl Pts',(0.512926016390591,-0.481808000615124,
-8.30264214177264));
#64215=CARTESIAN_POINT('Ctrl Pts',(0.741723760032622,-0.0781337614659248,
-8.28146001044675));
#64216=CARTESIAN_POINT('Ctrl Pts',(0.590788201416899,0.540742577860168,
-8.25498234628945));
#64217=CARTESIAN_POINT('Ctrl Pts',(-0.136775462740103,0.788525235335051,
-8.22320914930065));
#64218=CARTESIAN_POINT('Ctrl Pts',(-0.614839420141264,0.408047756448488,
-8.19775435999784));
#64219=CARTESIAN_POINT('Ctrl Pts',(-0.676849499199172,0.0910945255265748,
-8.18289063635796));
#64220=CARTESIAN_POINT('Ctrl Pts',(-0.676581765607971,3.46312420244597E-5,
-8.178617978381));
#64221=CARTESIAN_POINT('Ctrl Pts',(-0.675338277625542,0.000119265976971872,
-8.33918202161899));
#64222=CARTESIAN_POINT('Ctrl Pts',(-0.675125560369215,-0.12890170738665,
-8.33313175344091));
#64223=CARTESIAN_POINT('Ctrl Pts',(-0.578388002552477,-0.48415351739988,
-8.31649041959989));
#64224=CARTESIAN_POINT('Ctrl Pts',(-0.000450182530976969,-0.800299550983042,
-8.28925802009595));
#64225=CARTESIAN_POINT('Ctrl Pts',(0.55731818268824,-0.495656256237618,
-8.26278035593863));
#64226=CARTESIAN_POINT('Ctrl Pts',(0.70243916327569,-0.0530014935470479,
-8.24159822461277));
#64227=CARTESIAN_POINT('Ctrl Pts',(0.643605972302399,0.290050214182614,
-8.22571162611838));
#64228=CARTESIAN_POINT('Ctrl Pts',(0.426145850537514,0.56091854100633,-8.20982502762398));
#64229=CARTESIAN_POINT('Ctrl Pts',(-0.00261665234877711,0.746245353610373,
-8.18864289629813));
#64230=CARTESIAN_POINT('Ctrl Pts',(-0.478758691882225,0.5726749143775,-8.16746076497226));
#64231=CARTESIAN_POINT('Ctrl Pts',(-0.657683237969969,0.212924793057815,
-8.1492086291354));
#64232=CARTESIAN_POINT('Ctrl Pts',(-0.676498894574648,0.0497740418370898,
-8.14154755896147));
#64233=CARTESIAN_POINT('Ctrl Pts',(-0.676757248046547,-0.000512325571017335,
-8.139182021619));
#64234=CARTESIAN_POINT('Origin',(0.,0.,-12.278617978381));
#64235=CARTESIAN_POINT('',(-0.6767,2.45376068294393E-14,-8.578617978381));
#64236=CARTESIAN_POINT('',(-0.677509650187365,0.000766222167987149,-8.539182021619));
#64237=CARTESIAN_POINT('',(-0.6767,6.12423655037739E-13,-12.278617978381));
#64238=CARTESIAN_POINT('Ctrl Pts',(-0.6767,1.49211214436621E-14,-8.578617978381));
#64239=CARTESIAN_POINT('Ctrl Pts',(-0.676700000000002,-0.0956161613166699,
-8.57412033253705));
#64240=CARTESIAN_POINT('Ctrl Pts',(-0.65612415604488,-0.191237609808786,
-8.56962003485022));
#64241=CARTESIAN_POINT('Ctrl Pts',(-0.616773580775826,-0.278411996970255,
-8.56512106308482));
#64242=CARTESIAN_POINT('Ctrl Pts',(-0.536204436542128,-0.45689898793987,
-8.55590955086192));
#64243=CARTESIAN_POINT('Ctrl Pts',(-0.374385443722978,-0.596747369056862,
-8.54669803863901));
#64244=CARTESIAN_POINT('Ctrl Pts',(-0.186108082793701,-0.650604850519002,
-8.5374865264161));
#64245=CARTESIAN_POINT('Ctrl Pts',(0.00216927813557544,-0.704462331981142,
-8.5282750141932));
#64246=CARTESIAN_POINT('Ctrl Pts',(0.213465765134057,-0.671345105041863,
-8.51906350197029));
#64247=CARTESIAN_POINT('Ctrl Pts',(0.376236949824165,-0.562466574639782,
-8.50985198974738));
#64248=CARTESIAN_POINT('Ctrl Pts',(0.539008134514272,-0.453588044237701,
-8.50064047752448));
#64249=CARTESIAN_POINT('Ctrl Pts',(0.650280693397769,-0.270937082626308,
-8.49142896530157));
#64250=CARTESIAN_POINT('Ctrl Pts',(0.672378034059336,-0.0763588194939005,
-8.48221745307866));
#64251=CARTESIAN_POINT('Ctrl Pts',(0.694475374720904,0.118219443638507,
-8.47300594085575));
#64252=CARTESIAN_POINT('Ctrl Pts',(0.62699384744599,0.321170668356893,-8.46379442863285));
#64253=CARTESIAN_POINT('Ctrl Pts',(0.492782517846198,0.463776109890496,
-8.45458291640994));
#64254=CARTESIAN_POINT('Ctrl Pts',(0.358571188246407,0.6063815514241,-8.44537140418703));
#64255=CARTESIAN_POINT('Ctrl Pts',(0.160081680058386,0.686036251708044,
-8.43615989196413));
#64256=CARTESIAN_POINT('Ctrl Pts',(-0.0354779872946126,0.675769341134624,
-8.42694837974122));
#64257=CARTESIAN_POINT('Ctrl Pts',(-0.231037654647611,0.665502430561203,
-8.41773686751831));
#64258=CARTESIAN_POINT('Ctrl Pts',(-0.420095214026566,0.565501453667373,
-8.40852535529541));
#64259=CARTESIAN_POINT('Ctrl Pts',(-0.538636278782801,0.409626475192969,
-8.3993138430725));
#64260=CARTESIAN_POINT('Ctrl Pts',(-0.627413227207555,0.292889672185607,
-8.39241522150867));
#64261=CARTESIAN_POINT('Ctrl Pts',(-0.676699999999992,0.146509960619025,
-8.38550959488601));
#64262=CARTESIAN_POINT('Ctrl Pts',(-0.6767,3.91280786059017E-14,-8.378617978381));
#64263=CARTESIAN_POINT('Ctrl Pts',(-0.677509650187365,0.000766222167987083,
-8.539182021619));
#64264=CARTESIAN_POINT('Ctrl Pts',(-0.675844325969005,-0.193734978521912,
-8.53001148075182));
#64265=CARTESIAN_POINT('Ctrl Pts',(-0.485030615819685,-0.6166037500008,
-8.5102498742217));
#64266=CARTESIAN_POINT('Ctrl Pts',(0.10391852221122,-0.738565922476695,
-8.48519273486015));
#64267=CARTESIAN_POINT('Ctrl Pts',(0.501082034024498,-0.495122945943268,
-8.46401060353428));
#64268=CARTESIAN_POINT('Ctrl Pts',(0.678315270358112,-0.195566276054168,
-8.44812400503989));
#64269=CARTESIAN_POINT('Ctrl Pts',(0.687916430292161,0.151660411805788,
-8.43223740654549));
#64270=CARTESIAN_POINT('Ctrl Pts',(0.481089349371821,0.570475251501399,
-8.41105527521963));
#64271=CARTESIAN_POINT('Ctrl Pts',(0.00581701517587562,0.746413159680681,
-8.38987314389378));
#64272=CARTESIAN_POINT('Ctrl Pts',(-0.422719610264708,0.562619035266954,
-8.36869101256792));
#64273=CARTESIAN_POINT('Ctrl Pts',(-0.63318944003504,0.306541419473106,
-8.35355914942015));
#64274=CARTESIAN_POINT('Ctrl Pts',(-0.675497924430293,0.096951025181312,
-8.34372281910384));
#64275=CARTESIAN_POINT('Ctrl Pts',(-0.675338277625542,0.000119265976971872,
-8.33918202161899));
#64276=CARTESIAN_POINT('Origin',(0.,0.,-12.278617978381));
#64277=CARTESIAN_POINT('',(-0.6767,2.91801058245312E-14,-8.778617978381));
#64278=CARTESIAN_POINT('',(-0.67719182899154,-0.000898131385783873,-8.73918202161899));
#64279=CARTESIAN_POINT('',(-0.6767,6.12423655037739E-13,-12.278617978381));
#64280=CARTESIAN_POINT('Ctrl Pts',(-0.6767,3.87965912103085E-14,-8.778617978381));
#64281=CARTESIAN_POINT('Ctrl Pts',(-0.676700000000008,-0.141987090474437,
-8.77193911114168));
#64282=CARTESIAN_POINT('Ctrl Pts',(-0.630506051029792,-0.28387092797994,
-8.76524787263758));
#64283=CARTESIAN_POINT('Ctrl Pts',(-0.546771726394805,-0.398702356671295,
-8.75856281976587));
#64284=CARTESIAN_POINT('Ctrl Pts',(-0.431391972538878,-0.556931637615385,
-8.74935130754296));
#64285=CARTESIAN_POINT('Ctrl Pts',(-0.244385431591964,-0.660717521921091,
-8.74013979532005));
#64286=CARTESIAN_POINT('Ctrl Pts',(-0.0490720208180517,-0.674918385268051,
-8.73092828309715));
#64287=CARTESIAN_POINT('Ctrl Pts',(0.14624138995586,-0.68911924861501,-8.72171677087424));
#64288=CARTESIAN_POINT('Ctrl Pts',(0.346293901759852,-0.613475685379523,
-8.71250525865133));
#64289=CARTESIAN_POINT('Ctrl Pts',(0.483348266304422,-0.473600404835669,
-8.70329374642843));
#64290=CARTESIAN_POINT('Ctrl Pts',(0.620402630848992,-0.333725124291814,
-8.69408223420552));
#64291=CARTESIAN_POINT('Ctrl Pts',(0.69195529098788,-0.132173212951097,
-8.68487072198261));
#64292=CARTESIAN_POINT('Ctrl Pts',(0.67377870635233,0.0628103882027554,
-8.6756592097597));
#64293=CARTESIAN_POINT('Ctrl Pts',(0.65560212171678,0.257793989356608,-8.6664476975368));
#64294=CARTESIAN_POINT('Ctrl Pts',(0.548028321998149,0.442647536123078,
-8.65723618531389));
#64295=CARTESIAN_POINT('Ctrl Pts',(0.387481509598483,0.554780109339981,
-8.64802467309099));
#64296=CARTESIAN_POINT('Ctrl Pts',(0.226934697198816,0.666912682556885,
-8.63881316086808));
#64297=CARTESIAN_POINT('Ctrl Pts',(0.0163475632500464,0.704275968725133,
-8.62960164864517));
#64298=CARTESIAN_POINT('Ctrl Pts',(-0.17297564892576,0.654218858547132,
-8.62039013642226));
#64299=CARTESIAN_POINT('Ctrl Pts',(-0.362298861101567,0.604161748369132,
-8.61117862419936));
#64300=CARTESIAN_POINT('Ctrl Pts',(-0.526899805012704,0.467598629623219,
-8.60196711197645));
#64301=CARTESIAN_POINT('Ctrl Pts',(-0.611045038945032,0.290769411012686,
-8.59275559975354));
#64302=CARTESIAN_POINT('Ctrl Pts',(-0.654093108536358,0.200304911090468,
-8.58804305929603));
#64303=CARTESIAN_POINT('Ctrl Pts',(-0.676699999999998,0.100155113678007,
-8.58332912997485));
#64304=CARTESIAN_POINT('Ctrl Pts',(-0.6767,1.49211214436621E-14,-8.578617978381));
#64305=CARTESIAN_POINT('Ctrl Pts',(-0.67719182899154,-0.000898131385784005,
-8.73918202161899));
#64306=CARTESIAN_POINT('Ctrl Pts',(-0.677515066866202,-0.0369757515937125,
-8.73748227372565));
#64307=CARTESIAN_POINT('Ctrl Pts',(-0.6585483635347,-0.297371631309851,
-8.72519146016938));
#64308=CARTESIAN_POINT('Ctrl Pts',(-0.398906696132759,-0.630200070519562,
-8.70760511378165));
#64309=CARTESIAN_POINT('Ctrl Pts',(0.061401085864204,-0.701754831174225,
-8.68642298245581));
#64310=CARTESIAN_POINT('Ctrl Pts',(0.390405367007379,-0.588167853373958,
-8.67053638396139));
#64311=CARTESIAN_POINT('Ctrl Pts',(0.622501320628285,-0.329730194842773,
-8.65464978546701));
#64312=CARTESIAN_POINT('Ctrl Pts',(0.735980420215885,0.123376641684858,
-8.63346765414115));
#64313=CARTESIAN_POINT('Ctrl Pts',(0.487626042973425,0.565143596640834,
-8.61228552281528));
#64314=CARTESIAN_POINT('Ctrl Pts',(0.0420197908343311,0.702471625708329,
-8.59110339148945));
#64315=CARTESIAN_POINT('Ctrl Pts',(-0.414593702842348,0.619976678949471,
-8.56992126016356));
#64316=CARTESIAN_POINT('Ctrl Pts',(-0.662321132177836,0.285300701931316,
-8.55261413687343));
#64317=CARTESIAN_POINT('Ctrl Pts',(-0.677767610364351,0.0308946281568698,
-8.54060254641475));
#64318=CARTESIAN_POINT('Ctrl Pts',(-0.677509650187365,0.000766222167987083,
-8.539182021619));
#64319=CARTESIAN_POINT('Origin',(0.,0.,-12.278617978381));
#64320=CARTESIAN_POINT('',(-0.6767,3.38226048196233E-14,-8.978617978381));
#64321=CARTESIAN_POINT('',(-0.675362603300994,0.000190139876870055,-8.93918202161899));
#64322=CARTESIAN_POINT('',(-0.6767,6.12423655037739E-13,-12.278617978381));
#64323=CARTESIAN_POINT('Ctrl Pts',(-0.6767,2.42061194338461E-14,-8.978617978381));
#64324=CARTESIAN_POINT('Ctrl Pts',(-0.676700000000007,-0.188486775366012,
-8.96975183326294));
#64325=CARTESIAN_POINT('Ctrl Pts',(-0.593581982928983,-0.375700115386127,
-8.96087571042494));
#64326=CARTESIAN_POINT('Ctrl Pts',(-0.453641556933961,-0.502127700712211,
-8.95200457644691));
#64327=CARTESIAN_POINT('Ctrl Pts',(-0.308331729833587,-0.633406210362486,
-8.942793064224));
#64328=CARTESIAN_POINT('Ctrl Pts',(-0.104047973338697,-0.696739479426886,
-8.9335815520011));
#64329=CARTESIAN_POINT('Ctrl Pts',(0.0900397760654122,-0.670683031488117,
-8.92437003977819));
#64330=CARTESIAN_POINT('Ctrl Pts',(0.284127525469521,-0.644626583549348,
-8.91515852755528));
#64331=CARTESIAN_POINT('Ctrl Pts',(0.464473888008647,-0.529656388903286,
-8.90594701533237));
#64332=CARTESIAN_POINT('Ctrl Pts',(0.570014065109352,-0.364701049597491,
-8.89673550310947));
#64333=CARTESIAN_POINT('Ctrl Pts',(0.675554242210057,-0.199745710291696,
-8.88752399088656));
#64334=CARTESIAN_POINT('Ctrl Pts',(0.704360342954921,0.012181552461174,
-8.87831247866365));
#64335=CARTESIAN_POINT('Ctrl Pts',(0.646678698265703,0.199322731291181,
-8.86910096644075));
#64336=CARTESIAN_POINT('Ctrl Pts',(0.588997053576484,0.386463910121188,
-8.85988945421784));
#64337=CARTESIAN_POINT('Ctrl Pts',(0.445881327772811,0.54540051750204,-8.85067794199493));
#64338=CARTESIAN_POINT('Ctrl Pts',(0.26579012487558,0.622317040999701,-8.84146642977203));
#64339=CARTESIAN_POINT('Ctrl Pts',(0.0856989219783484,0.699233564497362,
-8.83225491754912));
#64340=CARTESIAN_POINT('Ctrl Pts',(-0.128078051628479,0.692724978356484,
-8.82304340532621));
#64341=CARTESIAN_POINT('Ctrl Pts',(-0.30315648140067,0.604995072529327,
-8.81383189310331));
#64342=CARTESIAN_POINT('Ctrl Pts',(-0.478234911172861,0.51726516670217,
-8.8046203808804));
#64343=CARTESIAN_POINT('Ctrl Pts',(-0.611416658507033,0.349916493821073,
-8.79540886865749));
#64344=CARTESIAN_POINT('Ctrl Pts',(-0.657606738064317,0.159612869319515,
-8.78619735643459));
#64345=CARTESIAN_POINT('Ctrl Pts',(-0.670275380911006,0.107417924553277,
-8.78367089708339));
#64346=CARTESIAN_POINT('Ctrl Pts',(-0.676699999999997,0.0536606993785083,
-8.78114210001714));
#64347=CARTESIAN_POINT('Ctrl Pts',(-0.6767,3.87965912103085E-14,-8.778617978381));
#64348=CARTESIAN_POINT('Ctrl Pts',(-0.675362603300994,0.000190139876870103,
-8.93918202161899));
#64349=CARTESIAN_POINT('Ctrl Pts',(-0.675434194437074,-0.102521459598344,
-8.93436200103656));
#64350=CARTESIAN_POINT('Ctrl Pts',(-0.62903813993231,-0.318143050274465,
-8.92424644762267));
#64351=CARTESIAN_POINT('Ctrl Pts',(-0.407483346505639,-0.574619229353,-8.90883536137732));
#64352=CARTESIAN_POINT('Ctrl Pts',(-0.0831884995869038,-0.701025996570153,
-8.89294876288291));
#64353=CARTESIAN_POINT('Ctrl Pts',(0.261013149201355,-0.654295064568733,
-8.87706216438852));
#64354=CARTESIAN_POINT('Ctrl Pts',(0.640825685227696,-0.382402165013538,
-8.85588003306267));
#64355=CARTESIAN_POINT('Ctrl Pts',(0.737511168356077,0.11508135887323,-8.8346979017368));
#64356=CARTESIAN_POINT('Ctrl Pts',(0.486773807622215,0.508215808451524,
-8.81351577041096));
#64357=CARTESIAN_POINT('Ctrl Pts',(0.0853438924577135,0.740928769112059,
-8.79233363908507));
#64358=CARTESIAN_POINT('Ctrl Pts',(-0.495149682015662,0.605321926693759,
-8.76755572282111));
#64359=CARTESIAN_POINT('Ctrl Pts',(-0.67550098373734,0.187822552956029,
-8.74807333938859));
#64360=CARTESIAN_POINT('Ctrl Pts',(-0.67719182899154,-0.000898131385784005,
-8.73918202161899));
#64361=CARTESIAN_POINT('Origin',(0.,0.,-12.278617978381));
#64362=CARTESIAN_POINT('',(-0.677457454399445,-0.000117200421055334,-9.17861797838101));
#64363=CARTESIAN_POINT('',(-0.677004582552561,0.000242201296634908,-9.13918202161899));
#64364=CARTESIAN_POINT('',(-0.6767,6.12423655037739E-13,-12.278617978381));
#64365=CARTESIAN_POINT('Ctrl Pts',(-0.677457454399445,-0.000117200421055338,
-9.17861797838101));
#64366=CARTESIAN_POINT('Ctrl Pts',(-0.677485000120747,-0.0157378251760865,
-9.17788033857543));
#64367=CARTESIAN_POINT('Ctrl Pts',(-0.66916109833789,-0.255569895231283,
-9.16655163310692));
#64368=CARTESIAN_POINT('Ctrl Pts',(-0.387077784779294,-0.701144794585703,
-9.14463186197549));
#64369=CARTESIAN_POINT('Ctrl Pts',(0.381518042580854,-0.703508036310348,
-9.11285866498672));
#64370=CARTESIAN_POINT('Ctrl Pts',(0.726298025262084,-0.169616802242028,
-9.08638100082937));
#64371=CARTESIAN_POINT('Ctrl Pts',(0.642587744543107,0.288636323051471,
-9.06519886950353));
#64372=CARTESIAN_POINT('Ctrl Pts',(0.427177008054458,0.562029872978596,
-9.04931227100912));
#64373=CARTESIAN_POINT('Ctrl Pts',(0.106813790756512,0.696290679012175,
-9.03342567251474));
#64374=CARTESIAN_POINT('Ctrl Pts',(-0.358417752115536,0.654542351282965,
-9.01224354118889));
#64375=CARTESIAN_POINT('Ctrl Pts',(-0.647864952636916,0.327011892154612,
-8.99397430981096));
#64376=CARTESIAN_POINT('Ctrl Pts',(-0.67717075072116,0.0512874461424838,
-8.98100061126452));
#64377=CARTESIAN_POINT('Ctrl Pts',(-0.676878116969163,0.000554397463382497,
-8.978617978381));
#64378=CARTESIAN_POINT('Ctrl Pts',(-0.677004582552561,0.000242201296634919,
-9.13918202161899));
#64379=CARTESIAN_POINT('Ctrl Pts',(-0.676751893901764,-0.056062095357369,
-9.13653726117894));
#64380=CARTESIAN_POINT('Ctrl Pts',(-0.654972458078587,-0.225288642313194,
-9.12859696790741));
#64381=CARTESIAN_POINT('Ctrl Pts',(-0.517216387829029,-0.48046329983859,
-9.11536114180443));
#64382=CARTESIAN_POINT('Ctrl Pts',(-0.224617670094119,-0.667665183948138,
-9.09947454331003));
#64383=CARTESIAN_POINT('Ctrl Pts',(0.240882484103758,-0.706303478333916,
-9.07829241198417));
#64384=CARTESIAN_POINT('Ctrl Pts',(0.636622435975274,-0.389715686909015,
-9.05711028065832));
#64385=CARTESIAN_POINT('Ctrl Pts',(0.700009260781494,0.0722432181399054,
-9.03592814933246));
#64386=CARTESIAN_POINT('Ctrl Pts',(0.544690364967499,0.509481527819525,
-9.0147460180066));
#64387=CARTESIAN_POINT('Ctrl Pts',(-0.0219154922400167,0.800595369487078,
-8.98826835384928));
#64388=CARTESIAN_POINT('Ctrl Pts',(-0.58488911759003,0.47170683380819,-8.96131517744292));
#64389=CARTESIAN_POINT('Ctrl Pts',(-0.675276886722274,0.123167471762641,
-8.94495306669949));
#64390=CARTESIAN_POINT('Ctrl Pts',(-0.675362603300994,0.000190139876870103,
-8.93918202161899));
#64391=CARTESIAN_POINT('Origin',(0.,0.,-12.278617978381));
#64392=CARTESIAN_POINT('',(-0.675869510275858,-0.000515265065460229,-9.378617978381));
#64393=CARTESIAN_POINT('',(-0.676863776772284,-0.000147692535406863,-9.33918202161899));
#64394=CARTESIAN_POINT('',(-0.6767,6.12423655037739E-13,-12.278617978381));
#64395=CARTESIAN_POINT('Ctrl Pts',(-0.675869510275858,-0.000515265065460194,
-9.378617978381));
#64396=CARTESIAN_POINT('Ctrl Pts',(-0.676533915652542,-0.0826540124146915,
-9.37476006588634));
#64397=CARTESIAN_POINT('Ctrl Pts',(-0.62509694516892,-0.389649898441223,
-9.36031108772875));
#64398=CARTESIAN_POINT('Ctrl Pts',(-0.164628083532023,-0.783183993759156,
-9.33527104390821));
#64399=CARTESIAN_POINT('Ctrl Pts',(0.443775836884319,-0.599451155391359,
-9.30879337975089));
#64400=CARTESIAN_POINT('Ctrl Pts',(0.676623900661522,-0.195984778682572,
-9.28761124842504));
#64401=CARTESIAN_POINT('Ctrl Pts',(0.689421792526712,0.151839936511941,
-9.27172464993064));
#64402=CARTESIAN_POINT('Ctrl Pts',(0.532157948497518,0.461560194802287,
-9.25583805143624));
#64403=CARTESIAN_POINT('Ctrl Pts',(0.150536857936622,0.730908769311981,
-9.2346559201104));
#64404=CARTESIAN_POINT('Ctrl Pts',(-0.351086430223958,0.658714476175113,
-9.21347378878452));
#64405=CARTESIAN_POINT('Ctrl Pts',(-0.629910032807131,0.305441235120693,
-9.19302929726426));
#64406=CARTESIAN_POINT('Ctrl Pts',(-0.677287248765119,0.0964029928941302,
-9.1831758714069));
#64407=CARTESIAN_POINT('Ctrl Pts',(-0.677457454399445,-0.000117200421055338,
-9.17861797838101));
#64408=CARTESIAN_POINT('Ctrl Pts',(-0.676863776772284,-0.000147692535406885,
-9.33918202161899));
#64409=CARTESIAN_POINT('Ctrl Pts',(-0.67688013367565,-0.0100987013725557,
-9.33871252132131));
#64410=CARTESIAN_POINT('Ctrl Pts',(-0.67431259378526,-0.132268211572331,
-9.33294748819216));
#64411=CARTESIAN_POINT('Ctrl Pts',(-0.603416199871352,-0.363481478631069,
-9.32188692223156));
#64412=CARTESIAN_POINT('Ctrl Pts',(-0.273628850822219,-0.694273884466568,
-9.30070479090568));
#64413=CARTESIAN_POINT('Ctrl Pts',(0.23294438000554,-0.709156793970058,
-9.27952265957983));
#64414=CARTESIAN_POINT('Ctrl Pts',(0.580307452228801,-0.398089573632346,
-9.25834052825398));
#64415=CARTESIAN_POINT('Ctrl Pts',(0.744972095404132,0.0357155140929017,
-9.2371583969281));
#64416=CARTESIAN_POINT('Ctrl Pts',(0.501563565304761,0.624393485234313,
-9.2106807327708));
#64417=CARTESIAN_POINT('Ctrl Pts',(-0.255245053230173,0.758504803392499,
-9.17890753578199));
#64418=CARTESIAN_POINT('Ctrl Pts',(-0.643387444434367,0.338269595953793,
-9.15507463206474));
#64419=CARTESIAN_POINT('Ctrl Pts',(-0.677257845603916,0.0566744863639501,
-9.1418327940104));
#64420=CARTESIAN_POINT('Ctrl Pts',(-0.677004582552561,0.000242201296634919,
-9.13918202161899));
#64421=CARTESIAN_POINT('Origin',(0.,0.,-12.278617978381));
#64422=CARTESIAN_POINT('',(-0.676043544325099,0.00066804154600488,-9.57861797838101));
#64423=CARTESIAN_POINT('',(-0.6767,6.90086009169644E-14,-9.53918202161899));
#64424=CARTESIAN_POINT('',(-0.6767,6.12423655037739E-13,-12.278617978381));
#64425=CARTESIAN_POINT('Ctrl Pts',(-0.676043544325099,0.000668041546004881,
-9.57861797838101));
#64426=CARTESIAN_POINT('Ctrl Pts',(-0.674905073035165,-0.148231709807252,
-9.57163979319725));
#64427=CARTESIAN_POINT('Ctrl Pts',(-0.552970071990971,-0.524995973750943,
-9.55407054235057));
#64428=CARTESIAN_POINT('Ctrl Pts',(-0.0498142904822183,-0.744175528733757,
-9.5312057586724));
#64429=CARTESIAN_POINT('Ctrl Pts',(0.388845301867087,-0.587391919962783,
-9.51002362734656));
#64430=CARTESIAN_POINT('Ctrl Pts',(0.623764909652236,-0.33056786265037,
-9.49413702885215));
#64431=CARTESIAN_POINT('Ctrl Pts',(0.704398011625223,0.00730320432709524,
-9.47825043035776));
#64432=CARTESIAN_POINT('Ctrl Pts',(0.587893373397589,0.459641551831196,
-9.45706829903191));
#64433=CARTESIAN_POINT('Ctrl Pts',(0.158825559311775,0.729342775599619,
-9.43588616770604));
#64434=CARTESIAN_POINT('Ctrl Pts',(-0.298302397103462,0.637375656602442,
-9.4147040363802));
#64435=CARTESIAN_POINT('Ctrl Pts',(-0.594288149775049,0.399868325412857,
-9.39737981754899));
#64436=CARTESIAN_POINT('Ctrl Pts',(-0.674709934164887,0.14284018110295,
-9.38535113154927));
#64437=CARTESIAN_POINT('Ctrl Pts',(-0.675869510275858,-0.000515265065460194,
-9.378617978381));
#64438=CARTESIAN_POINT('Ctrl Pts',(-0.676700480522553,-0.000119391525579517,
-9.53918202161899));
#64439=CARTESIAN_POINT('Ctrl Pts',(-0.676985427297024,-0.0767212178377484,
-9.53559224863222));
#64440=CARTESIAN_POINT('Ctrl Pts',(-0.627680731706276,-0.37935610130508,
-9.5214114099825));
#64441=CARTESIAN_POINT('Ctrl Pts',(-0.281526301655526,-0.691309904519107,
-9.50193503850135));
#64442=CARTESIAN_POINT('Ctrl Pts',(0.184600760711549,-0.679083652352037,
-9.48075290717548));
#64443=CARTESIAN_POINT('Ctrl Pts',(0.590931414136129,-0.455037454134073,
-9.45957077584963));
#64444=CARTESIAN_POINT('Ctrl Pts',(0.786489778819108,0.151218590977907,
-9.43309311169231));
#64445=CARTESIAN_POINT('Ctrl Pts',(0.296474486791864,0.743358898950881,
-9.40131991470351));
#64446=CARTESIAN_POINT('Ctrl Pts',(-0.334422425230761,0.666663575280057,
-9.3748422505462));
#64447=CARTESIAN_POINT('Ctrl Pts',(-0.626382474312723,0.317021538909944,
-9.35412961951802));
#64448=CARTESIAN_POINT('Ctrl Pts',(-0.676695642804777,0.102139553349016,
-9.34400805415277));
#64449=CARTESIAN_POINT('Ctrl Pts',(-0.676863776772284,-0.000147692535406885,
-9.33918202161899));
#64450=CARTESIAN_POINT('Origin',(0.,0.,-12.278617978381));
#64451=CARTESIAN_POINT('',(-0.677843803276718,-0.000108888079095037,-9.778617978381));
#64452=CARTESIAN_POINT('',(-0.6767,6.40345347733506E-14,-9.73918202161899));
#64453=CARTESIAN_POINT('',(-0.6767,6.12423655037739E-13,-12.278617978381));
#64454=CARTESIAN_POINT('Ctrl Pts',(-0.677843803276718,-0.000108888079095024,
-9.778617978381));
#64455=CARTESIAN_POINT('Ctrl Pts',(-0.67702325059819,-0.213595101097744,
-9.76851952050815));
#64456=CARTESIAN_POINT('Ctrl Pts',(-0.509576090600237,-0.538781197494748,
-9.75312552980383));
#64457=CARTESIAN_POINT('Ctrl Pts',(-0.0838752645359608,-0.69942467530156,
-9.73243600626807));
#64458=CARTESIAN_POINT('Ctrl Pts',(0.261433978866206,-0.655751514695071,
-9.71654940777366));
#64459=CARTESIAN_POINT('Ctrl Pts',(0.541613442530161,-0.450427324266235,
-9.70066280927928));
#64460=CARTESIAN_POINT('Ctrl Pts',(0.745637002453177,-0.0302396300775194,
-9.6794806779534));
#64461=CARTESIAN_POINT('Ctrl Pts',(0.593197195641168,0.453082254887026,
-9.65829854662756));
#64462=CARTESIAN_POINT('Ctrl Pts',(0.185243328053068,0.678908651556959,
-9.6371164153017));
#64463=CARTESIAN_POINT('Ctrl Pts',(-0.278581983793115,0.691846152828526,
-9.61593428397583));
#64464=CARTESIAN_POINT('Ctrl Pts',(-0.629111894284224,0.380057342876616,
-9.59643480500227));
#64465=CARTESIAN_POINT('Ctrl Pts',(-0.676632975615784,0.0777592896071504,
-9.58223085886018));
#64466=CARTESIAN_POINT('Ctrl Pts',(-0.676043544325099,0.000668041546004881,
-9.57861797838101));
#64467=CARTESIAN_POINT('Ctrl Pts',(-0.6767,8.3267505544905E-14,-9.73918202161899));
#64468=CARTESIAN_POINT('Ctrl Pts',(-0.676700000000012,-0.0950032677258063,
-9.73471320540252));
#64469=CARTESIAN_POINT('Ctrl Pts',(-0.656390733383678,-0.190013320510327,
-9.73024174265372));
#64470=CARTESIAN_POINT('Ctrl Pts',(-0.617527853484026,-0.276734963767522,
-9.72577160317108));
#64471=CARTESIAN_POINT('Ctrl Pts',(-0.537444022855581,-0.455440232351895,
-9.71656009094818));
#64472=CARTESIAN_POINT('Ctrl Pts',(-0.376005648018375,-0.595727820070727,
-9.70734857872527));
#64473=CARTESIAN_POINT('Ctrl Pts',(-0.187875333211616,-0.650096722934845,
-9.69813706650236));
#64474=CARTESIAN_POINT('Ctrl Pts',(0.000254981595142312,-0.704465625798963,
-9.68892555427946));
#64475=CARTESIAN_POINT('Ctrl Pts',(0.211640680406031,-0.671922692982764,
-9.67971404205655));
#64476=CARTESIAN_POINT('Ctrl Pts',(0.374707127961123,-0.563486874962609,
-9.67050252983364));
#64477=CARTESIAN_POINT('Ctrl Pts',(0.537773575516215,-0.455051056942453,
-9.66129101761074));
#64478=CARTESIAN_POINT('Ctrl Pts',(0.649542054782686,-0.272703138992979,
-9.65207950538783));
#64479=CARTESIAN_POINT('Ctrl Pts',(0.672168056022858,-0.0781856410247563,
-9.64286799316492));
#64480=CARTESIAN_POINT('Ctrl Pts',(0.69479405726303,0.116331856943467,-9.63365648094202));
#64481=CARTESIAN_POINT('Ctrl Pts',(0.627864273777154,0.319465704986035,
-9.62444496871911));
#64482=CARTESIAN_POINT('Ctrl Pts',(0.494040952197692,0.462435322560461,
-9.6152334564962));
#64483=CARTESIAN_POINT('Ctrl Pts',(0.360217630618229,0.605404940134888,
-9.6060219442733));
#64484=CARTESIAN_POINT('Ctrl Pts',(0.161945306981591,0.68559871681223,-9.59681043205039));
#64485=CARTESIAN_POINT('Ctrl Pts',(-0.0336415374002855,0.675863253152104,
-9.58759891982748));
#64486=CARTESIAN_POINT('Ctrl Pts',(-0.229228381782162,0.666127789491978,
-9.57838740760458));
#64487=CARTESIAN_POINT('Ctrl Pts',(-0.418556983330429,0.56664092214847,
-9.56917589538167));
#64488=CARTESIAN_POINT('Ctrl Pts',(-0.537521181238947,0.411088639735383,
-9.55996438315876));
#64489=CARTESIAN_POINT('Ctrl Pts',(-0.626987380758105,0.294106625157086,
-9.55303692931217));
#64490=CARTESIAN_POINT('Ctrl Pts',(-0.676699999999985,0.147120594995907,
-9.54610236148133));
#64491=CARTESIAN_POINT('Ctrl Pts',(-0.6767,6.90085211640358E-14,-9.53918202161899));
#64492=CARTESIAN_POINT('Origin',(0.,0.,-12.278617978381));
#64493=CARTESIAN_POINT('',(-0.67610244318158,-0.000267596609132326,-9.978617978381));
#64494=CARTESIAN_POINT('',(-0.677469765816856,0.000446699746677298,-9.93918202161899));
#64495=CARTESIAN_POINT('',(-0.6767,6.12423655037739E-13,-12.278617978381));
#64496=CARTESIAN_POINT('Ctrl Pts',(-0.67610244318158,-0.00026759660913226,
-9.978617978381));
#64497=CARTESIAN_POINT('Ctrl Pts',(-0.676583469304382,-0.0561528993705457,
-9.97599031348199));
#64498=CARTESIAN_POINT('Ctrl Pts',(-0.657565044010056,-0.224499853671964,
-9.96806711575151));
#64499=CARTESIAN_POINT('Ctrl Pts',(-0.516703214563073,-0.478798208519891,
-9.95484838518958));
#64500=CARTESIAN_POINT('Ctrl Pts',(-0.225239754106489,-0.669047701962083,
-9.93896178669518));
#64501=CARTESIAN_POINT('Ctrl Pts',(0.12122757218792,-0.693926344302069,
-9.92307518820078));
#64502=CARTESIAN_POINT('Ctrl Pts',(0.54874197779906,-0.505738288500843,
-9.90189305687493));
#64503=CARTESIAN_POINT('Ctrl Pts',(0.745433350289229,-0.0386725081502612,
-9.88071092554906));
#64504=CARTESIAN_POINT('Ctrl Pts',(0.580683923966688,0.397540222108045,
-9.85952879422322));
#64505=CARTESIAN_POINT('Ctrl Pts',(0.235535653683076,0.707659506204665,
-9.83834666289734));
#64506=CARTESIAN_POINT('Ctrl Pts',(-0.401313885472845,0.693094798545597,
-9.81186899874004));
#64507=CARTESIAN_POINT('Ctrl Pts',(-0.672947296769713,0.244628003099024,
-9.79019425962409));
#64508=CARTESIAN_POINT('Ctrl Pts',(-0.677883830243875,0.0103050754123359,
-9.77911058617108));
#64509=CARTESIAN_POINT('Ctrl Pts',(-0.677843803276718,-0.000108888079095024,
-9.778617978381));
#64510=CARTESIAN_POINT('Ctrl Pts',(-0.677469765816856,0.000446699746677286,
-9.93918202161899));
#64511=CARTESIAN_POINT('Ctrl Pts',(-0.67720463427496,-0.0957460685350012,
-9.9346472360855));
#64512=CARTESIAN_POINT('Ctrl Pts',(-0.629944124500754,-0.305187579010285,
-9.92481691772054));
#64513=CARTESIAN_POINT('Ctrl Pts',(-0.353382605913268,-0.65679506295015,
-9.90439553369265));
#64514=CARTESIAN_POINT('Ctrl Pts',(0.276533191529025,-0.751639959307012,
-9.87791786953533));
#64515=CARTESIAN_POINT('Ctrl Pts',(0.781545819003339,-0.172237355896938,
-9.84614467254655));
#64516=CARTESIAN_POINT('Ctrl Pts',(0.603738860340227,0.437924730538819,
-9.8196670083892));
#64517=CARTESIAN_POINT('Ctrl Pts',(0.202556190221955,0.674685798149359,
-9.79848487706338));
#64518=CARTESIAN_POINT('Ctrl Pts',(-0.145127604936405,0.690865944026855,
-9.78259827856895));
#64519=CARTESIAN_POINT('Ctrl Pts',(-0.456362724825398,0.536621802543421,
-9.76671168007457));
#64520=CARTESIAN_POINT('Ctrl Pts',(-0.642914547871936,0.277692214258572,
-9.75223959442458));
#64521=CARTESIAN_POINT('Ctrl Pts',(-0.676032577839247,0.0826491836746199,
-9.74306304160606));
#64522=CARTESIAN_POINT('Ctrl Pts',(-0.675534132712119,0.000105302539254004,
-9.73918202161899));
#64523=CARTESIAN_POINT('Origin',(0.,0.,-12.278617978381));
#64524=CARTESIAN_POINT('',(-0.6767,8.09105386856412E-14,-10.178617978381));
#64525=CARTESIAN_POINT('',(-0.676977044559859,-0.000480244224215359,-10.139182021619));
#64526=CARTESIAN_POINT('',(-0.6767,6.12423655037739E-13,-12.278617978381));
#64527=CARTESIAN_POINT('Ctrl Pts',(-0.676487528708653,-6.3808423934459E-5,
-10.178617978381));
#64528=CARTESIAN_POINT('Ctrl Pts',(-0.67646538092208,-0.00970439412085054,
-10.1781655736244));
#64529=CARTESIAN_POINT('Ctrl Pts',(-0.67359920801602,-0.13217276423391,
-10.1724176360363));
#64530=CARTESIAN_POINT('Ctrl Pts',(-0.604785322978651,-0.364132513572057,
-10.1613741656167));
#64531=CARTESIAN_POINT('Ctrl Pts',(-0.356816358110809,-0.607381249430332,
-10.1454875671223));
#64532=CARTESIAN_POINT('Ctrl Pts',(0.0908551895918876,-0.740698527863264,
-10.1243054357964));
#64533=CARTESIAN_POINT('Ctrl Pts',(0.543127711937286,-0.512033916001494,
-10.1031233044706));
#64534=CARTESIAN_POINT('Ctrl Pts',(0.69994058004243,-0.0729056387183608,
-10.0819411731447));
#64535=CARTESIAN_POINT('Ctrl Pts',(0.637628208112178,0.386897000631171,
-10.0607590418189));
#64536=CARTESIAN_POINT('Ctrl Pts',(0.142798839180318,0.788062006426542,
-10.0342813776615));
#64537=CARTESIAN_POINT('Ctrl Pts',(-0.525979911312534,0.564879541526795,
-10.0051358455718));
#64538=CARTESIAN_POINT('Ctrl Pts',(-0.67464464550151,0.169098391751588,
-9.98658137914492));
#64539=CARTESIAN_POINT('Ctrl Pts',(-0.67610244318158,-0.00026759660913226,
-9.978617978381));
#64540=CARTESIAN_POINT('Ctrl Pts',(-0.676977044559859,-0.000480244224215366,
-10.139182021619));
#64541=CARTESIAN_POINT('Ctrl Pts',(-0.677246035158063,-0.0505808665251606,
-10.1368224962279));
#64542=CARTESIAN_POINT('Ctrl Pts',(-0.648092810473929,-0.325072929503903,
-10.1238719051738));
#64543=CARTESIAN_POINT('Ctrl Pts',(-0.275804889831566,-0.751907505740747,
-10.1003302484568));
#64544=CARTESIAN_POINT('Ctrl Pts',(0.484188776139409,-0.637213310460941,
-10.0685570514681));
#64545=CARTESIAN_POINT('Ctrl Pts',(0.743655850199394,-0.0570496061916968,
-10.0420793873107));
#64546=CARTESIAN_POINT('Ctrl Pts',(0.591145954131398,0.383114078749073,
-10.0208972559849));
#64547=CARTESIAN_POINT('Ctrl Pts',(0.336618815106218,0.62052038455411,-10.0050106574905));
#64548=CARTESIAN_POINT('Ctrl Pts',(-0.000452053710239919,0.704435725401867,
-9.98912405899608));
#64549=CARTESIAN_POINT('Ctrl Pts',(-0.453902103296527,0.592335931104618,
-9.96794192767022));
#64550=CARTESIAN_POINT('Ctrl Pts',(-0.669133831075285,0.257202722580053,
-9.95129458187786));
#64551=CARTESIAN_POINT('Ctrl Pts',(-0.677514243797703,0.0165838220017427,
-9.93994276891696));
#64552=CARTESIAN_POINT('Ctrl Pts',(-0.677469765816856,0.000446699746677286,
-9.93918202161899));
#64553=CARTESIAN_POINT('Origin',(0.,0.,-12.278617978381));
#64554=CARTESIAN_POINT('',(-0.6767,6.63200977852672E-14,-10.378617978381));
#64555=CARTESIAN_POINT('',(-0.675326265922369,-7.01824404411022E-5,-10.339182021619));
#64556=CARTESIAN_POINT('',(-0.6767,6.12423655037739E-13,-12.278617978381));
#64557=CARTESIAN_POINT('Ctrl Pts',(-0.6767,6.63200977852672E-14,-10.378617978381));
#64558=CARTESIAN_POINT('Ctrl Pts',(-0.676700000000012,-0.122190759824434,
-10.3728703018844));
#64559=CARTESIAN_POINT('Ctrl Pts',(-0.642782324826098,-0.244335729754349,
-10.3671166238281));
#64560=CARTESIAN_POINT('Ctrl Pts',(-0.579718464473323,-0.349069322554551,
-10.3613659465517));
#64561=CARTESIAN_POINT('Ctrl Pts',(-0.478701924588147,-0.516833000439738,
-10.3521544343287));
#64562=CARTESIAN_POINT('Ctrl Pts',(-0.301547908367897,-0.636663758908016,
-10.3429429221058));
#64563=CARTESIAN_POINT('Ctrl Pts',(-0.108240294415161,-0.667987221932365,
-10.3337314098829));
#64564=CARTESIAN_POINT('Ctrl Pts',(0.0850673195375753,-0.699310684956715,
-10.32451989766));
#64565=CARTESIAN_POINT('Ctrl Pts',(0.290997402097898,-0.641554670250488,
-10.3153083854371));
#64566=CARTESIAN_POINT('Ctrl Pts',(0.439822575154538,-0.514275210742682,
-10.3060968732142));
#64567=CARTESIAN_POINT('Ctrl Pts',(0.588647748211179,-0.386995751234877,
-10.2968853609913));
#64568=CARTESIAN_POINT('Ctrl Pts',(0.677649438541112,-0.192517846946338,
-10.2876738487684));
#64569=CARTESIAN_POINT('Ctrl Pts',(0.676691910573216,0.00330880110782365,
-10.2784623365455));
#64570=CARTESIAN_POINT('Ctrl Pts',(0.675734382605319,0.199135449161986,
-10.2692508243226));
#64571=CARTESIAN_POINT('Ctrl Pts',(0.584835127398669,0.392733696935367,
-10.2600393120997));
#64572=CARTESIAN_POINT('Ctrl Pts',(0.434772390943479,0.518551692768706,
-10.2508277998768));
#64573=CARTESIAN_POINT('Ctrl Pts',(0.28470965448829,0.644369688602045,-10.2416162876539));
#64574=CARTESIAN_POINT('Ctrl Pts',(0.0782246164433667,0.700109128872225,
-10.232404775431));
#64575=CARTESIAN_POINT('Ctrl Pts',(-0.114767438629307,0.666896787389524,
-10.2231932632081));
#64576=CARTESIAN_POINT('Ctrl Pts',(-0.307759493701982,0.633684445906823,
-10.2139817509851));
#64577=CARTESIAN_POINT('Ctrl Pts',(-0.483733200957191,0.51212700889491,
-10.2047702387622));
#64578=CARTESIAN_POINT('Ctrl Pts',(-0.583104331267889,0.343383501142131,
-10.1955587265393));
#64579=CARTESIAN_POINT('Ctrl Pts',(-0.644021628814161,0.239938985228529,
-10.1899118104866));
#64580=CARTESIAN_POINT('Ctrl Pts',(-0.676699999999986,0.119990517192851,
-10.1842621586486));
#64581=CARTESIAN_POINT('Ctrl Pts',(-0.6767,8.09105695617297E-14,-10.178617978381));
#64582=CARTESIAN_POINT('Ctrl Pts',(-0.675326265922369,-7.01824404411369E-5,
-10.339182021619));
#64583=CARTESIAN_POINT('Ctrl Pts',(-0.675452075247173,-0.116937975956912,
-10.3337022235388));
#64584=CARTESIAN_POINT('Ctrl Pts',(-0.591837088309436,-0.459635281089491,
-10.3176313597956));
#64585=CARTESIAN_POINT('Ctrl Pts',(-0.0434573418998398,-0.79911891067786,
-10.2909694303896));
#64586=CARTESIAN_POINT('Ctrl Pts',(0.529876458749172,-0.524890102369867,
-10.2644917662322));
#64587=CARTESIAN_POINT('Ctrl Pts',(0.698575844497316,-0.0906737332777898,
-10.2433096349064));
#64588=CARTESIAN_POINT('Ctrl Pts',(0.658263143903542,0.255043932899648,
-10.227423036412));
#64589=CARTESIAN_POINT('Ctrl Pts',(0.455673622452517,0.537207078672659,
-10.2115364379176));
#64590=CARTESIAN_POINT('Ctrl Pts',(0.0374900855372222,0.745307633223355,
-10.1903543065917));
#64591=CARTESIAN_POINT('Ctrl Pts',(-0.447291532886714,0.597575708356613,
-10.1691721752659));
#64592=CARTESIAN_POINT('Ctrl Pts',(-0.651478821048851,0.237033566356607,
-10.1503495693311));
#64593=CARTESIAN_POINT('Ctrl Pts',(-0.676642333858851,0.061861021690888,
-10.1421180290593));
#64594=CARTESIAN_POINT('Ctrl Pts',(-0.676977044559859,-0.000480244224215366,
-10.139182021619));
#64595=CARTESIAN_POINT('Origin',(0.,0.,-12.278617978381));
#64596=CARTESIAN_POINT('',(-0.6767,7.09625967803593E-14,-10.578617978381));
#64597=CARTESIAN_POINT('',(-0.677129451882474,0.000855468478137583,-10.539182021619));
#64598=CARTESIAN_POINT('',(-0.6767,6.12423655037739E-13,-12.278617978381));
#64599=CARTESIAN_POINT('Ctrl Pts',(-0.6767,9.01955675519137E-14,-10.578617978381));
#64600=CARTESIAN_POINT('Ctrl Pts',(-0.676700000000023,-0.16852564549507,
-10.5706907759225));
#64601=CARTESIAN_POINT('Ctrl Pts',(-0.610812984105749,-0.336600349346967,
-10.5627444616155));
#64602=CARTESIAN_POINT('Ctrl Pts',(-0.496045337245928,-0.460284600433876,
-10.5548077032327));
#64603=CARTESIAN_POINT('Ctrl Pts',(-0.362844409252623,-0.603834263372039,
-10.5455961910098));
#64604=CARTESIAN_POINT('Ctrl Pts',(-0.1649223581656,-0.684888676154772,
-10.5363846787869));
#64605=CARTESIAN_POINT('Ctrl Pts',(0.0307049360566569,-0.676003030245987,
-10.527173166564));
#64606=CARTESIAN_POINT('Ctrl Pts',(0.226332230278914,-0.667117384337202,
-10.5179616543411));
#64607=CARTESIAN_POINT('Ctrl Pts',(0.416091265164732,-0.568453992862703,
-10.5087501421182));
#64608=CARTESIAN_POINT('Ctrl Pts',(0.535730136324974,-0.41342001769777,
-10.4995386298953));
#64609=CARTESIAN_POINT('Ctrl Pts',(0.655369007485216,-0.258386042532837,
-10.4903271176724));
#64610=CARTESIAN_POINT('Ctrl Pts',(0.702702284694006,-0.049813472412212,
-10.4811156054494));
#64611=CARTESIAN_POINT('Ctrl Pts',(0.661703046210972,0.141675575294828,
-10.4719040932265));
#64612=CARTESIAN_POINT('Ctrl Pts',(0.620703807727938,0.333164623001869,
-10.4626925810036));
#64613=CARTESIAN_POINT('Ctrl Pts',(0.49212098217594,0.504072238721918,-10.4534810687807));
#64614=CARTESIAN_POINT('Ctrl Pts',(0.319492372213088,0.596529558444218,
-10.4442695565578));
#64615=CARTESIAN_POINT('Ctrl Pts',(0.146863762250237,0.688986878166518,
-10.4350580443349));
#64616=CARTESIAN_POINT('Ctrl Pts',(-0.0666572441116555,0.701304994104118,
-10.425846532112));
#64617=CARTESIAN_POINT('Ctrl Pts',(-0.248773002156532,0.629313024970901,
-10.4166350198891));
#64618=CARTESIAN_POINT('Ctrl Pts',(-0.430888760201408,0.557321055837685,
-10.4074235076662));
#64619=CARTESIAN_POINT('Ctrl Pts',(-0.578272581216982,0.402334071090911,
-10.3982119954433));
#64620=CARTESIAN_POINT('Ctrl Pts',(-0.641020695498184,0.21683025144805,
-10.3890004832204));
#64621=CARTESIAN_POINT('Ctrl Pts',(-0.664595637535239,0.147135060670931,
-10.3855396482739));
#64622=CARTESIAN_POINT('Ctrl Pts',(-0.676699999999993,0.0735360430443412,
-10.3820770074178));
#64623=CARTESIAN_POINT('Ctrl Pts',(-0.6767,6.63200977852672E-14,-10.378617978381));
#64624=CARTESIAN_POINT('Ctrl Pts',(-0.677129451882474,0.000855468478137604,
-10.539182021619));
#64625=CARTESIAN_POINT('Ctrl Pts',(-0.675347882449493,-0.181846972849585,
-10.5305819508497));
#64626=CARTESIAN_POINT('Ctrl Pts',(-0.504225925926224,-0.593140613922127,
-10.5113908144174));
#64627=CARTESIAN_POINT('Ctrl Pts',(0.0640780911147829,-0.743083225043802,
-10.4869041451538));
#64628=CARTESIAN_POINT('Ctrl Pts',(0.473750232264011,-0.521335452325531,
-10.4657220138279));
#64629=CARTESIAN_POINT('Ctrl Pts',(0.666825430939749,-0.231736097711846,
-10.4498354153335));
#64630=CARTESIAN_POINT('Ctrl Pts',(0.695072554279996,0.114472878279935,
-10.4339488168391));
#64631=CARTESIAN_POINT('Ctrl Pts',(0.511051301097596,0.5437973356877,-10.4127666855133));
#64632=CARTESIAN_POINT('Ctrl Pts',(0.0459205840941021,0.745021974552772,
-10.3915845541874));
#64633=CARTESIAN_POINT('Ctrl Pts',(-0.39187382810385,0.584522840096347,
-10.3704024228615));
#64634=CARTESIAN_POINT('Ctrl Pts',(-0.624243083129975,0.33091208544373,
-10.3547000896159));
#64635=CARTESIAN_POINT('Ctrl Pts',(-0.675208917597839,0.108937951749951,
-10.3442932892017));
#64636=CARTESIAN_POINT('Ctrl Pts',(-0.675326265922369,-7.01824404411369E-5,
-10.339182021619));
#64637=CARTESIAN_POINT('Origin',(0.,0.,-12.278617978381));
#64638=CARTESIAN_POINT('',(-0.676458265251918,-5.37981942149026E-5,-10.778617978381));
#64639=CARTESIAN_POINT('',(-0.677536220770138,-0.000773839678422261,-10.739182021619));
#64640=CARTESIAN_POINT('',(-0.6767,6.12423655037739E-13,-12.278617978381));
#64641=CARTESIAN_POINT('Ctrl Pts',(-0.675361946382602,-0.000297784530493374,
-10.778617978381));
#64642=CARTESIAN_POINT('Ctrl Pts',(-0.675700118216433,-0.0963995788455786,
-10.7741002883886));
#64643=CARTESIAN_POINT('Ctrl Pts',(-0.634006218158301,-0.304924171127997,
-10.7642870655646));
#64644=CARTESIAN_POINT('Ctrl Pts',(-0.423251854828125,-0.562218743134393,
-10.7491783099093));
#64645=CARTESIAN_POINT('Ctrl Pts',(0.0028831951113741,-0.745822169195642,
-10.7279961785834));
#64646=CARTESIAN_POINT('Ctrl Pts',(0.601706547663041,-0.528566424343903,
-10.7015185144261));
#64647=CARTESIAN_POINT('Ctrl Pts',(0.769006630385937,0.221604098315976,
-10.6697453174373));
#64648=CARTESIAN_POINT('Ctrl Pts',(0.321574591885842,0.672955022981378,
-10.64326765328));
#64649=CARTESIAN_POINT('Ctrl Pts',(-0.143965254934612,0.689567938489952,
-10.6220855219541));
#64650=CARTESIAN_POINT('Ctrl Pts',(-0.457226793531636,0.537867487033261,
-10.6061989234597));
#64651=CARTESIAN_POINT('Ctrl Pts',(-0.639545145736122,0.278781774607292,
-10.5917097422687));
#64652=CARTESIAN_POINT('Ctrl Pts',(-0.677073472553969,0.0825194861469949,
-10.5825160939091));
#64653=CARTESIAN_POINT('Ctrl Pts',(-0.677379594393192,-0.000411018920503776,
-10.578617978381));
#64654=CARTESIAN_POINT('Ctrl Pts',(-0.677536220770138,-0.000773839678422372,
-10.739182021619));
#64655=CARTESIAN_POINT('Ctrl Pts',(-0.677711236608313,-0.0247038387901337,
-10.7380527438235));
#64656=CARTESIAN_POINT('Ctrl Pts',(-0.665747438455249,-0.272785151399114,
-10.7263324003651));
#64657=CARTESIAN_POINT('Ctrl Pts',(-0.432196993595701,-0.60785231744993,
-10.7093165240753));
#64658=CARTESIAN_POINT('Ctrl Pts',(0.0236003080504614,-0.704040454719466,
-10.6881343927494));
#64659=CARTESIAN_POINT('Ctrl Pts',(0.358233295234271,-0.608298183883769,
-10.672247794255));
#64660=CARTESIAN_POINT('Ctrl Pts',(0.603882212681613,-0.36270672558111,
-10.6563611957606));
#64661=CARTESIAN_POINT('Ctrl Pts',(0.741547131220323,0.0836470372069074,
-10.6351790644348));
#64662=CARTESIAN_POINT('Ctrl Pts',(0.517292027842344,0.53812210560505,-10.6139969331089));
#64663=CARTESIAN_POINT('Ctrl Pts',(0.0797096438481298,0.699198412773276,
-10.5928148017831));
#64664=CARTESIAN_POINT('Ctrl Pts',(-0.380677283636059,0.641360917581681,
-10.5716326704572));
#64665=CARTESIAN_POINT('Ctrl Pts',(-0.654778622651578,0.30990463904442,
-10.5537550770692));
#64666=CARTESIAN_POINT('Ctrl Pts',(-0.677541901470257,0.0431527515463504,
-10.5411730165126));
#64667=CARTESIAN_POINT('Ctrl Pts',(-0.677129451882474,0.000855468478137604,
-10.539182021619));
#64668=CARTESIAN_POINT('Origin',(0.,0.,-12.278617978381));
#64669=CARTESIAN_POINT('',(-0.6767,8.02475947705433E-14,-10.978617978381));
#64670=CARTESIAN_POINT('',(-0.67542960639225,3.49951570662865E-5,-10.939182021619));
#64671=CARTESIAN_POINT('',(-0.6767,6.12423655037739E-13,-12.278617978381));
#64672=CARTESIAN_POINT('Ctrl Pts',(-0.6767,9.46723228492091E-14,-10.978617978381));
#64673=CARTESIAN_POINT('Ctrl Pts',(-0.676700000000009,-0.0658041958681062,
-10.9755226442452));
#64674=CARTESIAN_POINT('Ctrl Pts',(-0.667020980110906,-0.131688646825892,
-10.972423161636));
#64675=CARTESIAN_POINT('Ctrl Pts',(-0.64807015609023,-0.194751027687109,
-10.9693257532635));
#64676=CARTESIAN_POINT('Ctrl Pts',(-0.591711508438059,-0.382294877980198,
-10.9601142410406));
#64677=CARTESIAN_POINT('Ctrl Pts',(-0.449721734150075,-0.542238180858732,
-10.9509027288177));
#64678=CARTESIAN_POINT('Ctrl Pts',(-0.270178193059374,-0.620424559471312,
-10.9416912165948));
#64679=CARTESIAN_POINT('Ctrl Pts',(-0.0906346519686727,-0.698610938083892,
-10.9324797043719));
#64680=CARTESIAN_POINT('Ctrl Pts',(0.123182953619341,-0.693612170370124,
-10.923268192149));
#64681=CARTESIAN_POINT('Ctrl Pts',(0.298876551279699,-0.607120825779477,
-10.9140566799261));
#64682=CARTESIAN_POINT('Ctrl Pts',(0.474570148940057,-0.52062948118883,
-10.9048451677032));
#64683=CARTESIAN_POINT('Ctrl Pts',(0.608930362864581,-0.354225487690465,
-10.8956336554803));
#64684=CARTESIAN_POINT('Ctrl Pts',(0.656463182062029,-0.164252794792037,
-10.8864221432573));
#64685=CARTESIAN_POINT('Ctrl Pts',(0.703996001259478,0.0257198981063917,
-10.8772106310344));
#64686=CARTESIAN_POINT('Ctrl Pts',(0.663833148899857,0.235791079919573,
-10.8679991188115));
#64687=CARTESIAN_POINT('Ctrl Pts',(0.549573659945365,0.394831207345944,
-10.8587876065886));
#64688=CARTESIAN_POINT('Ctrl Pts',(0.435314170990874,0.553871334772315,
-10.8495760943657));
#64689=CARTESIAN_POINT('Ctrl Pts',(0.249045211078671,0.658975239130211,
-10.8403645821428));
#64690=CARTESIAN_POINT('Ctrl Pts',(0.0538369544966078,0.674555018015974,
-10.8311530699199));
#64691=CARTESIAN_POINT('Ctrl Pts',(-0.141371302085456,0.690134796901736,
-10.821941557697));
#64692=CARTESIAN_POINT('Ctrl Pts',(-0.341953007380628,0.615905856191741,
-10.8127300454741));
#64693=CARTESIAN_POINT('Ctrl Pts',(-0.479991729591128,0.47700191773631,
-10.8035185332512));
#64694=CARTESIAN_POINT('Ctrl Pts',(-0.604373796054446,0.351840233910857,
-10.7952183482945));
#64695=CARTESIAN_POINT('Ctrl Pts',(-0.67669999999998,0.17626379960763,-10.7869091724096));
#64696=CARTESIAN_POINT('Ctrl Pts',(-0.6767,7.56050957754512E-14,-10.778617978381));
#64697=CARTESIAN_POINT('Ctrl Pts',(-0.67542960639225,3.4995157066342E-5,
-10.939182021619));
#64698=CARTESIAN_POINT('Ctrl Pts',(-0.675726540320146,-0.0905086959147912,
-10.9349324711344));
#64699=CARTESIAN_POINT('Ctrl Pts',(-0.637546849478435,-0.293800002514061,
-10.9253873878184));
#64700=CARTESIAN_POINT('Ctrl Pts',(-0.437774356145965,-0.551890885522362,
-10.9105467716709));
#64701=CARTESIAN_POINT('Ctrl Pts',(-0.120741175465174,-0.695542481001687,
-10.8946601731765));
#64702=CARTESIAN_POINT('Ctrl Pts',(0.225474399042472,-0.667376348810361,
-10.8787735746821));
#64703=CARTESIAN_POINT('Ctrl Pts',(0.619349525511595,-0.416287328540213,
-10.8575914433563));
#64704=CARTESIAN_POINT('Ctrl Pts',(0.7426298818878,0.0752814793781906,-10.8364093120304));
#64705=CARTESIAN_POINT('Ctrl Pts',(0.513381745134516,0.481322377944037,
-10.8152271807046));
#64706=CARTESIAN_POINT('Ctrl Pts',(0.12503781439124,0.735271763261725,-10.7940450493787));
#64707=CARTESIAN_POINT('Ctrl Pts',(-0.475417762247048,0.628657006331378,
-10.7686966630169));
#64708=CARTESIAN_POINT('Ctrl Pts',(-0.676069829824612,0.199726494404265,
-10.7486438094865));
#64709=CARTESIAN_POINT('Ctrl Pts',(-0.677536220770138,-0.000773839678422372,
-10.739182021619));
#64710=CARTESIAN_POINT('Origin',(0.,0.,-12.278617978381));
#64711=CARTESIAN_POINT('',(-0.677468338356203,7.29499899796481E-5,-11.178617978381));
#64712=CARTESIAN_POINT('',(-0.676834075999803,0.000191052801950281,-11.139182021619));
#64713=CARTESIAN_POINT('',(-0.6767,6.12423655037739E-13,-12.278617978381));
#64714=CARTESIAN_POINT('Ctrl Pts',(-0.677468338356203,7.29499899795568E-5,
-11.178617978381));
#64715=CARTESIAN_POINT('Ctrl Pts',(-0.677463317556368,-0.00346603282166678,
-11.1784508086733));
#64716=CARTESIAN_POINT('Ctrl Pts',(-0.67522084717329,-0.23121412904218,
-11.1676925733027));
#64717=CARTESIAN_POINT('Ctrl Pts',(-0.424197719174421,-0.679330206520831,
-11.1463432722691));
#64718=CARTESIAN_POINT('Ctrl Pts',(0.343160473225332,-0.722994096502876,
-11.1145700752803));
#64719=CARTESIAN_POINT('Ctrl Pts',(0.716133365261885,-0.208402697353022,
-11.088092411123));
#64720=CARTESIAN_POINT('Ctrl Pts',(0.657170405500786,0.253686804061263,
-11.0669102797971));
#64721=CARTESIAN_POINT('Ctrl Pts',(0.456763012508479,0.538261390715488,
-11.0510236813027));
#64722=CARTESIAN_POINT('Ctrl Pts',(0.144077853390088,0.689544391419175,
-11.0351370828084));
#64723=CARTESIAN_POINT('Ctrl Pts',(-0.322724961404119,0.672857766501242,
-11.0139549514825));
#64724=CARTESIAN_POINT('Ctrl Pts',(-0.638930029937868,0.351628493840238,
-10.9951152500067));
#64725=CARTESIAN_POINT('Ctrl Pts',(-0.6769768490303,0.0634282862764284,
-10.9815710813624));
#64726=CARTESIAN_POINT('Ctrl Pts',(-0.67664771829584,0.000479233537379581,
-10.978617978381));
#64727=CARTESIAN_POINT('Ctrl Pts',(-0.676834075999803,0.000191052801950271,
-11.139182021619));
#64728=CARTESIAN_POINT('Ctrl Pts',(-0.676650335253473,-0.0439955398353917,
-11.1371077312768));
#64729=CARTESIAN_POINT('Ctrl Pts',(-0.660795208169657,-0.201066433598618,
-11.1297379081032));
#64730=CARTESIAN_POINT('Ctrl Pts',(-0.542288925423647,-0.451973998913277,
-11.117072552098));
#64731=CARTESIAN_POINT('Ctrl Pts',(-0.260173180138369,-0.654629522639962,
-11.1011859536036));
#64732=CARTESIAN_POINT('Ctrl Pts',(0.20257790968715,-0.718227794756728,
-11.0800038222778));
#64733=CARTESIAN_POINT('Ctrl Pts',(0.61475932399721,-0.423364401158974,
-11.0588216909519));
#64734=CARTESIAN_POINT('Ctrl Pts',(0.702880058995295,0.0345205795692396,
-11.0376395596261));
#64735=CARTESIAN_POINT('Ctrl Pts',(0.571282631286294,0.479473853373007,
-11.0164574283002));
#64736=CARTESIAN_POINT('Ctrl Pts',(0.0211398831226441,0.800616225032851,
-10.9899797641429));
#64737=CARTESIAN_POINT('Ctrl Pts',(-0.570966914673425,0.496146330447829,
-10.9624561176387));
#64738=CARTESIAN_POINT('Ctrl Pts',(-0.674986498111135,0.135151448844078,
-10.9455235367974));
#64739=CARTESIAN_POINT('Ctrl Pts',(-0.67542960639225,3.4995157066342E-5,
-10.939182021619));
#64740=CARTESIAN_POINT('Origin',(0.,0.,-12.278617978381));
#64741=CARTESIAN_POINT('',(-0.676225509870168,-0.000584572772009204,-11.378617978381));
#64742=CARTESIAN_POINT('',(-0.676899469727254,-2.06163719228738E-5,-11.339182021619));
#64743=CARTESIAN_POINT('',(-0.6767,6.12423655037739E-13,-12.278617978381));
#64744=CARTESIAN_POINT('Ctrl Pts',(-0.676225509870168,-0.000584572772009233,
-11.378617978381));
#64745=CARTESIAN_POINT('Ctrl Pts',(-0.676904850538366,-0.0704961224808199,
-11.3753305359842));
#64746=CARTESIAN_POINT('Ctrl Pts',(-0.635139734798044,-0.365010782622285,
-11.3614520279245));
#64747=CARTESIAN_POINT('Ctrl Pts',(-0.206478220428704,-0.773205223454543,
-11.3369824542018));
#64748=CARTESIAN_POINT('Ctrl Pts',(0.410920283938739,-0.622433291638274,
-11.3105047900445));
#64749=CARTESIAN_POINT('Ctrl Pts',(0.665114014783227,-0.232063101779371,
-11.2893226587187));
#64750=CARTESIAN_POINT('Ctrl Pts',(0.696585389017661,0.11457124582531,-11.2734360602242));
#64751=CARTESIAN_POINT('Ctrl Pts',(0.55619304910803,0.432295255177504,-11.2575494617299));
#64752=CARTESIAN_POINT('Ctrl Pts',(0.189598103717612,0.721762795994409,
-11.236367330404));
#64753=CARTESIAN_POINT('Ctrl Pts',(-0.315180024953703,0.676629880018334,
-11.2151851990782));
#64754=CARTESIAN_POINT('Ctrl Pts',(-0.620884112411212,0.329425838331515,
-11.19417023746));
#64755=CARTESIAN_POINT('Ctrl Pts',(-0.677622364376125,0.10864040037347,
-11.1837463415048));
#64756=CARTESIAN_POINT('Ctrl Pts',(-0.677468338356203,7.29499899795568E-5,
-11.178617978381));
#64757=CARTESIAN_POINT('Ctrl Pts',(-0.676899469727254,-2.06163719228681E-5,
-11.339182021619));
#64758=CARTESIAN_POINT('Ctrl Pts',(-0.676893857161047,-0.110082133649128,
-11.3339874585877));
#64759=CARTESIAN_POINT('Ctrl Pts',(-0.620592612576125,-0.332187875396714,
-11.323497362725));
#64760=CARTESIAN_POINT('Ctrl Pts',(-0.310543480858139,-0.67856592981927,
-11.3024162011993));
#64761=CARTESIAN_POINT('Ctrl Pts',(0.194497940172004,-0.720650396469946,
-11.2812340698734));
#64762=CARTESIAN_POINT('Ctrl Pts',(0.558075706772724,-0.428699840487657,
-11.2600519385476));
#64763=CARTESIAN_POINT('Ctrl Pts',(0.745814935827746,-0.00437062783121209,
-11.2388698072217));
#64764=CARTESIAN_POINT('Ctrl Pts',(0.534393477883215,0.596537379583458,
-11.2123921430644));
#64765=CARTESIAN_POINT('Ctrl Pts',(-0.21411444420791,0.771125527228726,
-11.1806189460756));
#64766=CARTESIAN_POINT('Ctrl Pts',(-0.634097054479883,0.362811161644489,
-11.1562155722605));
#64767=CARTESIAN_POINT('Ctrl Pts',(-0.677119413826939,0.0688100531245896,
-11.1424032641083));
#64768=CARTESIAN_POINT('Ctrl Pts',(-0.676834075999803,0.000191052801950271,
-11.139182021619));
#64769=CARTESIAN_POINT('Origin',(0.,0.,-12.278617978381));
#64770=CARTESIAN_POINT('',(-0.67577016846339,0.000469772489560586,-11.578617978381));
#64771=CARTESIAN_POINT('',(-0.6767,1.01008828037874E-13,-11.539182021619));
#64772=CARTESIAN_POINT('',(-0.6767,6.12423655037739E-13,-12.278617978381));
#64773=CARTESIAN_POINT('Ctrl Pts',(-0.67577016846339,0.000469772489560594,
-11.578617978381));
#64774=CARTESIAN_POINT('Ctrl Pts',(-0.675013010550184,-0.13640120609862,
-11.5722102632951));
#64775=CARTESIAN_POINT('Ctrl Pts',(-0.56814302722758,-0.500655806665067,
-11.5552114825463));
#64776=CARTESIAN_POINT('Ctrl Pts',(-0.0897337187244002,-0.740423380881239,
-11.532917168966));
#64777=CARTESIAN_POINT('Ctrl Pts',(0.356717037324203,-0.607439441065005,
-11.5117350376402));
#64778=CARTESIAN_POINT('Ctrl Pts',(0.605099039586646,-0.36361113891817,
-11.4958484391458));
#64779=CARTESIAN_POINT('Ctrl Pts',(0.703772576709861,-0.0305614200295496,
-11.4799618406514));
#64780=CARTESIAN_POINT('Ctrl Pts',(0.611744859212238,0.427384163050785,
-11.4587797093255));
#64781=CARTESIAN_POINT('Ctrl Pts',(0.197790656500237,0.719753643173289,
-11.4375975779997));
#64782=CARTESIAN_POINT('Ctrl Pts',(-0.263619000263347,0.652485296666156,
-11.4164154466738));
#64783=CARTESIAN_POINT('Ctrl Pts',(-0.58209335344289,0.423941526590339,
-11.3985207577448));
#64784=CARTESIAN_POINT('Ctrl Pts',(-0.674716236790673,0.154736056274489,
-11.3859216016471));
#64785=CARTESIAN_POINT('Ctrl Pts',(-0.676225509870168,-0.000584572772009233,
-11.378617978381));
#64786=CARTESIAN_POINT('Ctrl Pts',(-0.676859540333324,-0.000246342469780166,
-11.539182021619));
#64787=CARTESIAN_POINT('Ctrl Pts',(-0.677143312751866,-0.0646519608093662,
-11.5361627187301));
#64788=CARTESIAN_POINT('Ctrl Pts',(-0.637526896910174,-0.354745471226495,
-11.5225523501783));
#64789=CARTESIAN_POINT('Ctrl Pts',(-0.318270223098515,-0.675181839024747,
-11.5036464487949));
#64790=CARTESIAN_POINT('Ctrl Pts',(0.147840292895422,-0.688022737605352,
-11.4824643174691));
#64791=CARTESIAN_POINT('Ctrl Pts',(0.565623962158729,-0.486136361723975,
-11.4612821861432));
#64792=CARTESIAN_POINT('Ctrl Pts',(0.793479716880401,0.108734401743206,
-11.4348045219859));
#64793=CARTESIAN_POINT('Ctrl Pts',(0.335993916742615,0.726352298131389,
-11.4030313249971));
#64794=CARTESIAN_POINT('Ctrl Pts',(-0.298112918637422,0.683671975462962,
-11.3765536608398));
#64795=CARTESIAN_POINT('Ctrl Pts',(-0.615475022766798,0.342666648827597,
-11.3553715295139));
#64796=CARTESIAN_POINT('Ctrl Pts',(-0.67634254234158,0.116460459871167,
-11.3446794940508));
#64797=CARTESIAN_POINT('Ctrl Pts',(-0.67689957882203,0.00211871456710879,
-11.3392829914192));
#64798=CARTESIAN_POINT('Ctrl Pts',(-0.676899469727254,-2.06163719228681E-5,
-11.339182021619));
#64799=CARTESIAN_POINT('Origin',(0.,0.,-12.278617978381));
#64800=CARTESIAN_POINT('',(-0.677716351375759,0.000193615723412327,-11.778617978381));
#64801=CARTESIAN_POINT('',(-0.6767,9.60347966456048E-14,-11.739182021619));
#64802=CARTESIAN_POINT('',(-0.6767,6.12423655037739E-13,-12.278617978381));
#64803=CARTESIAN_POINT('Ctrl Pts',(-0.677716351375759,0.000193615723412331,
-11.778617978381));
#64804=CARTESIAN_POINT('Ctrl Pts',(-0.676288025918613,-0.201313555190218,
-11.769089990606));
#64805=CARTESIAN_POINT('Ctrl Pts',(-0.526186147067614,-0.515751982643562,
-11.7542664699996));
#64806=CARTESIAN_POINT('Ctrl Pts',(-0.121403177164881,-0.693866619017976,
-11.7341474165617));
#64807=CARTESIAN_POINT('Ctrl Pts',(0.225850498452994,-0.668875211131948,
-11.7182608180673));
#64808=CARTESIAN_POINT('Ctrl Pts',(0.516608588870761,-0.478872034799853,
-11.7023742195729));
#64809=CARTESIAN_POINT('Ctrl Pts',(0.742947756127913,-0.0702747149864332,
-11.681192088247));
#64810=CARTESIAN_POINT('Ctrl Pts',(0.616681960998304,0.420553527772077,
-11.6600099569212));
#64811=CARTESIAN_POINT('Ctrl Pts',(0.221462490922912,0.667971079462276,
-11.6388278255953));
#64812=CARTESIAN_POINT('Ctrl Pts',(-0.241001769318581,0.705818539717338,
-11.6176456942695));
#64813=CARTESIAN_POINT('Ctrl Pts',(-0.618508626704561,0.404758836325352,
-11.597575745198));
#64814=CARTESIAN_POINT('Ctrl Pts',(-0.676264487725508,0.0898275668955524,
-11.582801328958));
#64815=CARTESIAN_POINT('Ctrl Pts',(-0.67577016846339,0.000469772489560594,
-11.578617978381));
#64816=CARTESIAN_POINT('Ctrl Pts',(-0.6767,8.52162505866054E-14,-11.739182021619));
#64817=CARTESIAN_POINT('Ctrl Pts',(-0.676700000000021,-0.167912749481023,
-11.731283648902));
#64818=CARTESIAN_POINT('Ctrl Pts',(-0.611309698394134,-0.335389744095952,
-11.723366169419));
#64819=CARTESIAN_POINT('Ctrl Pts',(-0.497294271809351,-0.458934959689941,
-11.715458243319));
#64820=CARTESIAN_POINT('Ctrl Pts',(-0.364483913909809,-0.602846049542439,
-11.7062467310961));
#64821=CARTESIAN_POINT('Ctrl Pts',(-0.16678284882323,-0.684437991556829,
-11.6970352188731));
#64822=CARTESIAN_POINT('Ctrl Pts',(0.028867868763758,-0.676083971229195,
-11.6878237066502));
#64823=CARTESIAN_POINT('Ctrl Pts',(0.224518586350746,-0.667729950901561,
-11.6786121944273));
#64824=CARTESIAN_POINT('Ctrl Pts',(0.414545026094418,-0.56958257021113,
-11.6694006822044));
#64825=CARTESIAN_POINT('Ctrl Pts',(0.534604741032153,-0.414874271154461,
-11.6601891699815));
#64826=CARTESIAN_POINT('Ctrl Pts',(0.654664455969888,-0.260165972097792,
-11.6509776577586));
#64827=CARTESIAN_POINT('Ctrl Pts',(0.702564328368376,-0.0517227943196359,
-11.6417661455357));
#64828=CARTESIAN_POINT('Ctrl Pts',(0.662085588863346,0.139876956713662,
-11.6325546333128));
#64829=CARTESIAN_POINT('Ctrl Pts',(0.621606849358317,0.331476707746961,
-11.6233431210899));
#64830=CARTESIAN_POINT('Ctrl Pts',(0.493488918674505,0.502733100256395,
-11.614131608867));
#64831=CARTESIAN_POINT('Ctrl Pts',(0.321112187304428,0.595659175338184,
-11.6049200966441));
#64832=CARTESIAN_POINT('Ctrl Pts',(0.148735455934352,0.688585250419974,
-11.5957085844212));
#64833=CARTESIAN_POINT('Ctrl Pts',(-0.0647512891489894,0.701483537584085,
-11.5864970721983));
#64834=CARTESIAN_POINT('Ctrl Pts',(-0.24706200400731,0.629986711110554,
-11.5772855599754));
#64835=CARTESIAN_POINT('Ctrl Pts',(-0.42937271886563,0.558489884637023,
-11.5680740477525));
#64836=CARTESIAN_POINT('Ctrl Pts',(-0.577177153531771,0.403903969266088,
-11.5588625355295));
#64837=CARTESIAN_POINT('Ctrl Pts',(-0.640429119637554,0.218571344691539,
-11.5496510233066));
#64838=CARTESIAN_POINT('Ctrl Pts',(-0.664391342990392,0.148360377064131,
-11.5461613560774));
#64839=CARTESIAN_POINT('Ctrl Pts',(-0.676699999999989,0.0741494619493284,
-11.5426699049933));
#64840=CARTESIAN_POINT('Ctrl Pts',(-0.6767,1.0100878303629E-13,-11.539182021619));
#64841=CARTESIAN_POINT('Ctrl Pts',(-0.292633023485541,-0.00545700788497927,
1.));
#64842=CARTESIAN_POINT('Ctrl Pts',(-0.292633023485541,-0.00545700788497927,
0.96));
#64843=CARTESIAN_POINT('Ctrl Pts',(-0.335948136076331,-0.00545700788497927,
1.));
#64844=CARTESIAN_POINT('Ctrl Pts',(-0.335948136076331,-0.00545700788497927,
0.96));
#64845=CARTESIAN_POINT('Ctrl Pts',(-0.364426996931434,-0.0341063976287842,
1.));
#64846=CARTESIAN_POINT('Ctrl Pts',(-0.364426996931434,-0.0341063976287842,
0.96));
#64847=CARTESIAN_POINT('',(-0.292633023485541,-0.00545700788497927,1.));
#64848=CARTESIAN_POINT('',(-0.364426996931434,-0.0341063976287842,1.));
#64849=CARTESIAN_POINT('Ctrl Pts',(-0.292633023485541,-0.00545700788497927,
1.));
#64850=CARTESIAN_POINT('Ctrl Pts',(-0.335948136076331,-0.00545700788497927,
1.));
#64851=CARTESIAN_POINT('Ctrl Pts',(-0.364426996931434,-0.0341063976287842,
1.));
#64852=CARTESIAN_POINT('',(-0.292633023485541,-0.00545700788497927,0.96));
#64853=CARTESIAN_POINT('',(-0.292633023485541,-0.00545700788497927,1.));
#64854=CARTESIAN_POINT('',(-0.364426996931434,-0.0341063976287842,0.96));
#64855=CARTESIAN_POINT('Ctrl Pts',(-0.292633023485541,-0.00545700788497927,
0.96));
#64856=CARTESIAN_POINT('Ctrl Pts',(-0.335948136076331,-0.00545700788497927,
0.96));
#64857=CARTESIAN_POINT('Ctrl Pts',(-0.364426996931434,-0.0341063976287842,
0.96));
#64858=CARTESIAN_POINT('',(-0.364426996931434,-0.0341063976287842,1.));
#64859=CARTESIAN_POINT('Ctrl Pts',(-0.218792613968253,-0.034447455406189,
1.));
#64860=CARTESIAN_POINT('Ctrl Pts',(-0.218792613968253,-0.034447455406189,
0.96));
#64861=CARTESIAN_POINT('Ctrl Pts',(-0.248294677957892,-0.00545700788497927,
1.));
#64862=CARTESIAN_POINT('Ctrl Pts',(-0.248294677957892,-0.00545700788497927,
0.96));
#64863=CARTESIAN_POINT('Ctrl Pts',(-0.292633023485541,-0.00545700788497927,
1.));
#64864=CARTESIAN_POINT('Ctrl Pts',(-0.292633023485541,-0.00545700788497927,
0.96));
#64865=CARTESIAN_POINT('',(-0.218792613968253,-0.034447455406189,1.));
#64866=CARTESIAN_POINT('Ctrl Pts',(-0.218792613968253,-0.034447455406189,
1.));
#64867=CARTESIAN_POINT('Ctrl Pts',(-0.248294677957892,-0.00545700788497927,
1.));
#64868=CARTESIAN_POINT('Ctrl Pts',(-0.292633023485541,-0.00545700788497927,
1.));
#64869=CARTESIAN_POINT('',(-0.218792613968253,-0.034447455406189,0.96));
#64870=CARTESIAN_POINT('',(-0.218792613968253,-0.034447455406189,1.));
#64871=CARTESIAN_POINT('Ctrl Pts',(-0.218792613968253,-0.034447455406189,
0.96));
#64872=CARTESIAN_POINT('Ctrl Pts',(-0.248294677957892,-0.00545700788497927,
0.96));
#64873=CARTESIAN_POINT('Ctrl Pts',(-0.292633023485541,-0.00545700788497927,
0.96));
#64874=CARTESIAN_POINT('Ctrl Pts',(-0.189290579780936,-0.107776248455048,
1.));
#64875=CARTESIAN_POINT('Ctrl Pts',(-0.189290579780936,-0.107776248455048,
0.96));
#64876=CARTESIAN_POINT('Ctrl Pts',(-0.189290579780936,-0.0634379029273987,
1.));
#64877=CARTESIAN_POINT('Ctrl Pts',(-0.189290579780936,-0.0634379029273987,
0.96));
#64878=CARTESIAN_POINT('Ctrl Pts',(-0.218792613968253,-0.034447455406189,
1.));
#64879=CARTESIAN_POINT('Ctrl Pts',(-0.218792613968253,-0.034447455406189,
0.96));
#64880=CARTESIAN_POINT('',(-0.189290579780936,-0.107776248455048,1.));
#64881=CARTESIAN_POINT('Ctrl Pts',(-0.189290579780936,-0.107776248455048,
1.));
#64882=CARTESIAN_POINT('Ctrl Pts',(-0.189290579780936,-0.0634379029273987,
1.));
#64883=CARTESIAN_POINT('Ctrl Pts',(-0.218792613968253,-0.034447455406189,
1.));
#64884=CARTESIAN_POINT('',(-0.189290579780936,-0.107776248455048,0.96));
#64885=CARTESIAN_POINT('',(-0.189290579780936,-0.107776248455048,1.));
#64886=CARTESIAN_POINT('Ctrl Pts',(-0.189290579780936,-0.107776248455048,
0.96));
#64887=CARTESIAN_POINT('Ctrl Pts',(-0.189290579780936,-0.0634379029273987,
0.96));
#64888=CARTESIAN_POINT('Ctrl Pts',(-0.218792613968253,-0.034447455406189,
0.96));
#64889=CARTESIAN_POINT('Ctrl Pts',(-0.217939969524741,-0.179740750789642,
1.));
#64890=CARTESIAN_POINT('Ctrl Pts',(-0.217939969524741,-0.179740750789642,
0.96));
#64891=CARTESIAN_POINT('Ctrl Pts',(-0.189290579780936,-0.151432418823242,
1.));
#64892=CARTESIAN_POINT('Ctrl Pts',(-0.189290579780936,-0.151432418823242,
0.96));
#64893=CARTESIAN_POINT('Ctrl Pts',(-0.189290579780936,-0.107776248455048,
1.));
#64894=CARTESIAN_POINT('Ctrl Pts',(-0.189290579780936,-0.107776248455048,
0.96));
#64895=CARTESIAN_POINT('',(-0.217939969524741,-0.179740750789642,1.));
#64896=CARTESIAN_POINT('Ctrl Pts',(-0.217939969524741,-0.179740750789642,
1.));
#64897=CARTESIAN_POINT('Ctrl Pts',(-0.189290579780936,-0.151432418823242,
1.));
#64898=CARTESIAN_POINT('Ctrl Pts',(-0.189290579780936,-0.107776248455048,
1.));
#64899=CARTESIAN_POINT('',(-0.217939969524741,-0.179740750789642,0.96));
#64900=CARTESIAN_POINT('',(-0.217939969524741,-0.179740750789642,1.));
#64901=CARTESIAN_POINT('Ctrl Pts',(-0.217939969524741,-0.179740750789642,
0.96));
#64902=CARTESIAN_POINT('Ctrl Pts',(-0.189290579780936,-0.151432418823242,
0.96));
#64903=CARTESIAN_POINT('Ctrl Pts',(-0.189290579780936,-0.107776248455048,
0.96));
#64904=CARTESIAN_POINT('Ctrl Pts',(-0.290586617216468,-0.208049082756043,
1.));
#64905=CARTESIAN_POINT('Ctrl Pts',(-0.290586617216468,-0.208049082756043,
0.96));
#64906=CARTESIAN_POINT('Ctrl Pts',(-0.246589359268546,-0.208049082756043,
1.));
#64907=CARTESIAN_POINT('Ctrl Pts',(-0.246589359268546,-0.208049082756043,
0.96));
#64908=CARTESIAN_POINT('Ctrl Pts',(-0.217939969524741,-0.179740750789642,
1.));
#64909=CARTESIAN_POINT('Ctrl Pts',(-0.217939969524741,-0.179740750789642,
0.96));
#64910=CARTESIAN_POINT('',(-0.290586617216468,-0.208049082756043,1.));
#64911=CARTESIAN_POINT('Ctrl Pts',(-0.290586617216468,-0.208049082756043,
1.));
#64912=CARTESIAN_POINT('Ctrl Pts',(-0.246589359268546,-0.208049082756043,
1.));
#64913=CARTESIAN_POINT('Ctrl Pts',(-0.217939969524741,-0.179740750789642,
1.));
#64914=CARTESIAN_POINT('',(-0.290586617216468,-0.208049082756043,0.96));
#64915=CARTESIAN_POINT('',(-0.290586617216468,-0.208049082756043,1.));
#64916=CARTESIAN_POINT('Ctrl Pts',(-0.290586617216468,-0.208049082756043,
0.96));
#64917=CARTESIAN_POINT('Ctrl Pts',(-0.246589359268546,-0.208049082756043,
0.96));
#64918=CARTESIAN_POINT('Ctrl Pts',(-0.217939969524741,-0.179740750789642,
0.96));
#64919=CARTESIAN_POINT('Ctrl Pts',(-0.343451556190848,-0.194577062129974,
1.));
#64920=CARTESIAN_POINT('Ctrl Pts',(-0.343451556190848,-0.194577062129974,
0.96));
#64921=CARTESIAN_POINT('Ctrl Pts',(-0.318894949182868,-0.208049082756043,
1.));
#64922=CARTESIAN_POINT('Ctrl Pts',(-0.318894949182868,-0.208049082756043,
0.96));
#64923=CARTESIAN_POINT('Ctrl Pts',(-0.290586617216468,-0.208049082756043,
1.));
#64924=CARTESIAN_POINT('Ctrl Pts',(-0.290586617216468,-0.208049082756043,
0.96));
#64925=CARTESIAN_POINT('',(-0.343451556190848,-0.194577062129974,1.));
#64926=CARTESIAN_POINT('Ctrl Pts',(-0.343451556190848,-0.194577062129974,
1.));
#64927=CARTESIAN_POINT('Ctrl Pts',(-0.318894949182868,-0.208049082756043,
1.));
#64928=CARTESIAN_POINT('Ctrl Pts',(-0.290586617216468,-0.208049082756043,
1.));
#64929=CARTESIAN_POINT('',(-0.343451556190848,-0.194577062129974,0.96));
#64930=CARTESIAN_POINT('',(-0.343451556190848,-0.194577062129974,1.));
#64931=CARTESIAN_POINT('Ctrl Pts',(-0.343451556190848,-0.194577062129974,
0.96));
#64932=CARTESIAN_POINT('Ctrl Pts',(-0.318894949182868,-0.208049082756043,
0.96));
#64933=CARTESIAN_POINT('Ctrl Pts',(-0.290586617216468,-0.208049082756043,
0.96));
#64934=CARTESIAN_POINT('Ctrl Pts',(-0.380457010492682,-0.156548404693604,
1.));
#64935=CARTESIAN_POINT('Ctrl Pts',(-0.380457010492682,-0.156548404693604,
0.96));
#64936=CARTESIAN_POINT('Ctrl Pts',(-0.368008163198829,-0.181104981899261,
1.));
#64937=CARTESIAN_POINT('Ctrl Pts',(-0.368008163198829,-0.181104981899261,
0.96));
#64938=CARTESIAN_POINT('Ctrl Pts',(-0.343451556190848,-0.194577062129974,
1.));
#64939=CARTESIAN_POINT('Ctrl Pts',(-0.343451556190848,-0.194577062129974,
0.96));
#64940=CARTESIAN_POINT('',(-0.380457010492682,-0.156548404693604,1.));
#64941=CARTESIAN_POINT('Ctrl Pts',(-0.380457010492682,-0.156548404693604,
1.));
#64942=CARTESIAN_POINT('Ctrl Pts',(-0.368008163198829,-0.181104981899261,
1.));
#64943=CARTESIAN_POINT('Ctrl Pts',(-0.343451556190848,-0.194577062129974,
1.));
#64944=CARTESIAN_POINT('',(-0.380457010492682,-0.156548404693604,0.96));
#64945=CARTESIAN_POINT('',(-0.380457010492682,-0.156548404693604,1.));
#64946=CARTESIAN_POINT('Ctrl Pts',(-0.380457010492682,-0.156548404693604,
0.96));
#64947=CARTESIAN_POINT('Ctrl Pts',(-0.368008163198829,-0.181104981899261,
0.96));
#64948=CARTESIAN_POINT('Ctrl Pts',(-0.343451556190848,-0.194577062129974,
0.96));
#64949=CARTESIAN_POINT('Ctrl Pts',(-0.392905857786536,-0.105729842185974,
1.));
#64950=CARTESIAN_POINT('Ctrl Pts',(-0.392905857786536,-0.105729842185974,
0.96));
#64951=CARTESIAN_POINT('Ctrl Pts',(-0.392905857786536,-0.131991767883301,
1.));
#64952=CARTESIAN_POINT('Ctrl Pts',(-0.392905857786536,-0.131991767883301,
0.96));
#64953=CARTESIAN_POINT('Ctrl Pts',(-0.380457010492682,-0.156548404693604,
1.));
#64954=CARTESIAN_POINT('Ctrl Pts',(-0.380457010492682,-0.156548404693604,
0.96));
#64955=CARTESIAN_POINT('',(-0.392905857786536,-0.105729842185974,1.));
#64956=CARTESIAN_POINT('Ctrl Pts',(-0.392905857786536,-0.105729842185974,
1.));
#64957=CARTESIAN_POINT('Ctrl Pts',(-0.392905857786536,-0.131991767883301,
1.));
#64958=CARTESIAN_POINT('Ctrl Pts',(-0.380457010492682,-0.156548404693604,
1.));
#64959=CARTESIAN_POINT('',(-0.392905857786536,-0.105729842185974,0.96));
#64960=CARTESIAN_POINT('',(-0.392905857786536,-0.105729842185974,1.));
#64961=CARTESIAN_POINT('Ctrl Pts',(-0.392905857786536,-0.105729842185974,
0.96));
#64962=CARTESIAN_POINT('Ctrl Pts',(-0.392905857786536,-0.131991767883301,
0.96));
#64963=CARTESIAN_POINT('Ctrl Pts',(-0.380457010492682,-0.156548404693604,
0.96));
#64964=CARTESIAN_POINT('Ctrl Pts',(-0.364426996931434,-0.0341063976287842,
1.));
#64965=CARTESIAN_POINT('Ctrl Pts',(-0.364426996931434,-0.0341063976287842,
0.96));
#64966=CARTESIAN_POINT('Ctrl Pts',(-0.392905857786536,-0.0627557873725891,
1.));
#64967=CARTESIAN_POINT('Ctrl Pts',(-0.392905857786536,-0.0627557873725891,
0.96));
#64968=CARTESIAN_POINT('Ctrl Pts',(-0.392905857786536,-0.105729842185974,
1.));
#64969=CARTESIAN_POINT('Ctrl Pts',(-0.392905857786536,-0.105729842185974,
0.96));
#64970=CARTESIAN_POINT('Ctrl Pts',(-0.364426996931434,-0.0341063976287842,
1.));
#64971=CARTESIAN_POINT('Ctrl Pts',(-0.392905857786536,-0.0627557873725891,
1.));
#64972=CARTESIAN_POINT('Ctrl Pts',(-0.392905857786536,-0.105729842185974,
1.));
#64973=CARTESIAN_POINT('Ctrl Pts',(-0.364426996931434,-0.0341063976287842,
0.96));
#64974=CARTESIAN_POINT('Ctrl Pts',(-0.392905857786536,-0.0627557873725891,
0.96));
#64975=CARTESIAN_POINT('Ctrl Pts',(-0.392905857786536,-0.105729842185974,
0.96));
#64976=CARTESIAN_POINT('Ctrl Pts',(-0.291609820351005,0.201568937301636,
1.));
#64977=CARTESIAN_POINT('Ctrl Pts',(-0.291609820351005,0.201568937301636,
0.96));
#64978=CARTESIAN_POINT('Ctrl Pts',(-0.32673942707479,0.201568937301636,
1.));
#64979=CARTESIAN_POINT('Ctrl Pts',(-0.32673942707479,0.201568937301636,
0.96));
#64980=CARTESIAN_POINT('Ctrl Pts',(-0.349931773170829,0.179058706760406,
1.));
#64981=CARTESIAN_POINT('Ctrl Pts',(-0.349931773170829,0.179058706760406,
0.96));
#64982=CARTESIAN_POINT('',(-0.291609820351005,0.201568937301636,1.));
#64983=CARTESIAN_POINT('',(-0.349931773170829,0.179058706760406,1.));
#64984=CARTESIAN_POINT('Ctrl Pts',(-0.291609820351005,0.201568937301636,
1.));
#64985=CARTESIAN_POINT('Ctrl Pts',(-0.32673942707479,0.201568937301636,
1.));
#64986=CARTESIAN_POINT('Ctrl Pts',(-0.349931773170829,0.179058706760406,
1.));
#64987=CARTESIAN_POINT('',(-0.291609820351005,0.201568937301636,0.96));
#64988=CARTESIAN_POINT('',(-0.291609820351005,0.201568937301636,1.));
#64989=CARTESIAN_POINT('',(-0.349931773170829,0.179058706760406,0.96));
#64990=CARTESIAN_POINT('Ctrl Pts',(-0.291609820351005,0.201568937301636,
0.96));
#64991=CARTESIAN_POINT('Ctrl Pts',(-0.32673942707479,0.201568937301636,
0.96));
#64992=CARTESIAN_POINT('Ctrl Pts',(-0.349931773170829,0.179058706760406,
0.96));
#64993=CARTESIAN_POINT('',(-0.349931773170829,0.179058706760406,1.));
#64994=CARTESIAN_POINT('Ctrl Pts',(-0.23345836661756,0.178547120094299,
1.));
#64995=CARTESIAN_POINT('Ctrl Pts',(-0.23345836661756,0.178547120094299,
0.96));
#64996=CARTESIAN_POINT('Ctrl Pts',(-0.256821271404624,0.201568937301636,
1.));
#64997=CARTESIAN_POINT('Ctrl Pts',(-0.256821271404624,0.201568937301636,
0.96));
#64998=CARTESIAN_POINT('Ctrl Pts',(-0.291609820351005,0.201568937301636,
1.));
#64999=CARTESIAN_POINT('Ctrl Pts',(-0.291609820351005,0.201568937301636,
0.96));
#65000=CARTESIAN_POINT('',(-0.23345836661756,0.178547120094299,1.));
#65001=CARTESIAN_POINT('Ctrl Pts',(-0.23345836661756,0.178547120094299,
1.));
#65002=CARTESIAN_POINT('Ctrl Pts',(-0.256821271404624,0.201568937301636,
1.));
#65003=CARTESIAN_POINT('Ctrl Pts',(-0.291609820351005,0.201568937301636,
1.));
#65004=CARTESIAN_POINT('',(-0.23345836661756,0.178547120094299,0.96));
#65005=CARTESIAN_POINT('',(-0.23345836661756,0.178547120094299,1.));
#65006=CARTESIAN_POINT('Ctrl Pts',(-0.23345836661756,0.178547120094299,
0.96));
#65007=CARTESIAN_POINT('Ctrl Pts',(-0.256821271404624,0.201568937301636,
0.96));
#65008=CARTESIAN_POINT('Ctrl Pts',(-0.291609820351005,0.201568937301636,
0.96));
#65009=CARTESIAN_POINT('Ctrl Pts',(-0.210095491632819,0.121759927272797,
1.));
#65010=CARTESIAN_POINT('Ctrl Pts',(-0.210095491632819,0.121759927272797,
0.96));
#65011=CARTESIAN_POINT('Ctrl Pts',(-0.210095491632819,0.15552527308464,
1.));
#65012=CARTESIAN_POINT('Ctrl Pts',(-0.210095491632819,0.15552527308464,
0.96));
#65013=CARTESIAN_POINT('Ctrl Pts',(-0.23345836661756,0.178547120094299,
1.));
#65014=CARTESIAN_POINT('Ctrl Pts',(-0.23345836661756,0.178547120094299,
0.96));
#65015=CARTESIAN_POINT('',(-0.210095491632819,0.121759927272797,1.));
#65016=CARTESIAN_POINT('Ctrl Pts',(-0.210095491632819,0.121759927272797,
1.));
#65017=CARTESIAN_POINT('Ctrl Pts',(-0.210095491632819,0.15552527308464,
1.));
#65018=CARTESIAN_POINT('Ctrl Pts',(-0.23345836661756,0.178547120094299,
1.));
#65019=CARTESIAN_POINT('',(-0.210095491632819,0.121759927272797,0.96));
#65020=CARTESIAN_POINT('',(-0.210095491632819,0.121759927272797,1.));
#65021=CARTESIAN_POINT('Ctrl Pts',(-0.210095491632819,0.121759927272797,
0.96));
#65022=CARTESIAN_POINT('Ctrl Pts',(-0.210095491632819,0.15552527308464,
0.96));
#65023=CARTESIAN_POINT('Ctrl Pts',(-0.23345836661756,0.178547120094299,
0.96));
#65024=CARTESIAN_POINT('Ctrl Pts',(-0.232776251062751,0.0670191407203674,
1.));
#65025=CARTESIAN_POINT('Ctrl Pts',(-0.232776251062751,0.0670191407203674,
0.96));
#65026=CARTESIAN_POINT('Ctrl Pts',(-0.210095491632819,0.0893588423728943,
1.));
#65027=CARTESIAN_POINT('Ctrl Pts',(-0.210095491632819,0.0893588423728943,
0.96));
#65028=CARTESIAN_POINT('Ctrl Pts',(-0.210095491632819,0.121759927272797,
1.));
#65029=CARTESIAN_POINT('Ctrl Pts',(-0.210095491632819,0.121759927272797,
0.96));
#65030=CARTESIAN_POINT('',(-0.232776251062751,0.0670191407203674,1.));
#65031=CARTESIAN_POINT('Ctrl Pts',(-0.232776251062751,0.0670191407203674,
1.));
#65032=CARTESIAN_POINT('Ctrl Pts',(-0.210095491632819,0.0893588423728943,
1.));
#65033=CARTESIAN_POINT('Ctrl Pts',(-0.210095491632819,0.121759927272797,
1.));
#65034=CARTESIAN_POINT('',(-0.232776251062751,0.0670191407203674,0.96));
#65035=CARTESIAN_POINT('',(-0.232776251062751,0.0670191407203674,1.));
#65036=CARTESIAN_POINT('Ctrl Pts',(-0.232776251062751,0.0670191407203674,
0.96));
#65037=CARTESIAN_POINT('Ctrl Pts',(-0.210095491632819,0.0893588423728943,
0.96));
#65038=CARTESIAN_POINT('Ctrl Pts',(-0.210095491632819,0.121759927272797,
0.96));
#65039=CARTESIAN_POINT('Ctrl Pts',(-0.290927674993873,0.0446794390678406,
1.));
#65040=CARTESIAN_POINT('Ctrl Pts',(-0.290927674993873,0.0446794390678406,
0.96));
#65041=CARTESIAN_POINT('Ctrl Pts',(-0.255457010492682,0.0446794390678406,
1.));
#65042=CARTESIAN_POINT('Ctrl Pts',(-0.255457010492682,0.0446794390678406,
0.96));
#65043=CARTESIAN_POINT('Ctrl Pts',(-0.232776251062751,0.0670191407203674,
1.));
#65044=CARTESIAN_POINT('Ctrl Pts',(-0.232776251062751,0.0670191407203674,
0.96));
#65045=CARTESIAN_POINT('',(-0.290927674993873,0.0446794390678406,1.));
#65046=CARTESIAN_POINT('Ctrl Pts',(-0.290927674993873,0.0446794390678406,
1.));
#65047=CARTESIAN_POINT('Ctrl Pts',(-0.255457010492682,0.0446794390678406,
1.));
#65048=CARTESIAN_POINT('Ctrl Pts',(-0.232776251062751,0.0670191407203674,
1.));
#65049=CARTESIAN_POINT('',(-0.290927674993873,0.0446794390678406,0.96));
#65050=CARTESIAN_POINT('',(-0.290927674993873,0.0446794390678406,1.));
#65051=CARTESIAN_POINT('Ctrl Pts',(-0.290927674993873,0.0446794390678406,
0.96));
#65052=CARTESIAN_POINT('Ctrl Pts',(-0.255457010492682,0.0446794390678406,
0.96));
#65053=CARTESIAN_POINT('Ctrl Pts',(-0.232776251062751,0.0670191407203674,
0.96));
#65054=CARTESIAN_POINT('Ctrl Pts',(-0.350272860750556,0.0671896696090698,
1.));
#65055=CARTESIAN_POINT('Ctrl Pts',(-0.350272860750556,0.0671896696090698,
0.96));
#65056=CARTESIAN_POINT('Ctrl Pts',(-0.3274215426296,0.0446794390678406,
1.));
#65057=CARTESIAN_POINT('Ctrl Pts',(-0.3274215426296,0.0446794390678406,
0.96));
#65058=CARTESIAN_POINT('Ctrl Pts',(-0.290927674993873,0.0446794390678406,
1.));
#65059=CARTESIAN_POINT('Ctrl Pts',(-0.290927674993873,0.0446794390678406,
0.96));
#65060=CARTESIAN_POINT('',(-0.350272860750556,0.0671896696090698,1.));
#65061=CARTESIAN_POINT('Ctrl Pts',(-0.350272860750556,0.0671896696090698,
1.));
#65062=CARTESIAN_POINT('Ctrl Pts',(-0.3274215426296,0.0446794390678406,
1.));
#65063=CARTESIAN_POINT('Ctrl Pts',(-0.290927674993873,0.0446794390678406,
1.));
#65064=CARTESIAN_POINT('',(-0.350272860750556,0.0671896696090698,0.96));
#65065=CARTESIAN_POINT('',(-0.350272860750556,0.0671896696090698,1.));
#65066=CARTESIAN_POINT('Ctrl Pts',(-0.350272860750556,0.0671896696090698,
0.96));
#65067=CARTESIAN_POINT('Ctrl Pts',(-0.3274215426296,0.0446794390678406,
0.96));
#65068=CARTESIAN_POINT('Ctrl Pts',(-0.290927674993873,0.0446794390678406,
0.96));
#65069=CARTESIAN_POINT('Ctrl Pts',(-0.37312414906919,0.125170594453812,
1.));
#65070=CARTESIAN_POINT('Ctrl Pts',(-0.37312414906919,0.125170594453812,
0.96));
#65071=CARTESIAN_POINT('Ctrl Pts',(-0.37312414906919,0.0896999001502991,
1.));
#65072=CARTESIAN_POINT('Ctrl Pts',(-0.37312414906919,0.0896999001502991,
0.96));
#65073=CARTESIAN_POINT('Ctrl Pts',(-0.350272860750556,0.0671896696090698,
1.));
#65074=CARTESIAN_POINT('Ctrl Pts',(-0.350272860750556,0.0671896696090698,
0.96));
#65075=CARTESIAN_POINT('',(-0.37312414906919,0.125170594453812,1.));
#65076=CARTESIAN_POINT('Ctrl Pts',(-0.37312414906919,0.125170594453812,
1.));
#65077=CARTESIAN_POINT('Ctrl Pts',(-0.37312414906919,0.0896999001502991,
1.));
#65078=CARTESIAN_POINT('Ctrl Pts',(-0.350272860750556,0.0671896696090698,
1.));
#65079=CARTESIAN_POINT('',(-0.37312414906919,0.125170594453812,0.96));
#65080=CARTESIAN_POINT('',(-0.37312414906919,0.125170594453812,1.));
#65081=CARTESIAN_POINT('Ctrl Pts',(-0.37312414906919,0.125170594453812,
0.96));
#65082=CARTESIAN_POINT('Ctrl Pts',(-0.37312414906919,0.0896999001502991,
0.96));
#65083=CARTESIAN_POINT('Ctrl Pts',(-0.350272860750556,0.0671896696090698,
0.96));
#65084=CARTESIAN_POINT('Ctrl Pts',(-0.349931773170829,0.179058706760406,
1.));
#65085=CARTESIAN_POINT('Ctrl Pts',(-0.349931773170829,0.179058706760406,
0.96));
#65086=CARTESIAN_POINT('Ctrl Pts',(-0.37312414906919,0.156548476219177,
1.));
#65087=CARTESIAN_POINT('Ctrl Pts',(-0.37312414906919,0.156548476219177,
0.96));
#65088=CARTESIAN_POINT('Ctrl Pts',(-0.37312414906919,0.125170594453812,
1.));
#65089=CARTESIAN_POINT('Ctrl Pts',(-0.37312414906919,0.125170594453812,
0.96));
#65090=CARTESIAN_POINT('Ctrl Pts',(-0.349931773170829,0.179058706760406,
1.));
#65091=CARTESIAN_POINT('Ctrl Pts',(-0.37312414906919,0.156548476219177,
1.));
#65092=CARTESIAN_POINT('Ctrl Pts',(-0.37312414906919,0.125170594453812,
1.));
#65093=CARTESIAN_POINT('Ctrl Pts',(-0.349931773170829,0.179058706760406,
0.96));
#65094=CARTESIAN_POINT('Ctrl Pts',(-0.37312414906919,0.156548476219177,
0.96));
#65095=CARTESIAN_POINT('Ctrl Pts',(-0.37312414906919,0.125170594453812,
0.96));
#65096=CARTESIAN_POINT('Ctrl Pts',(-0.410641190037131,-0.214699828624725,
1.));
#65097=CARTESIAN_POINT('Ctrl Pts',(-0.410641190037131,-0.214699828624725,
0.96));
#65098=CARTESIAN_POINT('Ctrl Pts',(-0.456002723798156,-0.170873069763184,
1.));
#65099=CARTESIAN_POINT('Ctrl Pts',(-0.456002723798156,-0.170873069763184,
0.96));
#65100=CARTESIAN_POINT('Ctrl Pts',(-0.456002723798156,-0.105388784408569,
1.));
#65101=CARTESIAN_POINT('Ctrl Pts',(-0.456002723798156,-0.105388784408569,
0.96));
#65102=CARTESIAN_POINT('',(-0.410641190037131,-0.214699828624725,1.));
#65103=CARTESIAN_POINT('',(-0.456002723798156,-0.105388784408569,1.));
#65104=CARTESIAN_POINT('Ctrl Pts',(-0.410641190037131,-0.214699828624725,
1.));
#65105=CARTESIAN_POINT('Ctrl Pts',(-0.456002723798156,-0.170873069763184,
1.));
#65106=CARTESIAN_POINT('Ctrl Pts',(-0.456002723798156,-0.105388784408569,
1.));
#65107=CARTESIAN_POINT('',(-0.410641190037131,-0.214699828624725,0.96));
#65108=CARTESIAN_POINT('',(-0.410641190037131,-0.214699828624725,1.));
#65109=CARTESIAN_POINT('',(-0.456002723798156,-0.105388784408569,0.96));
#65110=CARTESIAN_POINT('Ctrl Pts',(-0.410641190037131,-0.214699828624725,
0.96));
#65111=CARTESIAN_POINT('Ctrl Pts',(-0.456002723798156,-0.170873069763184,
0.96));
#65112=CARTESIAN_POINT('Ctrl Pts',(-0.456002723798156,-0.105388784408569,
0.96));
#65113=CARTESIAN_POINT('',(-0.456002723798156,-0.105388784408569,1.));
#65114=CARTESIAN_POINT('Ctrl Pts',(-0.291268732771277,-0.258526587486267,
1.));
#65115=CARTESIAN_POINT('Ctrl Pts',(-0.291268732771277,-0.258526587486267,
0.96));
#65116=CARTESIAN_POINT('Ctrl Pts',(-0.365279641374946,-0.258526587486267,
1.));
#65117=CARTESIAN_POINT('Ctrl Pts',(-0.365279641374946,-0.258526587486267,
0.96));
#65118=CARTESIAN_POINT('Ctrl Pts',(-0.410641190037131,-0.214699828624725,
1.));
#65119=CARTESIAN_POINT('Ctrl Pts',(-0.410641190037131,-0.214699828624725,
0.96));
#65120=CARTESIAN_POINT('',(-0.291268732771277,-0.258526587486267,1.));
#65121=CARTESIAN_POINT('Ctrl Pts',(-0.291268732771277,-0.258526587486267,
1.));
#65122=CARTESIAN_POINT('Ctrl Pts',(-0.365279641374946,-0.258526587486267,
1.));
#65123=CARTESIAN_POINT('Ctrl Pts',(-0.410641190037131,-0.214699828624725,
1.));
#65124=CARTESIAN_POINT('',(-0.291268732771277,-0.258526587486267,0.96));
#65125=CARTESIAN_POINT('',(-0.291268732771277,-0.258526587486267,1.));
#65126=CARTESIAN_POINT('Ctrl Pts',(-0.291268732771277,-0.258526587486267,
0.96));
#65127=CARTESIAN_POINT('Ctrl Pts',(-0.365279641374946,-0.258526587486267,
0.96));
#65128=CARTESIAN_POINT('Ctrl Pts',(-0.410641190037131,-0.214699828624725,
0.96));
#65129=CARTESIAN_POINT('Ctrl Pts',(-0.171896305307746,-0.214870357513428,
1.));
#65130=CARTESIAN_POINT('Ctrl Pts',(-0.171896305307746,-0.214870357513428,
0.96));
#65131=CARTESIAN_POINT('Ctrl Pts',(-0.217257824167609,-0.258526587486267,
1.));
#65132=CARTESIAN_POINT('Ctrl Pts',(-0.217257824167609,-0.258526587486267,
0.96));
#65133=CARTESIAN_POINT('Ctrl Pts',(-0.291268732771277,-0.258526587486267,
1.));
#65134=CARTESIAN_POINT('Ctrl Pts',(-0.291268732771277,-0.258526587486267,
0.96));
#65135=CARTESIAN_POINT('',(-0.171896305307746,-0.214870357513428,1.));
#65136=CARTESIAN_POINT('Ctrl Pts',(-0.171896305307746,-0.214870357513428,
1.));
#65137=CARTESIAN_POINT('Ctrl Pts',(-0.217257824167609,-0.258526587486267,
1.));
#65138=CARTESIAN_POINT('Ctrl Pts',(-0.291268732771277,-0.258526587486267,
1.));
#65139=CARTESIAN_POINT('',(-0.171896305307746,-0.214870357513428,0.96));
#65140=CARTESIAN_POINT('',(-0.171896305307746,-0.214870357513428,1.));
#65141=CARTESIAN_POINT('Ctrl Pts',(-0.171896305307746,-0.214870357513428,
0.96));
#65142=CARTESIAN_POINT('Ctrl Pts',(-0.217257824167609,-0.258526587486267,
0.96));
#65143=CARTESIAN_POINT('Ctrl Pts',(-0.291268732771277,-0.258526587486267,
0.96));
#65144=CARTESIAN_POINT('Ctrl Pts',(-0.126534726843238,-0.107094132900238,
1.));
#65145=CARTESIAN_POINT('Ctrl Pts',(-0.126534726843238,-0.107094132900238,
0.96));
#65146=CARTESIAN_POINT('Ctrl Pts',(-0.126534726843238,-0.171214127540588,
1.));
#65147=CARTESIAN_POINT('Ctrl Pts',(-0.126534726843238,-0.171214127540588,
0.96));
#65148=CARTESIAN_POINT('Ctrl Pts',(-0.171896305307746,-0.214870357513428,
1.));
#65149=CARTESIAN_POINT('Ctrl Pts',(-0.171896305307746,-0.214870357513428,
0.96));
#65150=CARTESIAN_POINT('',(-0.126534726843238,-0.107094132900238,1.));
#65151=CARTESIAN_POINT('Ctrl Pts',(-0.126534726843238,-0.107094132900238,
1.));
#65152=CARTESIAN_POINT('Ctrl Pts',(-0.126534726843238,-0.171214127540588,
1.));
#65153=CARTESIAN_POINT('Ctrl Pts',(-0.171896305307746,-0.214870357513428,
1.));
#65154=CARTESIAN_POINT('',(-0.126534726843238,-0.107094132900238,0.96));
#65155=CARTESIAN_POINT('',(-0.126534726843238,-0.107094132900238,1.));
#65156=CARTESIAN_POINT('Ctrl Pts',(-0.126534726843238,-0.107094132900238,
0.96));
#65157=CARTESIAN_POINT('Ctrl Pts',(-0.126534726843238,-0.171214127540588,
0.96));
#65158=CARTESIAN_POINT('Ctrl Pts',(-0.171896305307746,-0.214870357513428,
0.96));
#65159=CARTESIAN_POINT('Ctrl Pts',(-0.150579776987433,-0.0272850632667542,
1.));
#65160=CARTESIAN_POINT('Ctrl Pts',(-0.150579776987433,-0.0272850632667542,
0.96));
#65161=CARTESIAN_POINT('Ctrl Pts',(-0.126534726843238,-0.0607093811035156,
1.));
#65162=CARTESIAN_POINT('Ctrl Pts',(-0.126534726843238,-0.0607093811035156,
0.96));
#65163=CARTESIAN_POINT('Ctrl Pts',(-0.126534726843238,-0.107094132900238,
1.));
#65164=CARTESIAN_POINT('Ctrl Pts',(-0.126534726843238,-0.107094132900238,
0.96));
#65165=CARTESIAN_POINT('',(-0.150579776987433,-0.0272850632667542,1.));
#65166=CARTESIAN_POINT('Ctrl Pts',(-0.150579776987433,-0.0272850632667542,
1.));
#65167=CARTESIAN_POINT('Ctrl Pts',(-0.126534726843238,-0.0607093811035156,
1.));
#65168=CARTESIAN_POINT('Ctrl Pts',(-0.126534726843238,-0.107094132900238,
1.));
#65169=CARTESIAN_POINT('',(-0.150579776987433,-0.0272850632667542,0.96));
#65170=CARTESIAN_POINT('',(-0.150579776987433,-0.0272850632667542,1.));
#65171=CARTESIAN_POINT('Ctrl Pts',(-0.150579776987433,-0.0272850632667542,
0.96));
#65172=CARTESIAN_POINT('Ctrl Pts',(-0.126534726843238,-0.0607093811035156,
0.96));
#65173=CARTESIAN_POINT('Ctrl Pts',(-0.126534726843238,-0.107094132900238,
0.96));
#65174=CARTESIAN_POINT('Ctrl Pts',(-0.220668461546302,0.021146035194397,
1.));
#65175=CARTESIAN_POINT('Ctrl Pts',(-0.220668461546302,0.021146035194397,
0.96));
#65176=CARTESIAN_POINT('Ctrl Pts',(-0.174624797329307,0.00613919496536253,
1.));
#65177=CARTESIAN_POINT('Ctrl Pts',(-0.174624797329307,0.00613919496536253,
0.96));
#65178=CARTESIAN_POINT('Ctrl Pts',(-0.150579776987433,-0.0272850632667542,
1.));
#65179=CARTESIAN_POINT('Ctrl Pts',(-0.150579776987433,-0.0272850632667542,
0.96));
#65180=CARTESIAN_POINT('',(-0.220668461546302,0.021146035194397,1.));
#65181=CARTESIAN_POINT('Ctrl Pts',(-0.220668461546302,0.021146035194397,
1.));
#65182=CARTESIAN_POINT('Ctrl Pts',(-0.174624797329307,0.00613919496536253,
1.));
#65183=CARTESIAN_POINT('Ctrl Pts',(-0.150579776987433,-0.0272850632667542,
1.));
#65184=CARTESIAN_POINT('',(-0.220668461546302,0.021146035194397,0.96));
#65185=CARTESIAN_POINT('',(-0.220668461546302,0.021146035194397,1.));
#65186=CARTESIAN_POINT('Ctrl Pts',(-0.220668461546302,0.021146035194397,
0.96));
#65187=CARTESIAN_POINT('Ctrl Pts',(-0.174624797329307,0.00613919496536253,
0.96));
#65188=CARTESIAN_POINT('Ctrl Pts',(-0.150579776987433,-0.0272850632667542,
0.96));
#65189=CARTESIAN_POINT('Ctrl Pts',(-0.165245559439063,0.0608799815177917,
1.));
#65190=CARTESIAN_POINT('Ctrl Pts',(-0.165245559439063,0.0608799815177917,
0.96));
#65191=CARTESIAN_POINT('Ctrl Pts',(-0.183492478355765,0.0351296424865722,
1.));
#65192=CARTESIAN_POINT('Ctrl Pts',(-0.183492478355765,0.0351296424865722,
0.96));
#65193=CARTESIAN_POINT('Ctrl Pts',(-0.220668461546302,0.021146035194397,
1.));
#65194=CARTESIAN_POINT('Ctrl Pts',(-0.220668461546302,0.021146035194397,
0.96));
#65195=CARTESIAN_POINT('',(-0.165245559439063,0.0608799815177917,1.));
#65196=CARTESIAN_POINT('Ctrl Pts',(-0.165245559439063,0.0608799815177917,
1.));
#65197=CARTESIAN_POINT('Ctrl Pts',(-0.183492478355765,0.0351296424865722,
1.));
#65198=CARTESIAN_POINT('Ctrl Pts',(-0.220668461546302,0.021146035194397,
1.));
#65199=CARTESIAN_POINT('',(-0.165245559439063,0.0608799815177917,0.96));
#65200=CARTESIAN_POINT('',(-0.165245559439063,0.0608799815177917,1.));
#65201=CARTESIAN_POINT('Ctrl Pts',(-0.165245559439063,0.0608799815177917,
0.96));
#65202=CARTESIAN_POINT('Ctrl Pts',(-0.183492478355765,0.0351296424865722,
0.96));
#65203=CARTESIAN_POINT('Ctrl Pts',(-0.220668461546302,0.021146035194397,
0.96));
#65204=CARTESIAN_POINT('Ctrl Pts',(-0.146998610720038,0.121418869495392,
1.));
#65205=CARTESIAN_POINT('Ctrl Pts',(-0.146998610720038,0.121418869495392,
0.96));
#65206=CARTESIAN_POINT('Ctrl Pts',(-0.146998610720038,0.0866303205490112,
1.));
#65207=CARTESIAN_POINT('Ctrl Pts',(-0.146998610720038,0.0866303205490112,
0.96));
#65208=CARTESIAN_POINT('Ctrl Pts',(-0.165245559439063,0.0608799815177917,
1.));
#65209=CARTESIAN_POINT('Ctrl Pts',(-0.165245559439063,0.0608799815177917,
0.96));
#65210=CARTESIAN_POINT('',(-0.146998610720038,0.121418869495392,1.));
#65211=CARTESIAN_POINT('Ctrl Pts',(-0.146998610720038,0.121418869495392,
1.));
#65212=CARTESIAN_POINT('Ctrl Pts',(-0.146998610720038,0.0866303205490112,
1.));
#65213=CARTESIAN_POINT('Ctrl Pts',(-0.165245559439063,0.0608799815177917,
1.));
#65214=CARTESIAN_POINT('',(-0.146998610720038,0.121418869495392,0.96));
#65215=CARTESIAN_POINT('',(-0.146998610720038,0.121418869495392,1.));
#65216=CARTESIAN_POINT('Ctrl Pts',(-0.146998610720038,0.121418869495392,
0.96));
#65217=CARTESIAN_POINT('Ctrl Pts',(-0.146998610720038,0.0866303205490112,
0.96));
#65218=CARTESIAN_POINT('Ctrl Pts',(-0.165245559439063,0.0608799815177917,
0.96));
#65219=CARTESIAN_POINT('Ctrl Pts',(-0.186903115734458,0.214017784595489,
1.));
#65220=CARTESIAN_POINT('Ctrl Pts',(-0.186903115734458,0.214017784595489,
0.96));
#65221=CARTESIAN_POINT('Ctrl Pts',(-0.146998610720038,0.175989127159119,
1.));
#65222=CARTESIAN_POINT('Ctrl Pts',(-0.146998610720038,0.175989127159119,
0.96));
#65223=CARTESIAN_POINT('Ctrl Pts',(-0.146998610720038,0.121418869495392,
1.));
#65224=CARTESIAN_POINT('Ctrl Pts',(-0.146998610720038,0.121418869495392,
0.96));
#65225=CARTESIAN_POINT('',(-0.186903115734458,0.214017784595489,1.));
#65226=CARTESIAN_POINT('Ctrl Pts',(-0.186903115734458,0.214017784595489,
1.));
#65227=CARTESIAN_POINT('Ctrl Pts',(-0.146998610720038,0.175989127159119,
1.));
#65228=CARTESIAN_POINT('Ctrl Pts',(-0.146998610720038,0.121418869495392,
1.));
#65229=CARTESIAN_POINT('',(-0.186903115734458,0.214017784595489,0.96));
#65230=CARTESIAN_POINT('',(-0.186903115734458,0.214017784595489,1.));
#65231=CARTESIAN_POINT('Ctrl Pts',(-0.186903115734458,0.214017784595489,
0.96));
#65232=CARTESIAN_POINT('Ctrl Pts',(-0.146998610720038,0.175989127159119,
0.96));
#65233=CARTESIAN_POINT('Ctrl Pts',(-0.146998610720038,0.121418869495392,
0.96));
#65234=CARTESIAN_POINT('Ctrl Pts',(-0.292291965708137,0.252046382427216,
1.));
#65235=CARTESIAN_POINT('Ctrl Pts',(-0.292291965708137,0.252046382427216,
0.96));
#65236=CARTESIAN_POINT('Ctrl Pts',(-0.226807620748878,0.252046382427216,
1.));
#65237=CARTESIAN_POINT('Ctrl Pts',(-0.226807620748878,0.252046382427216,
0.96));
#65238=CARTESIAN_POINT('Ctrl Pts',(-0.186903115734458,0.214017784595489,
1.));
#65239=CARTESIAN_POINT('Ctrl Pts',(-0.186903115734458,0.214017784595489,
0.96));
#65240=CARTESIAN_POINT('',(-0.292291965708137,0.252046382427216,1.));
#65241=CARTESIAN_POINT('Ctrl Pts',(-0.292291965708137,0.252046382427216,
1.));
#65242=CARTESIAN_POINT('Ctrl Pts',(-0.226807620748878,0.252046382427216,
1.));
#65243=CARTESIAN_POINT('Ctrl Pts',(-0.186903115734458,0.214017784595489,
1.));
#65244=CARTESIAN_POINT('',(-0.292291965708137,0.252046382427216,0.96));
#65245=CARTESIAN_POINT('',(-0.292291965708137,0.252046382427216,1.));
#65246=CARTESIAN_POINT('Ctrl Pts',(-0.292291965708137,0.252046382427216,
0.96));
#65247=CARTESIAN_POINT('Ctrl Pts',(-0.226807620748878,0.252046382427216,
0.96));
#65248=CARTESIAN_POINT('Ctrl Pts',(-0.186903115734458,0.214017784595489,
0.96));
#65249=CARTESIAN_POINT('Ctrl Pts',(-0.396657552942634,0.214870429039001,
1.));
#65250=CARTESIAN_POINT('Ctrl Pts',(-0.396657552942634,0.214870429039001,
0.96));
#65251=CARTESIAN_POINT('Ctrl Pts',(-0.357435193285346,0.252046382427216,
1.));
#65252=CARTESIAN_POINT('Ctrl Pts',(-0.357435193285346,0.252046382427216,
0.96));
#65253=CARTESIAN_POINT('Ctrl Pts',(-0.292291965708137,0.252046382427216,
1.));
#65254=CARTESIAN_POINT('Ctrl Pts',(-0.292291965708137,0.252046382427216,
0.96));
#65255=CARTESIAN_POINT('',(-0.396657552942634,0.214870429039001,1.));
#65256=CARTESIAN_POINT('Ctrl Pts',(-0.396657552942634,0.214870429039001,
1.));
#65257=CARTESIAN_POINT('Ctrl Pts',(-0.357435193285346,0.252046382427216,
1.));
#65258=CARTESIAN_POINT('Ctrl Pts',(-0.292291965708137,0.252046382427216,
1.));
#65259=CARTESIAN_POINT('',(-0.396657552942634,0.214870429039001,0.96));
#65260=CARTESIAN_POINT('',(-0.396657552942634,0.214870429039001,1.));
#65261=CARTESIAN_POINT('Ctrl Pts',(-0.396657552942634,0.214870429039001,
0.96));
#65262=CARTESIAN_POINT('Ctrl Pts',(-0.357435193285346,0.252046382427216,
0.96));
#65263=CARTESIAN_POINT('Ctrl Pts',(-0.292291965708137,0.252046382427216,
0.96));
#65264=CARTESIAN_POINT('Ctrl Pts',(-0.435879942402244,0.123124188184738,
1.));
#65265=CARTESIAN_POINT('Ctrl Pts',(-0.435879942402244,0.123124188184738,
0.96));
#65266=CARTESIAN_POINT('Ctrl Pts',(-0.435879942402244,0.177694445848465,
1.));
#65267=CARTESIAN_POINT('Ctrl Pts',(-0.435879942402244,0.177694445848465,
0.96));
#65268=CARTESIAN_POINT('Ctrl Pts',(-0.396657552942634,0.214870429039001,
1.));
#65269=CARTESIAN_POINT('Ctrl Pts',(-0.396657552942634,0.214870429039001,
0.96));
#65270=CARTESIAN_POINT('',(-0.435879942402244,0.123124188184738,1.));
#65271=CARTESIAN_POINT('Ctrl Pts',(-0.435879942402244,0.123124188184738,
1.));
#65272=CARTESIAN_POINT('Ctrl Pts',(-0.435879942402244,0.177694445848465,
1.));
#65273=CARTESIAN_POINT('Ctrl Pts',(-0.396657552942634,0.214870429039001,
1.));
#65274=CARTESIAN_POINT('',(-0.435879942402244,0.123124188184738,0.96));
#65275=CARTESIAN_POINT('',(-0.435879942402244,0.123124188184738,1.));
#65276=CARTESIAN_POINT('Ctrl Pts',(-0.435879942402244,0.123124188184738,
0.96));
#65277=CARTESIAN_POINT('Ctrl Pts',(-0.435879942402244,0.177694445848465,
0.96));
#65278=CARTESIAN_POINT('Ctrl Pts',(-0.396657552942634,0.214870429039001,
0.96));
#65279=CARTESIAN_POINT('Ctrl Pts',(-0.417462464794517,0.0610505104064941,
1.));
#65280=CARTESIAN_POINT('Ctrl Pts',(-0.417462464794517,0.0610505104064941,
0.96));
#65281=CARTESIAN_POINT('Ctrl Pts',(-0.435879942402244,0.0869714081287384,
1.));
#65282=CARTESIAN_POINT('Ctrl Pts',(-0.435879942402244,0.0869714081287384,
0.96));
#65283=CARTESIAN_POINT('Ctrl Pts',(-0.435879942402244,0.123124188184738,
1.));
#65284=CARTESIAN_POINT('Ctrl Pts',(-0.435879942402244,0.123124188184738,
0.96));
#65285=CARTESIAN_POINT('',(-0.417462464794517,0.0610505104064941,1.));
#65286=CARTESIAN_POINT('Ctrl Pts',(-0.417462464794517,0.0610505104064941,
1.));
#65287=CARTESIAN_POINT('Ctrl Pts',(-0.435879942402244,0.0869714081287384,
1.));
#65288=CARTESIAN_POINT('Ctrl Pts',(-0.435879942402244,0.123124188184738,
1.));
#65289=CARTESIAN_POINT('',(-0.417462464794517,0.0610505104064941,0.96));
#65290=CARTESIAN_POINT('',(-0.417462464794517,0.0610505104064941,1.));
#65291=CARTESIAN_POINT('Ctrl Pts',(-0.417462464794517,0.0610505104064941,
0.96));
#65292=CARTESIAN_POINT('Ctrl Pts',(-0.435879942402244,0.0869714081287384,
0.96));
#65293=CARTESIAN_POINT('Ctrl Pts',(-0.435879942402244,0.123124188184738,
0.96));
#65294=CARTESIAN_POINT('Ctrl Pts',(-0.360845830664039,0.021146035194397,
1.));
#65295=CARTESIAN_POINT('Ctrl Pts',(-0.360845830664039,0.021146035194397,
0.96));
#65296=CARTESIAN_POINT('Ctrl Pts',(-0.399045016989112,0.0351296424865722,
1.));
#65297=CARTESIAN_POINT('Ctrl Pts',(-0.399045016989112,0.0351296424865722,
0.96));
#65298=CARTESIAN_POINT('Ctrl Pts',(-0.417462464794517,0.0610505104064941,
1.));
#65299=CARTESIAN_POINT('Ctrl Pts',(-0.417462464794517,0.0610505104064941,
0.96));
#65300=CARTESIAN_POINT('',(-0.360845830664039,0.021146035194397,1.));
#65301=CARTESIAN_POINT('Ctrl Pts',(-0.360845830664039,0.021146035194397,
1.));
#65302=CARTESIAN_POINT('Ctrl Pts',(-0.399045016989112,0.0351296424865722,
1.));
#65303=CARTESIAN_POINT('Ctrl Pts',(-0.417462464794517,0.0610505104064941,
1.));
#65304=CARTESIAN_POINT('',(-0.360845830664039,0.021146035194397,0.96));
#65305=CARTESIAN_POINT('',(-0.360845830664039,0.021146035194397,1.));
#65306=CARTESIAN_POINT('Ctrl Pts',(-0.360845830664039,0.021146035194397,
0.96));
#65307=CARTESIAN_POINT('Ctrl Pts',(-0.399045016989112,0.0351296424865722,
0.96));
#65308=CARTESIAN_POINT('Ctrl Pts',(-0.417462464794517,0.0610505104064941,
0.96));
#65309=CARTESIAN_POINT('Ctrl Pts',(-0.431275573000312,-0.0237038969993592,
1.));
#65310=CARTESIAN_POINT('Ctrl Pts',(-0.431275573000312,-0.0237038969993592,
0.96));
#65311=CARTESIAN_POINT('Ctrl Pts',(-0.406548422202468,0.00920877456665037,
1.));
#65312=CARTESIAN_POINT('Ctrl Pts',(-0.406548422202468,0.00920877456665037,
0.96));
#65313=CARTESIAN_POINT('Ctrl Pts',(-0.360845830664039,0.021146035194397,
1.));
#65314=CARTESIAN_POINT('Ctrl Pts',(-0.360845830664039,0.021146035194397,
0.96));
#65315=CARTESIAN_POINT('',(-0.431275573000312,-0.0237038969993592,1.));
#65316=CARTESIAN_POINT('Ctrl Pts',(-0.431275573000312,-0.0237038969993592,
1.));
#65317=CARTESIAN_POINT('Ctrl Pts',(-0.406548422202468,0.00920877456665037,
1.));
#65318=CARTESIAN_POINT('Ctrl Pts',(-0.360845830664039,0.021146035194397,
1.));
#65319=CARTESIAN_POINT('',(-0.431275573000312,-0.0237038969993592,0.96));
#65320=CARTESIAN_POINT('',(-0.431275573000312,-0.0237038969993592,1.));
#65321=CARTESIAN_POINT('Ctrl Pts',(-0.431275573000312,-0.0237038969993592,
0.96));
#65322=CARTESIAN_POINT('Ctrl Pts',(-0.406548422202468,0.00920877456665037,
0.96));
#65323=CARTESIAN_POINT('Ctrl Pts',(-0.360845830664039,0.021146035194397,
0.96));
#65324=CARTESIAN_POINT('Ctrl Pts',(-0.456002723798156,-0.105388784408569,
1.));
#65325=CARTESIAN_POINT('Ctrl Pts',(-0.456002723798156,-0.105388784408569,
0.96));
#65326=CARTESIAN_POINT('Ctrl Pts',(-0.456002723798156,-0.0566166281700134,
1.));
#65327=CARTESIAN_POINT('Ctrl Pts',(-0.456002723798156,-0.0566166281700134,
0.96));
#65328=CARTESIAN_POINT('Ctrl Pts',(-0.431275573000312,-0.0237038969993592,
1.));
#65329=CARTESIAN_POINT('Ctrl Pts',(-0.431275573000312,-0.0237038969993592,
0.96));
#65330=CARTESIAN_POINT('Ctrl Pts',(-0.456002723798156,-0.105388784408569,
1.));
#65331=CARTESIAN_POINT('Ctrl Pts',(-0.456002723798156,-0.0566166281700134,
1.));
#65332=CARTESIAN_POINT('Ctrl Pts',(-0.431275573000312,-0.0237038969993592,
1.));
#65333=CARTESIAN_POINT('Ctrl Pts',(-0.456002723798156,-0.105388784408569,
0.96));
#65334=CARTESIAN_POINT('Ctrl Pts',(-0.456002723798156,-0.0566166281700134,
0.96));
#65335=CARTESIAN_POINT('Ctrl Pts',(-0.431275573000312,-0.0237038969993592,
0.96));
#65336=CARTESIAN_POINT('Origin',(-0.291268725320697,-0.00324010252952578,
0.96));
#65337=CARTESIAN_POINT('Origin',(-0.0324011113494634,-0.180081808567047,
1.));
#65338=CARTESIAN_POINT('',(-0.0324011113494634,-0.180081808567047,1.));
#65339=CARTESIAN_POINT('',(0.0375170443207026,-0.180081808567047,1.));
#65340=CARTESIAN_POINT('',(-0.0162005556747317,-0.180081808567047,1.));
#65341=CARTESIAN_POINT('',(-0.0324011113494634,-0.180081808567047,0.96));
#65342=CARTESIAN_POINT('',(-0.0324011113494634,-0.180081808567047,1.));
#65343=CARTESIAN_POINT('',(0.0375170443207026,-0.180081808567047,0.96));
#65344=CARTESIAN_POINT('',(-0.0324011113494634,-0.180081808567047,0.96));
#65345=CARTESIAN_POINT('',(0.0375170443207026,-0.180081808567047,1.));
#65346=CARTESIAN_POINT('Origin',(-0.0324011113494634,-0.249999964237213,
1.));
#65347=CARTESIAN_POINT('',(-0.0324011113494634,-0.249999964237213,1.));
#65348=CARTESIAN_POINT('',(-0.0324011113494634,-0.124999982118607,1.));
#65349=CARTESIAN_POINT('',(-0.0324011113494634,-0.249999964237213,0.96));
#65350=CARTESIAN_POINT('',(-0.0324011113494634,-0.249999964237213,1.));
#65351=CARTESIAN_POINT('',(-0.0324011113494634,-0.249999964237213,0.96));
#65352=CARTESIAN_POINT('Origin',(0.0375170443207026,-0.249999964237213,
1.));
#65353=CARTESIAN_POINT('',(0.0375170443207026,-0.249999964237213,1.));
#65354=CARTESIAN_POINT('',(0.0187585221603513,-0.249999964237213,1.));
#65355=CARTESIAN_POINT('',(0.0375170443207026,-0.249999964237213,0.96));
#65356=CARTESIAN_POINT('',(0.0375170443207026,-0.249999964237213,1.));
#65357=CARTESIAN_POINT('',(0.0375170443207026,-0.249999964237213,0.96));
#65358=CARTESIAN_POINT('Origin',(0.0375170443207026,-0.180081808567047,
1.));
#65359=CARTESIAN_POINT('',(0.0375170443207026,-0.0900409042835236,1.));
#65360=CARTESIAN_POINT('',(0.0375170443207026,-0.180081808567047,0.96));
#65361=CARTESIAN_POINT('Origin',(0.00255796648561957,-0.21504088640213,
0.96));
#65362=CARTESIAN_POINT('Ctrl Pts',(0.289904567971826,-0.00545700788497927,
1.));
#65363=CARTESIAN_POINT('Ctrl Pts',(0.289904567971826,-0.00545700788497927,
0.96));
#65364=CARTESIAN_POINT('Ctrl Pts',(0.246589395776391,-0.00545700788497927,
1.));
#65365=CARTESIAN_POINT('Ctrl Pts',(0.246589395776391,-0.00545700788497927,
0.96));
#65366=CARTESIAN_POINT('Ctrl Pts',(0.218110534921289,-0.0341063976287842,
1.));
#65367=CARTESIAN_POINT('Ctrl Pts',(0.218110534921289,-0.0341063976287842,
0.96));
#65368=CARTESIAN_POINT('',(0.289904567971826,-0.00545700788497927,1.));
#65369=CARTESIAN_POINT('',(0.218110534921289,-0.0341063976287842,1.));
#65370=CARTESIAN_POINT('Ctrl Pts',(0.289904567971826,-0.00545700788497927,
1.));
#65371=CARTESIAN_POINT('Ctrl Pts',(0.246589395776391,-0.00545700788497927,
1.));
#65372=CARTESIAN_POINT('Ctrl Pts',(0.218110534921289,-0.0341063976287842,
1.));
#65373=CARTESIAN_POINT('',(0.289904567971826,-0.00545700788497927,0.96));
#65374=CARTESIAN_POINT('',(0.289904567971826,-0.00545700788497927,1.));
#65375=CARTESIAN_POINT('',(0.218110534921289,-0.0341063976287842,0.96));
#65376=CARTESIAN_POINT('Ctrl Pts',(0.289904567971826,-0.00545700788497927,
0.96));
#65377=CARTESIAN_POINT('Ctrl Pts',(0.246589395776391,-0.00545700788497927,
0.96));
#65378=CARTESIAN_POINT('Ctrl Pts',(0.218110534921289,-0.0341063976287842,
0.96));
#65379=CARTESIAN_POINT('',(0.218110534921289,-0.0341063976287842,1.));
#65380=CARTESIAN_POINT('Ctrl Pts',(0.363744947686791,-0.034447455406189,
1.));
#65381=CARTESIAN_POINT('Ctrl Pts',(0.363744947686791,-0.034447455406189,
0.96));
#65382=CARTESIAN_POINT('Ctrl Pts',(0.334242913499475,-0.00545700788497927,
1.));
#65383=CARTESIAN_POINT('Ctrl Pts',(0.334242913499475,-0.00545700788497927,
0.96));
#65384=CARTESIAN_POINT('Ctrl Pts',(0.289904567971826,-0.00545700788497927,
1.));
#65385=CARTESIAN_POINT('Ctrl Pts',(0.289904567971826,-0.00545700788497927,
0.96));
#65386=CARTESIAN_POINT('',(0.363744947686791,-0.034447455406189,1.));
#65387=CARTESIAN_POINT('Ctrl Pts',(0.363744947686791,-0.034447455406189,
1.));
#65388=CARTESIAN_POINT('Ctrl Pts',(0.334242913499475,-0.00545700788497927,
1.));
#65389=CARTESIAN_POINT('Ctrl Pts',(0.289904567971826,-0.00545700788497927,
1.));
#65390=CARTESIAN_POINT('',(0.363744947686791,-0.034447455406189,0.96));
#65391=CARTESIAN_POINT('',(0.363744947686791,-0.034447455406189,1.));
#65392=CARTESIAN_POINT('Ctrl Pts',(0.363744947686791,-0.034447455406189,
0.96));
#65393=CARTESIAN_POINT('Ctrl Pts',(0.334242913499475,-0.00545700788497927,
0.96));
#65394=CARTESIAN_POINT('Ctrl Pts',(0.289904567971826,-0.00545700788497927,
0.96));
#65395=CARTESIAN_POINT('Ctrl Pts',(0.393246981874108,-0.107776248455048,
1.));
#65396=CARTESIAN_POINT('Ctrl Pts',(0.393246981874108,-0.107776248455048,
0.96));
#65397=CARTESIAN_POINT('Ctrl Pts',(0.393246981874108,-0.0634379029273987,
1.));
#65398=CARTESIAN_POINT('Ctrl Pts',(0.393246981874108,-0.0634379029273987,
0.96));
#65399=CARTESIAN_POINT('Ctrl Pts',(0.363744947686791,-0.034447455406189,
1.));
#65400=CARTESIAN_POINT('Ctrl Pts',(0.363744947686791,-0.034447455406189,
0.96));
#65401=CARTESIAN_POINT('',(0.393246981874108,-0.107776248455048,1.));
#65402=CARTESIAN_POINT('Ctrl Pts',(0.393246981874108,-0.107776248455048,
1.));
#65403=CARTESIAN_POINT('Ctrl Pts',(0.393246981874108,-0.0634379029273987,
1.));
#65404=CARTESIAN_POINT('Ctrl Pts',(0.363744947686791,-0.034447455406189,
1.));
#65405=CARTESIAN_POINT('',(0.393246981874108,-0.107776248455048,0.96));
#65406=CARTESIAN_POINT('',(0.393246981874108,-0.107776248455048,1.));
#65407=CARTESIAN_POINT('Ctrl Pts',(0.393246981874108,-0.107776248455048,
0.96));
#65408=CARTESIAN_POINT('Ctrl Pts',(0.393246981874108,-0.0634379029273987,
0.96));
#65409=CARTESIAN_POINT('Ctrl Pts',(0.363744947686791,-0.034447455406189,
0.96));
#65410=CARTESIAN_POINT('Ctrl Pts',(0.364597532525659,-0.179740750789642,
1.));
#65411=CARTESIAN_POINT('Ctrl Pts',(0.364597532525659,-0.179740750789642,
0.96));
#65412=CARTESIAN_POINT('Ctrl Pts',(0.393246981874108,-0.151432418823242,
1.));
#65413=CARTESIAN_POINT('Ctrl Pts',(0.393246981874108,-0.151432418823242,
0.96));
#65414=CARTESIAN_POINT('Ctrl Pts',(0.393246981874108,-0.107776248455048,
1.));
#65415=CARTESIAN_POINT('Ctrl Pts',(0.393246981874108,-0.107776248455048,
0.96));
#65416=CARTESIAN_POINT('',(0.364597532525659,-0.179740750789642,1.));
#65417=CARTESIAN_POINT('Ctrl Pts',(0.364597532525659,-0.179740750789642,
1.));
#65418=CARTESIAN_POINT('Ctrl Pts',(0.393246981874108,-0.151432418823242,
1.));
#65419=CARTESIAN_POINT('Ctrl Pts',(0.393246981874108,-0.107776248455048,
1.));
#65420=CARTESIAN_POINT('',(0.364597532525659,-0.179740750789642,0.96));
#65421=CARTESIAN_POINT('',(0.364597532525659,-0.179740750789642,1.));
#65422=CARTESIAN_POINT('Ctrl Pts',(0.364597532525659,-0.179740750789642,
0.96));
#65423=CARTESIAN_POINT('Ctrl Pts',(0.393246981874108,-0.151432418823242,
0.96));
#65424=CARTESIAN_POINT('Ctrl Pts',(0.393246981874108,-0.107776248455048,
0.96));
#65425=CARTESIAN_POINT('Ctrl Pts',(0.291950914636254,-0.208049082756043,
1.));
#65426=CARTESIAN_POINT('Ctrl Pts',(0.291950914636254,-0.208049082756043,
0.96));
#65427=CARTESIAN_POINT('Ctrl Pts',(0.335948202386498,-0.208049082756043,
1.));
#65428=CARTESIAN_POINT('Ctrl Pts',(0.335948202386498,-0.208049082756043,
0.96));
#65429=CARTESIAN_POINT('Ctrl Pts',(0.364597532525659,-0.179740750789642,
1.));
#65430=CARTESIAN_POINT('Ctrl Pts',(0.364597532525659,-0.179740750789642,
0.96));
#65431=CARTESIAN_POINT('',(0.291950914636254,-0.208049082756043,1.));
#65432=CARTESIAN_POINT('Ctrl Pts',(0.291950914636254,-0.208049082756043,
1.));
#65433=CARTESIAN_POINT('Ctrl Pts',(0.335948202386498,-0.208049082756043,
1.));
#65434=CARTESIAN_POINT('Ctrl Pts',(0.364597532525659,-0.179740750789642,
1.));
#65435=CARTESIAN_POINT('',(0.291950914636254,-0.208049082756043,0.96));
#65436=CARTESIAN_POINT('',(0.291950914636254,-0.208049082756043,1.));
#65437=CARTESIAN_POINT('Ctrl Pts',(0.291950914636254,-0.208049082756043,
0.96));
#65438=CARTESIAN_POINT('Ctrl Pts',(0.335948202386498,-0.208049082756043,
0.96));
#65439=CARTESIAN_POINT('Ctrl Pts',(0.364597532525659,-0.179740750789642,
0.96));
#65440=CARTESIAN_POINT('Ctrl Pts',(0.239086005464196,-0.194577062129974,
1.));
#65441=CARTESIAN_POINT('Ctrl Pts',(0.239086005464196,-0.194577062129974,
0.96));
#65442=CARTESIAN_POINT('Ctrl Pts',(0.263642642274499,-0.208049082756043,
1.));
#65443=CARTESIAN_POINT('Ctrl Pts',(0.263642642274499,-0.208049082756043,
0.96));
#65444=CARTESIAN_POINT('Ctrl Pts',(0.291950914636254,-0.208049082756043,
1.));
#65445=CARTESIAN_POINT('Ctrl Pts',(0.291950914636254,-0.208049082756043,
0.96));
#65446=CARTESIAN_POINT('',(0.239086005464196,-0.194577062129974,1.));
#65447=CARTESIAN_POINT('Ctrl Pts',(0.239086005464196,-0.194577062129974,
1.));
#65448=CARTESIAN_POINT('Ctrl Pts',(0.263642642274499,-0.208049082756043,
1.));
#65449=CARTESIAN_POINT('Ctrl Pts',(0.291950914636254,-0.208049082756043,
1.));
#65450=CARTESIAN_POINT('',(0.239086005464196,-0.194577062129974,0.96));
#65451=CARTESIAN_POINT('',(0.239086005464196,-0.194577062129974,1.));
#65452=CARTESIAN_POINT('Ctrl Pts',(0.239086005464196,-0.194577062129974,
0.96));
#65453=CARTESIAN_POINT('Ctrl Pts',(0.263642642274499,-0.208049082756043,
0.96));
#65454=CARTESIAN_POINT('Ctrl Pts',(0.291950914636254,-0.208049082756043,
0.96));
#65455=CARTESIAN_POINT('Ctrl Pts',(0.202080580964685,-0.156548404693604,
1.));
#65456=CARTESIAN_POINT('Ctrl Pts',(0.202080580964685,-0.156548404693604,
0.96));
#65457=CARTESIAN_POINT('Ctrl Pts',(0.214529368653893,-0.181104981899261,
1.));
#65458=CARTESIAN_POINT('Ctrl Pts',(0.214529368653893,-0.181104981899261,
0.96));
#65459=CARTESIAN_POINT('Ctrl Pts',(0.239086005464196,-0.194577062129974,
1.));
#65460=CARTESIAN_POINT('Ctrl Pts',(0.239086005464196,-0.194577062129974,
0.96));
#65461=CARTESIAN_POINT('',(0.202080580964685,-0.156548404693604,1.));
#65462=CARTESIAN_POINT('Ctrl Pts',(0.202080580964685,-0.156548404693604,
1.));
#65463=CARTESIAN_POINT('Ctrl Pts',(0.214529368653893,-0.181104981899261,
1.));
#65464=CARTESIAN_POINT('Ctrl Pts',(0.239086005464196,-0.194577062129974,
1.));
#65465=CARTESIAN_POINT('',(0.202080580964685,-0.156548404693604,0.96));
#65466=CARTESIAN_POINT('',(0.202080580964685,-0.156548404693604,1.));
#65467=CARTESIAN_POINT('Ctrl Pts',(0.202080580964685,-0.156548404693604,
0.96));
#65468=CARTESIAN_POINT('Ctrl Pts',(0.214529368653893,-0.181104981899261,
0.96));
#65469=CARTESIAN_POINT('Ctrl Pts',(0.239086005464196,-0.194577062129974,
0.96));
#65470=CARTESIAN_POINT('Ctrl Pts',(0.189631674066186,-0.105729842185974,
1.));
#65471=CARTESIAN_POINT('Ctrl Pts',(0.189631674066186,-0.105729842185974,
0.96));
#65472=CARTESIAN_POINT('Ctrl Pts',(0.189631674066186,-0.131991767883301,
1.));
#65473=CARTESIAN_POINT('Ctrl Pts',(0.189631674066186,-0.131991767883301,
0.96));
#65474=CARTESIAN_POINT('Ctrl Pts',(0.202080580964685,-0.156548404693604,
1.));
#65475=CARTESIAN_POINT('Ctrl Pts',(0.202080580964685,-0.156548404693604,
0.96));
#65476=CARTESIAN_POINT('',(0.189631674066186,-0.105729842185974,1.));
#65477=CARTESIAN_POINT('Ctrl Pts',(0.189631674066186,-0.105729842185974,
1.));
#65478=CARTESIAN_POINT('Ctrl Pts',(0.189631674066186,-0.131991767883301,
1.));
#65479=CARTESIAN_POINT('Ctrl Pts',(0.202080580964685,-0.156548404693604,
1.));
#65480=CARTESIAN_POINT('',(0.189631674066186,-0.105729842185974,0.96));
#65481=CARTESIAN_POINT('',(0.189631674066186,-0.105729842185974,1.));
#65482=CARTESIAN_POINT('Ctrl Pts',(0.189631674066186,-0.105729842185974,
0.96));
#65483=CARTESIAN_POINT('Ctrl Pts',(0.189631674066186,-0.131991767883301,
0.96));
#65484=CARTESIAN_POINT('Ctrl Pts',(0.202080580964685,-0.156548404693604,
0.96));
#65485=CARTESIAN_POINT('Ctrl Pts',(0.218110534921289,-0.0341063976287842,
1.));
#65486=CARTESIAN_POINT('Ctrl Pts',(0.218110534921289,-0.0341063976287842,
0.96));
#65487=CARTESIAN_POINT('Ctrl Pts',(0.189631674066186,-0.0627557873725891,
1.));
#65488=CARTESIAN_POINT('Ctrl Pts',(0.189631674066186,-0.0627557873725891,
0.96));
#65489=CARTESIAN_POINT('Ctrl Pts',(0.189631674066186,-0.105729842185974,
1.));
#65490=CARTESIAN_POINT('Ctrl Pts',(0.189631674066186,-0.105729842185974,
0.96));
#65491=CARTESIAN_POINT('Ctrl Pts',(0.218110534921289,-0.0341063976287842,
1.));
#65492=CARTESIAN_POINT('Ctrl Pts',(0.189631674066186,-0.0627557873725891,
1.));
#65493=CARTESIAN_POINT('Ctrl Pts',(0.189631674066186,-0.105729842185974,
1.));
#65494=CARTESIAN_POINT('Ctrl Pts',(0.218110534921289,-0.0341063976287842,
0.96));
#65495=CARTESIAN_POINT('Ctrl Pts',(0.189631674066186,-0.0627557873725891,
0.96));
#65496=CARTESIAN_POINT('Ctrl Pts',(0.189631674066186,-0.105729842185974,
0.96));
#65497=CARTESIAN_POINT('Ctrl Pts',(0.29092774130404,0.201568937301636,1.));
#65498=CARTESIAN_POINT('Ctrl Pts',(0.29092774130404,0.201568937301636,0.96));
#65499=CARTESIAN_POINT('Ctrl Pts',(0.25579807497561,0.201568937301636,1.));
#65500=CARTESIAN_POINT('Ctrl Pts',(0.25579807497561,0.201568937301636,0.96));
#65501=CARTESIAN_POINT('Ctrl Pts',(0.232605788484216,0.179058706760406,
1.));
#65502=CARTESIAN_POINT('Ctrl Pts',(0.232605788484216,0.179058706760406,
0.96));
#65503=CARTESIAN_POINT('',(0.29092774130404,0.201568937301636,1.));
#65504=CARTESIAN_POINT('',(0.232605788484216,0.179058706760406,1.));
#65505=CARTESIAN_POINT('Ctrl Pts',(0.29092774130404,0.201568937301636,1.));
#65506=CARTESIAN_POINT('Ctrl Pts',(0.25579807497561,0.201568937301636,1.));
#65507=CARTESIAN_POINT('Ctrl Pts',(0.232605788484216,0.179058706760406,
1.));
#65508=CARTESIAN_POINT('',(0.29092774130404,0.201568937301636,0.96));
#65509=CARTESIAN_POINT('',(0.29092774130404,0.201568937301636,1.));
#65510=CARTESIAN_POINT('',(0.232605788484216,0.179058706760406,0.96));
#65511=CARTESIAN_POINT('Ctrl Pts',(0.29092774130404,0.201568937301636,0.96));
#65512=CARTESIAN_POINT('Ctrl Pts',(0.25579807497561,0.201568937301636,0.96));
#65513=CARTESIAN_POINT('Ctrl Pts',(0.232605788484216,0.179058706760406,
0.96));
#65514=CARTESIAN_POINT('',(0.232605788484216,0.179058706760406,1.));
#65515=CARTESIAN_POINT('Ctrl Pts',(0.349079224839807,0.178547120094299,
1.));
#65516=CARTESIAN_POINT('Ctrl Pts',(0.349079224839807,0.178547120094299,
0.96));
#65517=CARTESIAN_POINT('Ctrl Pts',(0.325716230645776,0.201568937301636,
1.));
#65518=CARTESIAN_POINT('Ctrl Pts',(0.325716230645776,0.201568937301636,
0.96));
#65519=CARTESIAN_POINT('Ctrl Pts',(0.29092774130404,0.201568937301636,1.));
#65520=CARTESIAN_POINT('Ctrl Pts',(0.29092774130404,0.201568937301636,0.96));
#65521=CARTESIAN_POINT('',(0.349079224839807,0.178547120094299,1.));
#65522=CARTESIAN_POINT('Ctrl Pts',(0.349079224839807,0.178547120094299,
1.));
#65523=CARTESIAN_POINT('Ctrl Pts',(0.325716230645776,0.201568937301636,
1.));
#65524=CARTESIAN_POINT('Ctrl Pts',(0.29092774130404,0.201568937301636,1.));
#65525=CARTESIAN_POINT('',(0.349079224839807,0.178547120094299,0.96));
#65526=CARTESIAN_POINT('',(0.349079224839807,0.178547120094299,1.));
#65527=CARTESIAN_POINT('Ctrl Pts',(0.349079224839807,0.178547120094299,
0.96));
#65528=CARTESIAN_POINT('Ctrl Pts',(0.325716230645776,0.201568937301636,
0.96));
#65529=CARTESIAN_POINT('Ctrl Pts',(0.29092774130404,0.201568937301636,0.96));
#65530=CARTESIAN_POINT('Ctrl Pts',(0.372442099824548,0.121759927272797,
1.));
#65531=CARTESIAN_POINT('Ctrl Pts',(0.372442099824548,0.121759927272797,
0.96));
#65532=CARTESIAN_POINT('Ctrl Pts',(0.372442099824548,0.15552527308464,1.));
#65533=CARTESIAN_POINT('Ctrl Pts',(0.372442099824548,0.15552527308464,0.96));
#65534=CARTESIAN_POINT('Ctrl Pts',(0.349079224839807,0.178547120094299,
1.));
#65535=CARTESIAN_POINT('Ctrl Pts',(0.349079224839807,0.178547120094299,
0.96));
#65536=CARTESIAN_POINT('',(0.372442099824548,0.121759927272797,1.));
#65537=CARTESIAN_POINT('Ctrl Pts',(0.372442099824548,0.121759927272797,
1.));
#65538=CARTESIAN_POINT('Ctrl Pts',(0.372442099824548,0.15552527308464,1.));
#65539=CARTESIAN_POINT('Ctrl Pts',(0.349079224839807,0.178547120094299,
1.));
#65540=CARTESIAN_POINT('',(0.372442099824548,0.121759927272797,0.96));
#65541=CARTESIAN_POINT('',(0.372442099824548,0.121759927272797,1.));
#65542=CARTESIAN_POINT('Ctrl Pts',(0.372442099824548,0.121759927272797,
0.96));
#65543=CARTESIAN_POINT('Ctrl Pts',(0.372442099824548,0.15552527308464,0.96));
#65544=CARTESIAN_POINT('Ctrl Pts',(0.349079224839807,0.178547120094299,
0.96));
#65545=CARTESIAN_POINT('Ctrl Pts',(0.349761340394616,0.0670191407203674,
1.));
#65546=CARTESIAN_POINT('Ctrl Pts',(0.349761340394616,0.0670191407203674,
0.96));
#65547=CARTESIAN_POINT('Ctrl Pts',(0.372442099824548,0.0893588423728943,
1.));
#65548=CARTESIAN_POINT('Ctrl Pts',(0.372442099824548,0.0893588423728943,
0.96));
#65549=CARTESIAN_POINT('Ctrl Pts',(0.372442099824548,0.121759927272797,
1.));
#65550=CARTESIAN_POINT('Ctrl Pts',(0.372442099824548,0.121759927272797,
0.96));
#65551=CARTESIAN_POINT('',(0.349761340394616,0.0670191407203674,1.));
#65552=CARTESIAN_POINT('Ctrl Pts',(0.349761340394616,0.0670191407203674,
1.));
#65553=CARTESIAN_POINT('Ctrl Pts',(0.372442099824548,0.0893588423728943,
1.));
#65554=CARTESIAN_POINT('Ctrl Pts',(0.372442099824548,0.121759927272797,
1.));
#65555=CARTESIAN_POINT('',(0.349761340394616,0.0670191407203674,0.96));
#65556=CARTESIAN_POINT('',(0.349761340394616,0.0670191407203674,1.));
#65557=CARTESIAN_POINT('Ctrl Pts',(0.349761340394616,0.0670191407203674,
0.96));
#65558=CARTESIAN_POINT('Ctrl Pts',(0.372442099824548,0.0893588423728943,
0.96));
#65559=CARTESIAN_POINT('Ctrl Pts',(0.372442099824548,0.121759927272797,
0.96));
#65560=CARTESIAN_POINT('Ctrl Pts',(0.29160985685885,0.0446794390678406,
1.));
#65561=CARTESIAN_POINT('Ctrl Pts',(0.29160985685885,0.0446794390678406,
0.96));
#65562=CARTESIAN_POINT('Ctrl Pts',(0.327080580964685,0.0446794390678406,
1.));
#65563=CARTESIAN_POINT('Ctrl Pts',(0.327080580964685,0.0446794390678406,
0.96));
#65564=CARTESIAN_POINT('Ctrl Pts',(0.349761340394616,0.0670191407203674,
1.));
#65565=CARTESIAN_POINT('Ctrl Pts',(0.349761340394616,0.0670191407203674,
0.96));
#65566=CARTESIAN_POINT('',(0.29160985685885,0.0446794390678406,1.));
#65567=CARTESIAN_POINT('Ctrl Pts',(0.29160985685885,0.0446794390678406,
1.));
#65568=CARTESIAN_POINT('Ctrl Pts',(0.327080580964685,0.0446794390678406,
1.));
#65569=CARTESIAN_POINT('Ctrl Pts',(0.349761340394616,0.0670191407203674,
1.));
#65570=CARTESIAN_POINT('',(0.29160985685885,0.0446794390678406,0.96));
#65571=CARTESIAN_POINT('',(0.29160985685885,0.0446794390678406,1.));
#65572=CARTESIAN_POINT('Ctrl Pts',(0.29160985685885,0.0446794390678406,
0.96));
#65573=CARTESIAN_POINT('Ctrl Pts',(0.327080580964685,0.0446794390678406,
0.96));
#65574=CARTESIAN_POINT('Ctrl Pts',(0.349761340394616,0.0670191407203674,
0.96));
#65575=CARTESIAN_POINT('Ctrl Pts',(0.232264730706811,0.0671896696090698,
1.));
#65576=CARTESIAN_POINT('Ctrl Pts',(0.232264730706811,0.0671896696090698,
0.96));
#65577=CARTESIAN_POINT('Ctrl Pts',(0.2551159594208,0.0446794390678406,1.));
#65578=CARTESIAN_POINT('Ctrl Pts',(0.2551159594208,0.0446794390678406,0.96));
#65579=CARTESIAN_POINT('Ctrl Pts',(0.29160985685885,0.0446794390678406,
1.));
#65580=CARTESIAN_POINT('Ctrl Pts',(0.29160985685885,0.0446794390678406,
0.96));
#65581=CARTESIAN_POINT('',(0.232264730706811,0.0671896696090698,1.));
#65582=CARTESIAN_POINT('Ctrl Pts',(0.232264730706811,0.0671896696090698,
1.));
#65583=CARTESIAN_POINT('Ctrl Pts',(0.2551159594208,0.0446794390678406,1.));
#65584=CARTESIAN_POINT('Ctrl Pts',(0.29160985685885,0.0446794390678406,
1.));
#65585=CARTESIAN_POINT('',(0.232264730706811,0.0671896696090698,0.96));
#65586=CARTESIAN_POINT('',(0.232264730706811,0.0671896696090698,1.));
#65587=CARTESIAN_POINT('Ctrl Pts',(0.232264730706811,0.0671896696090698,
0.96));
#65588=CARTESIAN_POINT('Ctrl Pts',(0.2551159594208,0.0446794390678406,0.96));
#65589=CARTESIAN_POINT('Ctrl Pts',(0.29160985685885,0.0446794390678406,
0.96));
#65590=CARTESIAN_POINT('Ctrl Pts',(0.209413382783532,0.125170594453812,
1.));
#65591=CARTESIAN_POINT('Ctrl Pts',(0.209413382783532,0.125170594453812,
0.96));
#65592=CARTESIAN_POINT('Ctrl Pts',(0.209413382783532,0.0896999001502991,
1.));
#65593=CARTESIAN_POINT('Ctrl Pts',(0.209413382783532,0.0896999001502991,
0.96));
#65594=CARTESIAN_POINT('Ctrl Pts',(0.232264730706811,0.0671896696090698,
1.));
#65595=CARTESIAN_POINT('Ctrl Pts',(0.232264730706811,0.0671896696090698,
0.96));
#65596=CARTESIAN_POINT('',(0.209413382783532,0.125170594453812,1.));
#65597=CARTESIAN_POINT('Ctrl Pts',(0.209413382783532,0.125170594453812,
1.));
#65598=CARTESIAN_POINT('Ctrl Pts',(0.209413382783532,0.0896999001502991,
1.));
#65599=CARTESIAN_POINT('Ctrl Pts',(0.232264730706811,0.0671896696090698,
1.));
#65600=CARTESIAN_POINT('',(0.209413382783532,0.125170594453812,0.96));
#65601=CARTESIAN_POINT('',(0.209413382783532,0.125170594453812,1.));
#65602=CARTESIAN_POINT('Ctrl Pts',(0.209413382783532,0.125170594453812,
0.96));
#65603=CARTESIAN_POINT('Ctrl Pts',(0.209413382783532,0.0896999001502991,
0.96));
#65604=CARTESIAN_POINT('Ctrl Pts',(0.232264730706811,0.0671896696090698,
0.96));
#65605=CARTESIAN_POINT('Ctrl Pts',(0.232605788484216,0.179058706760406,
1.));
#65606=CARTESIAN_POINT('Ctrl Pts',(0.232605788484216,0.179058706760406,
0.96));
#65607=CARTESIAN_POINT('Ctrl Pts',(0.209413382783532,0.156548476219177,
1.));
#65608=CARTESIAN_POINT('Ctrl Pts',(0.209413382783532,0.156548476219177,
0.96));
#65609=CARTESIAN_POINT('Ctrl Pts',(0.209413382783532,0.125170594453812,
1.));
#65610=CARTESIAN_POINT('Ctrl Pts',(0.209413382783532,0.125170594453812,
0.96));
#65611=CARTESIAN_POINT('Ctrl Pts',(0.232605788484216,0.179058706760406,
1.));
#65612=CARTESIAN_POINT('Ctrl Pts',(0.209413382783532,0.156548476219177,
1.));
#65613=CARTESIAN_POINT('Ctrl Pts',(0.209413382783532,0.125170594453812,
1.));
#65614=CARTESIAN_POINT('Ctrl Pts',(0.232605788484216,0.179058706760406,
0.96));
#65615=CARTESIAN_POINT('Ctrl Pts',(0.209413382783532,0.156548476219177,
0.96));
#65616=CARTESIAN_POINT('Ctrl Pts',(0.209413382783532,0.125170594453812,
0.96));
#65617=CARTESIAN_POINT('Ctrl Pts',(0.171896312013268,-0.214699828624725,
1.));
#65618=CARTESIAN_POINT('Ctrl Pts',(0.171896312013268,-0.214699828624725,
0.96));
#65619=CARTESIAN_POINT('Ctrl Pts',(0.126534793153405,-0.170873069763184,
1.));
#65620=CARTESIAN_POINT('Ctrl Pts',(0.126534793153405,-0.170873069763184,
0.96));
#65621=CARTESIAN_POINT('Ctrl Pts',(0.126534793153405,-0.105388784408569,
1.));
#65622=CARTESIAN_POINT('Ctrl Pts',(0.126534793153405,-0.105388784408569,
0.96));
#65623=CARTESIAN_POINT('',(0.171896312013268,-0.214699828624725,1.));
#65624=CARTESIAN_POINT('',(0.126534793153405,-0.105388784408569,1.));
#65625=CARTESIAN_POINT('Ctrl Pts',(0.171896312013268,-0.214699828624725,
1.));
#65626=CARTESIAN_POINT('Ctrl Pts',(0.126534793153405,-0.170873069763184,
1.));
#65627=CARTESIAN_POINT('Ctrl Pts',(0.126534793153405,-0.105388784408569,
1.));
#65628=CARTESIAN_POINT('',(0.171896312013268,-0.214699828624725,0.96));
#65629=CARTESIAN_POINT('',(0.171896312013268,-0.214699828624725,1.));
#65630=CARTESIAN_POINT('',(0.126534793153405,-0.105388784408569,0.96));
#65631=CARTESIAN_POINT('Ctrl Pts',(0.171896312013268,-0.214699828624725,
0.96));
#65632=CARTESIAN_POINT('Ctrl Pts',(0.126534793153405,-0.170873069763184,
0.96));
#65633=CARTESIAN_POINT('Ctrl Pts',(0.126534793153405,-0.105388784408569,
0.96));
#65634=CARTESIAN_POINT('',(0.126534793153405,-0.105388784408569,1.));
#65635=CARTESIAN_POINT('Ctrl Pts',(0.291268799081445,-0.258526587486267,
1.));
#65636=CARTESIAN_POINT('Ctrl Pts',(0.291268799081445,-0.258526587486267,
0.96));
#65637=CARTESIAN_POINT('Ctrl Pts',(0.217257830873132,-0.258526587486267,
1.));
#65638=CARTESIAN_POINT('Ctrl Pts',(0.217257830873132,-0.258526587486267,
0.96));
#65639=CARTESIAN_POINT('Ctrl Pts',(0.171896312013268,-0.214699828624725,
1.));
#65640=CARTESIAN_POINT('Ctrl Pts',(0.171896312013268,-0.214699828624725,
0.96));
#65641=CARTESIAN_POINT('',(0.291268799081445,-0.258526587486267,1.));
#65642=CARTESIAN_POINT('Ctrl Pts',(0.291268799081445,-0.258526587486267,
1.));
#65643=CARTESIAN_POINT('Ctrl Pts',(0.217257830873132,-0.258526587486267,
1.));
#65644=CARTESIAN_POINT('Ctrl Pts',(0.171896312013268,-0.214699828624725,
1.));
#65645=CARTESIAN_POINT('',(0.291268799081445,-0.258526587486267,0.96));
#65646=CARTESIAN_POINT('',(0.291268799081445,-0.258526587486267,1.));
#65647=CARTESIAN_POINT('Ctrl Pts',(0.291268799081445,-0.258526587486267,
0.96));
#65648=CARTESIAN_POINT('Ctrl Pts',(0.217257830873132,-0.258526587486267,
0.96));
#65649=CARTESIAN_POINT('Ctrl Pts',(0.171896312013268,-0.214699828624725,
0.96));
#65650=CARTESIAN_POINT('Ctrl Pts',(0.410641286149621,-0.214870357513428,
1.));
#65651=CARTESIAN_POINT('Ctrl Pts',(0.410641286149621,-0.214870357513428,
0.96));
#65652=CARTESIAN_POINT('Ctrl Pts',(0.365279767289758,-0.258526587486267,
1.));
#65653=CARTESIAN_POINT('Ctrl Pts',(0.365279767289758,-0.258526587486267,
0.96));
#65654=CARTESIAN_POINT('Ctrl Pts',(0.291268799081445,-0.258526587486267,
1.));
#65655=CARTESIAN_POINT('Ctrl Pts',(0.291268799081445,-0.258526587486267,
0.96));
#65656=CARTESIAN_POINT('',(0.410641286149621,-0.214870357513428,1.));
#65657=CARTESIAN_POINT('Ctrl Pts',(0.410641286149621,-0.214870357513428,
1.));
#65658=CARTESIAN_POINT('Ctrl Pts',(0.365279767289758,-0.258526587486267,
1.));
#65659=CARTESIAN_POINT('Ctrl Pts',(0.291268799081445,-0.258526587486267,
1.));
#65660=CARTESIAN_POINT('',(0.410641286149621,-0.214870357513428,0.96));
#65661=CARTESIAN_POINT('',(0.410641286149621,-0.214870357513428,1.));
#65662=CARTESIAN_POINT('Ctrl Pts',(0.410641286149621,-0.214870357513428,
0.96));
#65663=CARTESIAN_POINT('Ctrl Pts',(0.365279767289758,-0.258526587486267,
0.96));
#65664=CARTESIAN_POINT('Ctrl Pts',(0.291268799081445,-0.258526587486267,
0.96));
#65665=CARTESIAN_POINT('Ctrl Pts',(0.456002805009484,-0.107094132900238,
1.));
#65666=CARTESIAN_POINT('Ctrl Pts',(0.456002805009484,-0.107094132900238,
0.96));
#65667=CARTESIAN_POINT('Ctrl Pts',(0.456002805009484,-0.171214127540588,
1.));
#65668=CARTESIAN_POINT('Ctrl Pts',(0.456002805009484,-0.171214127540588,
0.96));
#65669=CARTESIAN_POINT('Ctrl Pts',(0.410641286149621,-0.214870357513428,
1.));
#65670=CARTESIAN_POINT('Ctrl Pts',(0.410641286149621,-0.214870357513428,
0.96));
#65671=CARTESIAN_POINT('',(0.456002805009484,-0.107094132900238,1.));
#65672=CARTESIAN_POINT('Ctrl Pts',(0.456002805009484,-0.107094132900238,
1.));
#65673=CARTESIAN_POINT('Ctrl Pts',(0.456002805009484,-0.171214127540588,
1.));
#65674=CARTESIAN_POINT('Ctrl Pts',(0.410641286149621,-0.214870357513428,
1.));
#65675=CARTESIAN_POINT('',(0.456002805009484,-0.107094132900238,0.96));
#65676=CARTESIAN_POINT('',(0.456002805009484,-0.107094132900238,1.));
#65677=CARTESIAN_POINT('Ctrl Pts',(0.456002805009484,-0.107094132900238,
0.96));
#65678=CARTESIAN_POINT('Ctrl Pts',(0.456002805009484,-0.171214127540588,
0.96));
#65679=CARTESIAN_POINT('Ctrl Pts',(0.410641286149621,-0.214870357513428,
0.96));
#65680=CARTESIAN_POINT('Ctrl Pts',(0.431957814469934,-0.0272850632667542,
1.));
#65681=CARTESIAN_POINT('Ctrl Pts',(0.431957814469934,-0.0272850632667542,
0.96));
#65682=CARTESIAN_POINT('Ctrl Pts',(0.456002805009484,-0.0607093811035156,
1.));
#65683=CARTESIAN_POINT('Ctrl Pts',(0.456002805009484,-0.0607093811035156,
0.96));
#65684=CARTESIAN_POINT('Ctrl Pts',(0.456002805009484,-0.107094132900238,
1.));
#65685=CARTESIAN_POINT('Ctrl Pts',(0.456002805009484,-0.107094132900238,
0.96));
#65686=CARTESIAN_POINT('',(0.431957814469934,-0.0272850632667542,1.));
#65687=CARTESIAN_POINT('Ctrl Pts',(0.431957814469934,-0.0272850632667542,
1.));
#65688=CARTESIAN_POINT('Ctrl Pts',(0.456002805009484,-0.0607093811035156,
1.));
#65689=CARTESIAN_POINT('Ctrl Pts',(0.456002805009484,-0.107094132900238,
1.));
#65690=CARTESIAN_POINT('',(0.431957814469934,-0.0272850632667542,0.96));
#65691=CARTESIAN_POINT('',(0.431957814469934,-0.0272850632667542,1.));
#65692=CARTESIAN_POINT('Ctrl Pts',(0.431957814469934,-0.0272850632667542,
0.96));
#65693=CARTESIAN_POINT('Ctrl Pts',(0.456002805009484,-0.0607093811035156,
0.96));
#65694=CARTESIAN_POINT('Ctrl Pts',(0.456002805009484,-0.107094132900238,
0.96));
#65695=CARTESIAN_POINT('Ctrl Pts',(0.36186907030642,0.021146035194397,1.));
#65696=CARTESIAN_POINT('Ctrl Pts',(0.36186907030642,0.021146035194397,0.96));
#65697=CARTESIAN_POINT('Ctrl Pts',(0.407912704721093,0.00613919496536253,
1.));
#65698=CARTESIAN_POINT('Ctrl Pts',(0.407912704721093,0.00613919496536253,
0.96));
#65699=CARTESIAN_POINT('Ctrl Pts',(0.431957814469934,-0.0272850632667542,
1.));
#65700=CARTESIAN_POINT('Ctrl Pts',(0.431957814469934,-0.0272850632667542,
0.96));
#65701=CARTESIAN_POINT('',(0.36186907030642,0.021146035194397,1.));
#65702=CARTESIAN_POINT('Ctrl Pts',(0.36186907030642,0.021146035194397,1.));
#65703=CARTESIAN_POINT('Ctrl Pts',(0.407912704721093,0.00613919496536253,
1.));
#65704=CARTESIAN_POINT('Ctrl Pts',(0.431957814469934,-0.0272850632667542,
1.));
#65705=CARTESIAN_POINT('',(0.36186907030642,0.021146035194397,0.96));
#65706=CARTESIAN_POINT('',(0.36186907030642,0.021146035194397,1.));
#65707=CARTESIAN_POINT('Ctrl Pts',(0.36186907030642,0.021146035194397,0.96));
#65708=CARTESIAN_POINT('Ctrl Pts',(0.407912704721093,0.00613919496536253,
0.96));
#65709=CARTESIAN_POINT('Ctrl Pts',(0.431957814469934,-0.0272850632667542,
0.96));
#65710=CARTESIAN_POINT('Ctrl Pts',(0.417291972413659,0.0608799815177917,
1.));
#65711=CARTESIAN_POINT('Ctrl Pts',(0.417291972413659,0.0608799815177917,
0.96));
#65712=CARTESIAN_POINT('Ctrl Pts',(0.399045083299279,0.0351296424865722,
1.));
#65713=CARTESIAN_POINT('Ctrl Pts',(0.399045083299279,0.0351296424865722,
0.96));
#65714=CARTESIAN_POINT('Ctrl Pts',(0.36186907030642,0.021146035194397,1.));
#65715=CARTESIAN_POINT('Ctrl Pts',(0.36186907030642,0.021146035194397,0.96));
#65716=CARTESIAN_POINT('',(0.417291972413659,0.0608799815177917,1.));
#65717=CARTESIAN_POINT('Ctrl Pts',(0.417291972413659,0.0608799815177917,
1.));
#65718=CARTESIAN_POINT('Ctrl Pts',(0.399045083299279,0.0351296424865722,
1.));
#65719=CARTESIAN_POINT('Ctrl Pts',(0.36186907030642,0.021146035194397,1.));
#65720=CARTESIAN_POINT('',(0.417291972413659,0.0608799815177917,0.96));
#65721=CARTESIAN_POINT('',(0.417291972413659,0.0608799815177917,1.));
#65722=CARTESIAN_POINT('Ctrl Pts',(0.417291972413659,0.0608799815177917,
0.96));
#65723=CARTESIAN_POINT('Ctrl Pts',(0.399045083299279,0.0351296424865722,
0.96));
#65724=CARTESIAN_POINT('Ctrl Pts',(0.36186907030642,0.021146035194397,0.96));
#65725=CARTESIAN_POINT('Ctrl Pts',(0.435538980737329,0.121418869495392,
1.));
#65726=CARTESIAN_POINT('Ctrl Pts',(0.435538980737329,0.121418869495392,
0.96));
#65727=CARTESIAN_POINT('Ctrl Pts',(0.435538980737329,0.0866303205490112,
1.));
#65728=CARTESIAN_POINT('Ctrl Pts',(0.435538980737329,0.0866303205490112,
0.96));
#65729=CARTESIAN_POINT('Ctrl Pts',(0.417291972413659,0.0608799815177917,
1.));
#65730=CARTESIAN_POINT('Ctrl Pts',(0.417291972413659,0.0608799815177917,
0.96));
#65731=CARTESIAN_POINT('',(0.435538980737329,0.121418869495392,1.));
#65732=CARTESIAN_POINT('Ctrl Pts',(0.435538980737329,0.121418869495392,
1.));
#65733=CARTESIAN_POINT('Ctrl Pts',(0.435538980737329,0.0866303205490112,
1.));
#65734=CARTESIAN_POINT('Ctrl Pts',(0.417291972413659,0.0608799815177917,
1.));
#65735=CARTESIAN_POINT('',(0.435538980737329,0.121418869495392,0.96));
#65736=CARTESIAN_POINT('',(0.435538980737329,0.121418869495392,1.));
#65737=CARTESIAN_POINT('Ctrl Pts',(0.435538980737329,0.121418869495392,
0.96));
#65738=CARTESIAN_POINT('Ctrl Pts',(0.435538980737329,0.0866303205490112,
0.96));
#65739=CARTESIAN_POINT('Ctrl Pts',(0.417291972413659,0.0608799815177917,
0.96));
#65740=CARTESIAN_POINT('Ctrl Pts',(0.395634386315942,0.214017784595489,
1.));
#65741=CARTESIAN_POINT('Ctrl Pts',(0.395634386315942,0.214017784595489,
0.96));
#65742=CARTESIAN_POINT('Ctrl Pts',(0.435538980737329,0.175989127159119,
1.));
#65743=CARTESIAN_POINT('Ctrl Pts',(0.435538980737329,0.175989127159119,
0.96));
#65744=CARTESIAN_POINT('Ctrl Pts',(0.435538980737329,0.121418869495392,
1.));
#65745=CARTESIAN_POINT('Ctrl Pts',(0.435538980737329,0.121418869495392,
0.96));
#65746=CARTESIAN_POINT('',(0.395634386315942,0.214017784595489,1.));
#65747=CARTESIAN_POINT('Ctrl Pts',(0.395634386315942,0.214017784595489,
1.));
#65748=CARTESIAN_POINT('Ctrl Pts',(0.435538980737329,0.175989127159119,
1.));
#65749=CARTESIAN_POINT('Ctrl Pts',(0.435538980737329,0.121418869495392,
1.));
#65750=CARTESIAN_POINT('',(0.395634386315942,0.214017784595489,0.96));
#65751=CARTESIAN_POINT('',(0.395634386315942,0.214017784595489,1.));
#65752=CARTESIAN_POINT('Ctrl Pts',(0.395634386315942,0.214017784595489,
0.96));
#65753=CARTESIAN_POINT('Ctrl Pts',(0.435538980737329,0.175989127159119,
0.96));
#65754=CARTESIAN_POINT('Ctrl Pts',(0.435538980737329,0.121418869495392,
0.96));
#65755=CARTESIAN_POINT('Ctrl Pts',(0.29024562574923,0.252046382427216,1.));
#65756=CARTESIAN_POINT('Ctrl Pts',(0.29024562574923,0.252046382427216,0.96));
#65757=CARTESIAN_POINT('Ctrl Pts',(0.355729911103845,0.252046382427216,
1.));
#65758=CARTESIAN_POINT('Ctrl Pts',(0.355729911103845,0.252046382427216,
0.96));
#65759=CARTESIAN_POINT('Ctrl Pts',(0.395634386315942,0.214017784595489,
1.));
#65760=CARTESIAN_POINT('Ctrl Pts',(0.395634386315942,0.214017784595489,
0.96));
#65761=CARTESIAN_POINT('',(0.29024562574923,0.252046382427216,1.));
#65762=CARTESIAN_POINT('Ctrl Pts',(0.29024562574923,0.252046382427216,1.));
#65763=CARTESIAN_POINT('Ctrl Pts',(0.355729911103845,0.252046382427216,
1.));
#65764=CARTESIAN_POINT('Ctrl Pts',(0.395634386315942,0.214017784595489,
1.));
#65765=CARTESIAN_POINT('',(0.29024562574923,0.252046382427216,0.96));
#65766=CARTESIAN_POINT('',(0.29024562574923,0.252046382427216,1.));
#65767=CARTESIAN_POINT('Ctrl Pts',(0.29024562574923,0.252046382427216,0.96));
#65768=CARTESIAN_POINT('Ctrl Pts',(0.355729911103845,0.252046382427216,
0.96));
#65769=CARTESIAN_POINT('Ctrl Pts',(0.395634386315942,0.214017784595489,
0.96));
#65770=CARTESIAN_POINT('Ctrl Pts',(0.185880038514733,0.214870429039001,
1.));
#65771=CARTESIAN_POINT('Ctrl Pts',(0.185880038514733,0.214870429039001,
0.96));
#65772=CARTESIAN_POINT('Ctrl Pts',(0.225102398172021,0.252046382427216,
1.));
#65773=CARTESIAN_POINT('Ctrl Pts',(0.225102398172021,0.252046382427216,
0.96));
#65774=CARTESIAN_POINT('Ctrl Pts',(0.29024562574923,0.252046382427216,1.));
#65775=CARTESIAN_POINT('Ctrl Pts',(0.29024562574923,0.252046382427216,0.96));
#65776=CARTESIAN_POINT('',(0.185880038514733,0.214870429039001,1.));
#65777=CARTESIAN_POINT('Ctrl Pts',(0.185880038514733,0.214870429039001,
1.));
#65778=CARTESIAN_POINT('Ctrl Pts',(0.225102398172021,0.252046382427216,
1.));
#65779=CARTESIAN_POINT('Ctrl Pts',(0.29024562574923,0.252046382427216,1.));
#65780=CARTESIAN_POINT('',(0.185880038514733,0.214870429039001,0.96));
#65781=CARTESIAN_POINT('',(0.185880038514733,0.214870429039001,1.));
#65782=CARTESIAN_POINT('Ctrl Pts',(0.185880038514733,0.214870429039001,
0.96));
#65783=CARTESIAN_POINT('Ctrl Pts',(0.225102398172021,0.252046382427216,
0.96));
#65784=CARTESIAN_POINT('Ctrl Pts',(0.29024562574923,0.252046382427216,0.96));
#65785=CARTESIAN_POINT('Ctrl Pts',(0.146657559648156,0.123124188184738,
1.));
#65786=CARTESIAN_POINT('Ctrl Pts',(0.146657559648156,0.123124188184738,
0.96));
#65787=CARTESIAN_POINT('Ctrl Pts',(0.146657559648156,0.177694445848465,
1.));
#65788=CARTESIAN_POINT('Ctrl Pts',(0.146657559648156,0.177694445848465,
0.96));
#65789=CARTESIAN_POINT('Ctrl Pts',(0.185880038514733,0.214870429039001,
1.));
#65790=CARTESIAN_POINT('Ctrl Pts',(0.185880038514733,0.214870429039001,
0.96));
#65791=CARTESIAN_POINT('',(0.146657559648156,0.123124188184738,1.));
#65792=CARTESIAN_POINT('Ctrl Pts',(0.146657559648156,0.123124188184738,
1.));
#65793=CARTESIAN_POINT('Ctrl Pts',(0.146657559648156,0.177694445848465,
1.));
#65794=CARTESIAN_POINT('Ctrl Pts',(0.185880038514733,0.214870429039001,
1.));
#65795=CARTESIAN_POINT('',(0.146657559648156,0.123124188184738,0.96));
#65796=CARTESIAN_POINT('',(0.146657559648156,0.123124188184738,1.));
#65797=CARTESIAN_POINT('Ctrl Pts',(0.146657559648156,0.123124188184738,
0.96));
#65798=CARTESIAN_POINT('Ctrl Pts',(0.146657559648156,0.177694445848465,
0.96));
#65799=CARTESIAN_POINT('Ctrl Pts',(0.185880038514733,0.214870429039001,
0.96));
#65800=CARTESIAN_POINT('Ctrl Pts',(0.165075037255883,0.0610505104064941,
1.));
#65801=CARTESIAN_POINT('Ctrl Pts',(0.165075037255883,0.0610505104064941,
0.96));
#65802=CARTESIAN_POINT('Ctrl Pts',(0.146657559648156,0.0869714081287384,
1.));
#65803=CARTESIAN_POINT('Ctrl Pts',(0.146657559648156,0.0869714081287384,
0.96));
#65804=CARTESIAN_POINT('Ctrl Pts',(0.146657559648156,0.123124188184738,
1.));
#65805=CARTESIAN_POINT('Ctrl Pts',(0.146657559648156,0.123124188184738,
0.96));
#65806=CARTESIAN_POINT('',(0.165075037255883,0.0610505104064941,1.));
#65807=CARTESIAN_POINT('Ctrl Pts',(0.165075037255883,0.0610505104064941,
1.));
#65808=CARTESIAN_POINT('Ctrl Pts',(0.146657559648156,0.0869714081287384,
1.));
#65809=CARTESIAN_POINT('Ctrl Pts',(0.146657559648156,0.123124188184738,
1.));
#65810=CARTESIAN_POINT('',(0.165075037255883,0.0610505104064941,0.96));
#65811=CARTESIAN_POINT('',(0.165075037255883,0.0610505104064941,1.));
#65812=CARTESIAN_POINT('Ctrl Pts',(0.165075037255883,0.0610505104064941,
0.96));
#65813=CARTESIAN_POINT('Ctrl Pts',(0.146657559648156,0.0869714081287384,
0.96));
#65814=CARTESIAN_POINT('Ctrl Pts',(0.146657559648156,0.123124188184738,
0.96));
#65815=CARTESIAN_POINT('Ctrl Pts',(0.221691701188684,0.021146035194397,
1.));
#65816=CARTESIAN_POINT('Ctrl Pts',(0.221691701188684,0.021146035194397,
0.96));
#65817=CARTESIAN_POINT('Ctrl Pts',(0.18349251486361,0.0351296424865722,
1.));
#65818=CARTESIAN_POINT('Ctrl Pts',(0.18349251486361,0.0351296424865722,
0.96));
#65819=CARTESIAN_POINT('Ctrl Pts',(0.165075037255883,0.0610505104064941,
1.));
#65820=CARTESIAN_POINT('Ctrl Pts',(0.165075037255883,0.0610505104064941,
0.96));
#65821=CARTESIAN_POINT('',(0.221691701188684,0.021146035194397,1.));
#65822=CARTESIAN_POINT('Ctrl Pts',(0.221691701188684,0.021146035194397,
1.));
#65823=CARTESIAN_POINT('Ctrl Pts',(0.18349251486361,0.0351296424865722,
1.));
#65824=CARTESIAN_POINT('Ctrl Pts',(0.165075037255883,0.0610505104064941,
1.));
#65825=CARTESIAN_POINT('',(0.221691701188684,0.021146035194397,0.96));
#65826=CARTESIAN_POINT('',(0.221691701188684,0.021146035194397,1.));
#65827=CARTESIAN_POINT('Ctrl Pts',(0.221691701188684,0.021146035194397,
0.96));
#65828=CARTESIAN_POINT('Ctrl Pts',(0.18349251486361,0.0351296424865722,
0.96));
#65829=CARTESIAN_POINT('Ctrl Pts',(0.165075037255883,0.0610505104064941,
0.96));
#65830=CARTESIAN_POINT('Ctrl Pts',(0.151262018457055,-0.0237038969993592,
1.));
#65831=CARTESIAN_POINT('Ctrl Pts',(0.151262018457055,-0.0237038969993592,
0.96));
#65832=CARTESIAN_POINT('Ctrl Pts',(0.175989124551415,0.00920877456665037,
1.));
#65833=CARTESIAN_POINT('Ctrl Pts',(0.175989124551415,0.00920877456665037,
0.96));
#65834=CARTESIAN_POINT('Ctrl Pts',(0.221691701188684,0.021146035194397,
1.));
#65835=CARTESIAN_POINT('Ctrl Pts',(0.221691701188684,0.021146035194397,
0.96));
#65836=CARTESIAN_POINT('',(0.151262018457055,-0.0237038969993592,1.));
#65837=CARTESIAN_POINT('Ctrl Pts',(0.151262018457055,-0.0237038969993592,
1.));
#65838=CARTESIAN_POINT('Ctrl Pts',(0.175989124551415,0.00920877456665037,
1.));
#65839=CARTESIAN_POINT('Ctrl Pts',(0.221691701188684,0.021146035194397,
1.));
#65840=CARTESIAN_POINT('',(0.151262018457055,-0.0237038969993592,0.96));
#65841=CARTESIAN_POINT('',(0.151262018457055,-0.0237038969993592,1.));
#65842=CARTESIAN_POINT('Ctrl Pts',(0.151262018457055,-0.0237038969993592,
0.96));
#65843=CARTESIAN_POINT('Ctrl Pts',(0.175989124551415,0.00920877456665037,
0.96));
#65844=CARTESIAN_POINT('Ctrl Pts',(0.221691701188684,0.021146035194397,
0.96));
#65845=CARTESIAN_POINT('Ctrl Pts',(0.126534793153405,-0.105388784408569,
1.));
#65846=CARTESIAN_POINT('Ctrl Pts',(0.126534793153405,-0.105388784408569,
0.96));
#65847=CARTESIAN_POINT('Ctrl Pts',(0.126534793153405,-0.0566166281700134,
1.));
#65848=CARTESIAN_POINT('Ctrl Pts',(0.126534793153405,-0.0566166281700134,
0.96));
#65849=CARTESIAN_POINT('Ctrl Pts',(0.151262018457055,-0.0237038969993592,
1.));
#65850=CARTESIAN_POINT('Ctrl Pts',(0.151262018457055,-0.0237038969993592,
0.96));
#65851=CARTESIAN_POINT('Ctrl Pts',(0.126534793153405,-0.105388784408569,
1.));
#65852=CARTESIAN_POINT('Ctrl Pts',(0.126534793153405,-0.0566166281700134,
1.));
#65853=CARTESIAN_POINT('Ctrl Pts',(0.151262018457055,-0.0237038969993592,
1.));
#65854=CARTESIAN_POINT('Ctrl Pts',(0.126534793153405,-0.105388784408569,
0.96));
#65855=CARTESIAN_POINT('Ctrl Pts',(0.126534793153405,-0.0566166281700134,
0.96));
#65856=CARTESIAN_POINT('Ctrl Pts',(0.151262018457055,-0.0237038969993592,
0.96));
#65857=CARTESIAN_POINT('Origin',(0.291268799081445,-0.00324010252952578,
0.96));
#65858=CARTESIAN_POINT('Origin',(0.,0.,1.));
#65859=CARTESIAN_POINT('Origin',(0.,0.,1.));
#65860=CARTESIAN_POINT('Origin',(0.,0.,1.));
#65861=CARTESIAN_POINT('Origin',(0.,0.,1.));
#65862=CARTESIAN_POINT('Origin',(1.87869726832665E-16,-4.25270154953079E-17,
-0.0599999999999987));
#65863=CARTESIAN_POINT('Ctrl Pts',(0.564519729112616,0.374023388155322,
-0.06));
#65864=CARTESIAN_POINT('Ctrl Pts',(0.556017057337338,0.389715461663178,
-0.0599999999999997));
#65865=CARTESIAN_POINT('Ctrl Pts',(0.546881793340869,0.405030545447623,
-0.0600000000000022));
#65866=CARTESIAN_POINT('Ctrl Pts',(0.537121082038997,0.419926055265349,
-0.0600000000000023));
#65867=CARTESIAN_POINT('Ctrl Pts',(0.521265382290218,0.444122932313598,
-0.0600000000000025));
#65868=CARTESIAN_POINT('Ctrl Pts',(0.503760937756791,0.467213595952793,
-0.0600000000000015));
#65869=CARTESIAN_POINT('Ctrl Pts',(0.484792757621966,0.489116897605382,
-0.060000000000003));
#65870=CARTESIAN_POINT('Ctrl Pts',(0.477747354694951,0.497252500730066,
-0.0600000000000035));
#65871=CARTESIAN_POINT('Ctrl Pts',(0.47049970935453,0.505224152689485,-0.0600000000000051));
#65872=CARTESIAN_POINT('Ctrl Pts',(0.463058313081755,0.513027130461428,
-0.0600000000000055));
#65873=CARTESIAN_POINT('Ctrl Pts',(0.457142398647175,0.519230502401535,
-0.0600000000000059));
#65874=CARTESIAN_POINT('Ctrl Pts',(0.451104521358182,0.525326494138705,
-0.0600000000000083));
#65875=CARTESIAN_POINT('Ctrl Pts',(0.444958706598096,0.531303709121088,
-0.0600000000000078));
#65876=CARTESIAN_POINT('Ctrl Pts',(0.420677607542062,0.554918698301855,
-0.0600000000000056));
#65877=CARTESIAN_POINT('Ctrl Pts',(0.394678481543999,0.576721462967644,
-0.06));
#65878=CARTESIAN_POINT('Ctrl Pts',(0.367241084736883,0.596581858045739,
-0.0599999999999993));
#65879=CARTESIAN_POINT('Ctrl Pts',(0.349962505322962,0.60908885409792,-0.059999999999999));
#65880=CARTESIAN_POINT('Ctrl Pts',(0.332112498690617,0.620825037936489,
-0.0600000000000051));
#65881=CARTESIAN_POINT('Ctrl Pts',(0.313752738001227,0.631750795096854,
-0.0600000000000059));
#65882=CARTESIAN_POINT('Ctrl Pts',(0.307066444369792,0.635729758753072,
-0.0600000000000062));
#65883=CARTESIAN_POINT('Ctrl Pts',(0.300320585088648,0.639596340261989,
-0.0600000000000039));
#65884=CARTESIAN_POINT('Ctrl Pts',(0.293519801750991,0.643348510928835,
-0.0600000000000039));
#65885=CARTESIAN_POINT('Ctrl Pts',(0.289341260343745,0.645653921896958,
-0.0600000000000039));
#65886=CARTESIAN_POINT('Ctrl Pts',(0.285141833540485,0.647916228279921,
-0.0600000000000032));
#65887=CARTESIAN_POINT('Ctrl Pts',(0.280922298401405,0.650135110019904,
-0.0600000000000031));
#65888=CARTESIAN_POINT('Ctrl Pts',(0.25053489436036,0.666114608644694,-0.060000000000002));
#65889=CARTESIAN_POINT('Ctrl Pts',(0.219107606892874,0.679845250773148,
-0.0600000000000015));
#65890=CARTESIAN_POINT('Ctrl Pts',(0.186893278148277,0.691299397430587,
-0.0600000000000007));
#65891=CARTESIAN_POINT('Ctrl Pts',(0.154590738619216,0.702784908369121,
-0.0599999999999998));
#65892=CARTESIAN_POINT('Ctrl Pts',(0.121495760592277,0.711981939343559,
-0.0600000000000043));
#65893=CARTESIAN_POINT('Ctrl Pts',(0.087835924422175,0.718818063572574,
-0.0600000000000051));
#65894=CARTESIAN_POINT('Ctrl Pts',(0.078192029520663,0.720776684620672,
-0.0600000000000053));
#65895=CARTESIAN_POINT('Ctrl Pts',(0.0685016518516216,0.722541197386995,
-0.060000000000002));
#65896=CARTESIAN_POINT('Ctrl Pts',(0.0587699268909895,0.724109135045819,
-0.0600000000000022));
#65897=CARTESIAN_POINT('Ctrl Pts',(0.051744008636474,0.725241123656639,
-0.0600000000000024));
#65898=CARTESIAN_POINT('Ctrl Pts',(0.0446979572491356,0.72627029397537,
-0.0600000000000017));
#65899=CARTESIAN_POINT('Ctrl Pts',(0.0376459184080252,0.72719449158428,
-0.0600000000000016));
#65900=CARTESIAN_POINT('Ctrl Pts',(0.00302545646785632,0.731731640182775,
-0.0600000000000011));
#65901=CARTESIAN_POINT('Ctrl Pts',(-0.031815950771749,0.733755643496836,
-0.0600000000000015));
#65902=CARTESIAN_POINT('Ctrl Pts',(-0.0666351986914192,0.733220747553446,
-0.0600000000000016));
#65903=CARTESIAN_POINT('Ctrl Pts',(-0.0978099748576694,0.73274183826322,
-0.0600000000000017));
#65904=CARTESIAN_POINT('Ctrl Pts',(-0.128967916329204,0.730211415375235,
-0.0600000000000015));
#65905=CARTESIAN_POINT('Ctrl Pts',(-0.159918958605025,0.725709968094987,
-0.0600000000000019));
#65906=CARTESIAN_POINT('Ctrl Pts',(-0.177115326992562,0.72320896845115,
-0.0600000000000022));
#65907=CARTESIAN_POINT('Ctrl Pts',(-0.194247924239629,0.720098917582186,
-0.0600000000000003));
#65908=CARTESIAN_POINT('Ctrl Pts',(-0.211284081588466,0.716389152698896,
-0.0600000000000005));
#65909=CARTESIAN_POINT('Ctrl Pts',(-0.21877637839257,0.714757642786777,
-0.0600000000000005));
#65910=CARTESIAN_POINT('Ctrl Pts',(-0.226252210451876,0.713009546015677,
-0.0600000000000036));
#65911=CARTESIAN_POINT('Ctrl Pts',(-0.233701701874929,0.711147247282136,
-0.0600000000000037));
#65912=CARTESIAN_POINT('Ctrl Pts',(-0.268556898996262,0.702433794809997,
-0.0600000000000039));
#65913=CARTESIAN_POINT('Ctrl Pts',(-0.302694523266425,0.691261318242376,
-0.0599999999999986));
#65914=CARTESIAN_POINT('Ctrl Pts',(-0.335838445624681,0.677768486476775,
-0.0599999999999999));
#65915=CARTESIAN_POINT('Ctrl Pts',(-0.366475589801689,0.665296159644406,
-0.0600000000000011));
#65916=CARTESIAN_POINT('Ctrl Pts',(-0.396264622338141,0.650840433539252,
-0.0600000000000013));
#65917=CARTESIAN_POINT('Ctrl Pts',(-0.424984508158568,0.634471369253308,
-0.0600000000000007));
#65918=CARTESIAN_POINT('Ctrl Pts',(-0.439836175671524,0.626006575841765,
-0.0600000000000003));
#65919=CARTESIAN_POINT('Ctrl Pts',(-0.454401799726264,0.617029523971439,
-0.0600000000000031));
#65920=CARTESIAN_POINT('Ctrl Pts',(-0.46866343319739,0.607559896176671,
-0.060000000000003));
#65921=CARTESIAN_POINT('Ctrl Pts',(-0.476254270714066,0.602519631603962,
-0.060000000000003));
#65922=CARTESIAN_POINT('Ctrl Pts',(-0.483758966532017,0.597339781307538,
-0.0600000000000032));
#65923=CARTESIAN_POINT('Ctrl Pts',(-0.491174642031591,0.592023050064053,
-0.0600000000000034));
#65924=CARTESIAN_POINT('Ctrl Pts',(-0.497227421634385,0.587683458556044,
-0.0600000000000035));
#65925=CARTESIAN_POINT('Ctrl Pts',(-0.503220520759525,0.583252774240972,
-0.0600000000000041));
#65926=CARTESIAN_POINT('Ctrl Pts',(-0.509141502723096,0.57874116345263,
-0.0600000000000041));
#65927=CARTESIAN_POINT('Ctrl Pts',(-0.538044859697743,0.556717671750003,
-0.060000000000004));
#65928=CARTESIAN_POINT('Ctrl Pts',(-0.565299991169042,0.532721355130354,
-0.0600000000000025));
#65929=CARTESIAN_POINT('Ctrl Pts',(-0.590759649941275,0.506978100941496,
-0.0600000000000023));
#65930=CARTESIAN_POINT('Ctrl Pts',(-0.616419524097047,0.481032401167758,
-0.060000000000002));
#65931=CARTESIAN_POINT('Ctrl Pts',(-0.640256514113435,0.453311469631144,
-0.0600000000000016));
#65932=CARTESIAN_POINT('Ctrl Pts',(-0.662093299222365,0.424001632204223,
-0.0600000000000009));
#65933=CARTESIAN_POINT('Ctrl Pts',(-0.675906732853106,0.405460922479556,
-0.0600000000000005));
#65934=CARTESIAN_POINT('Ctrl Pts',(-0.688919204795322,0.386283542748579,
-0.0600000000000007));
#65935=CARTESIAN_POINT('Ctrl Pts',(-0.701077753000027,0.366509473613485,
-0.0600000000000005));
#65936=CARTESIAN_POINT('',(0.7911,-9.68818082805471E-17,-0.0599999999999996));
#65937=CARTESIAN_POINT('Origin',(0.,0.,-0.0599999999999996));
#65938=CARTESIAN_POINT('',(-0.725153241366725,-0.317623382068616,-0.0600000000000044));
#65939=CARTESIAN_POINT('Origin',(0.,0.,-0.0599999999999996));
#65940=CARTESIAN_POINT('Ctrl Pts',(-0.725153241366672,-0.31762338206874,
-0.059999999999999));
#65941=CARTESIAN_POINT('Ctrl Pts',(-0.71567638822314,-0.336030067509267,
-0.0599999999999988));
#65942=CARTESIAN_POINT('Ctrl Pts',(-0.705459356711865,-0.354019774411552,
-0.0599999999999999));
#65943=CARTESIAN_POINT('Ctrl Pts',(-0.69449898909459,-0.371543591325028,
-0.0599999999999991));
#65944=CARTESIAN_POINT('Ctrl Pts',(-0.677442366510842,-0.398814312687398,
-0.059999999999998));
#65945=CARTESIAN_POINT('Ctrl Pts',(-0.658586409729439,-0.42495799055036,
-0.0599999999999969));
#65946=CARTESIAN_POINT('Ctrl Pts',(-0.638101393125394,-0.449852933456938,
-0.0599999999999976));
#65947=CARTESIAN_POINT('Ctrl Pts',(-0.628212892280591,-0.461870188249615,
-0.059999999999998));
#65948=CARTESIAN_POINT('Ctrl Pts',(-0.617944473508911,-0.473596129144332,
-0.0600000000000003));
#65949=CARTESIAN_POINT('Ctrl Pts',(-0.607313831651076,-0.485014974644845,
-0.0600000000000007));
#65950=CARTESIAN_POINT('Ctrl Pts',(-0.60081457747583,-0.491996112781956,
-0.0600000000000009));
#65951=CARTESIAN_POINT('Ctrl Pts',(-0.594186380454014,-0.498855443847342,
-0.0600000000000002));
#65952=CARTESIAN_POINT('Ctrl Pts',(-0.587436138509517,-0.505587758432277,
-0.0600000000000002));
#65953=CARTESIAN_POINT('Ctrl Pts',(-0.562022501970022,-0.530933901183581,
-0.0600000000000004));
#65954=CARTESIAN_POINT('Ctrl Pts',(-0.534870946059782,-0.554493762857957,
-0.0599999999999985));
#65955=CARTESIAN_POINT('Ctrl Pts',(-0.506214094516617,-0.576089885197481,
-0.0599999999999995));
#65956=CARTESIAN_POINT('Ctrl Pts',(-0.488437010443516,-0.589486893654757,
-0.0600000000000001));
#65957=CARTESIAN_POINT('Ctrl Pts',(-0.470080056783044,-0.602127431065171,
-0.0599999999999962));
#65958=CARTESIAN_POINT('Ctrl Pts',(-0.4511951475437,-0.613960201983324,
-0.0599999999999962));
#65959=CARTESIAN_POINT('Ctrl Pts',(-0.444140303534987,-0.618380575518637,
-0.0599999999999961));
#65960=CARTESIAN_POINT('Ctrl Pts',(-0.437018723894153,-0.622683725880098,
-0.0600000000000009));
#65961=CARTESIAN_POINT('Ctrl Pts',(-0.429837497145262,-0.626865226020263,
-0.0600000000000009));
#65962=CARTESIAN_POINT('Ctrl Pts',(-0.425253905882446,-0.629534169388592,
-0.0600000000000009));
#65963=CARTESIAN_POINT('Ctrl Pts',(-0.420645488243079,-0.632153880439322,
-0.0600000000000031));
#65964=CARTESIAN_POINT('Ctrl Pts',(-0.416013022974233,-0.634723838317226,
-0.060000000000003));
#65965=CARTESIAN_POINT('Ctrl Pts',(-0.384772265521933,-0.652055307862434,
-0.0600000000000021));
#65966=CARTESIAN_POINT('Ctrl Pts',(-0.352439280623423,-0.667128030309419,
-0.0599999999999987));
#65967=CARTESIAN_POINT('Ctrl Pts',(-0.319245655087293,-0.679866938257725,
-0.0599999999999985));
#65968=CARTESIAN_POINT('Ctrl Pts',(-0.286427032018807,-0.692461929359391,
-0.0599999999999983));
#65969=CARTESIAN_POINT('Ctrl Pts',(-0.252765977888783,-0.702775719150857,
-0.0599999999999996));
#65970=CARTESIAN_POINT('Ctrl Pts',(-0.21847902697937,-0.710686039402769,
-0.059999999999999));
#65971=CARTESIAN_POINT('Ctrl Pts',(-0.206107665761941,-0.713540228141817,
-0.0599999999999988));
#65972=CARTESIAN_POINT('Ctrl Pts',(-0.193654831169708,-0.716081022922348,
-0.0599999999999994));
#65973=CARTESIAN_POINT('Ctrl Pts',(-0.181130885406342,-0.718300992752236,
-0.0599999999999992));
#65974=CARTESIAN_POINT('Ctrl Pts',(-0.173595035779981,-0.719636782536796,
-0.059999999999999));
#65975=CARTESIAN_POINT('Ctrl Pts',(-0.166041024822709,-0.720854991242619,
-0.0600000000000011));
#65976=CARTESIAN_POINT('Ctrl Pts',(-0.158476926682109,-0.721953909943718,
-0.060000000000001));
#65977=CARTESIAN_POINT('Ctrl Pts',(-0.125718579853494,-0.726713070821577,
-0.0600000000000005));
#65978=CARTESIAN_POINT('Ctrl Pts',(-0.0927368516621256,-0.729244442193755,
-0.0600000000000052));
#65979=CARTESIAN_POINT('Ctrl Pts',(-0.0597155451061104,-0.729466847379534,
-0.0600000000000033));
#65980=CARTESIAN_POINT('Ctrl Pts',(-0.0298340896154985,-0.729668105032634,
-0.0600000000000016));
#65981=CARTESIAN_POINT('Ctrl Pts',(8.04126947938424E-5,-0.727977909840741,
-0.0599999999999993));
#65982=CARTESIAN_POINT('Ctrl Pts',(0.0298429891659583,-0.724431762203439,
-0.0600000000000001));
#65983=CARTESIAN_POINT('Ctrl Pts',(0.0450151293358453,-0.72262403399589,
-0.0600000000000005));
#65984=CARTESIAN_POINT('Ctrl Pts',(0.0601476579444566,-0.720333564472935,
-0.0599999999999992));
#65985=CARTESIAN_POINT('Ctrl Pts',(0.0752148178788815,-0.717562461013743,
-0.0599999999999992));
#65986=CARTESIAN_POINT('Ctrl Pts',(0.0841519166525747,-0.715918778632013,
-0.0599999999999991));
#65987=CARTESIAN_POINT('Ctrl Pts',(0.0930659974908798,-0.714105963589849,
-0.0600000000000014));
#65988=CARTESIAN_POINT('Ctrl Pts',(0.101951481945639,-0.712124184480052,
-0.0600000000000016));
#65989=CARTESIAN_POINT('Ctrl Pts',(0.108774015869091,-0.710602516722462,
-0.0600000000000018));
#65990=CARTESIAN_POINT('Ctrl Pts',(0.115570530759411,-0.708983264219682,
-0.0599999999999967));
#65991=CARTESIAN_POINT('Ctrl Pts',(0.12233784538292,-0.70726743743928,-0.0599999999999969));
#65992=CARTESIAN_POINT('Ctrl Pts',(0.155294287876727,-0.698911457295961,
-0.0599999999999979));
#65993=CARTESIAN_POINT('Ctrl Pts',(0.187566989762046,-0.688267264048053,
-0.0600000000000011));
#65994=CARTESIAN_POINT('Ctrl Pts',(0.218886517124081,-0.675398199752587,
-0.0600000000000005));
#65995=CARTESIAN_POINT('Ctrl Pts',(0.241740156394627,-0.666007733869806,
-0.06));
#65996=CARTESIAN_POINT('Ctrl Pts',(0.264086117884324,-0.655431560122243,
-0.0599999999999987));
#65997=CARTESIAN_POINT('Ctrl Pts',(0.285810299892495,-0.643679437283942,
-0.0599999999999986));
#65998=CARTESIAN_POINT('Ctrl Pts',(0.299989747415091,-0.636008786715737,
-0.0599999999999985));
#65999=CARTESIAN_POINT('Ctrl Pts',(0.313904101961907,-0.627836877170446,
-0.0599999999999994));
#66000=CARTESIAN_POINT('Ctrl Pts',(0.327530462491282,-0.619179691563123,
-0.0599999999999993));
#66001=CARTESIAN_POINT('Ctrl Pts',(0.334428494585131,-0.614797190158366,
-0.0599999999999992));
#66002=CARTESIAN_POINT('Ctrl Pts',(0.341252690027423,-0.610290304047882,
-0.0599999999999995));
#66003=CARTESIAN_POINT('Ctrl Pts',(0.347999856950083,-0.605660967794704,
-0.0599999999999994));
#66004=CARTESIAN_POINT('Ctrl Pts',(0.353764495005457,-0.601705759891582,
-0.0599999999999992));
#66005=CARTESIAN_POINT('Ctrl Pts',(0.359471946468096,-0.59766166929808,
-0.0600000000000004));
#66006=CARTESIAN_POINT('Ctrl Pts',(0.365110271189495,-0.593537654738276,
-0.0600000000000004));
#66007=CARTESIAN_POINT('Ctrl Pts',(0.392009677179333,-0.573862742874626,
-0.0600000000000001));
#66008=CARTESIAN_POINT('Ctrl Pts',(0.417402536256808,-0.552328568843849,
-0.059999999999997));
#66009=CARTESIAN_POINT('Ctrl Pts',(0.441115049422705,-0.529109016476954,
-0.059999999999997));
#66010=CARTESIAN_POINT('Ctrl Pts',(0.464440006753227,-0.506268963024899,
-0.059999999999997));
#66011=CARTESIAN_POINT('Ctrl Pts',(0.486139746646728,-0.481797195771757,
-0.0599999999999998));
#66012=CARTESIAN_POINT('Ctrl Pts',(0.506008214264659,-0.455831110125939,
-0.0599999999999989));
#66013=CARTESIAN_POINT('Ctrl Pts',(0.516926413410576,-0.441562123731379,
-0.0599999999999985));
#66014=CARTESIAN_POINT('Ctrl Pts',(0.527290837420226,-0.426841476968761,
-0.0599999999999988));
#66015=CARTESIAN_POINT('Ctrl Pts',(0.537060862935828,-0.411689834101626,
-0.0599999999999987));
#66016=CARTESIAN_POINT('Ctrl Pts',(-0.29260193430685,0.610169646934268,
-11.9749488707953));
#66017=CARTESIAN_POINT('Ctrl Pts',(-0.39411224040642,0.561491198135562,
-11.9696533379638));
#66018=CARTESIAN_POINT('Ctrl Pts',(-0.572019135180604,0.412886067482696,
-11.9590622723009));
#66019=CARTESIAN_POINT('Ctrl Pts',(-0.700345999063052,0.0876437013347023,
-11.9431756738065));
#66020=CARTESIAN_POINT('Ctrl Pts',(-0.655981217404692,-0.256375724037327,
-11.9272890753121));
#66021=CARTESIAN_POINT('Ctrl Pts',(-0.387452247378358,-0.637512366484492,
-11.9061069439862));
#66022=CARTESIAN_POINT('Ctrl Pts',(0.235314852578195,-0.765023683212307,
-11.879629279829));
#66023=CARTESIAN_POINT('Ctrl Pts',(0.77140418662287,-0.214212144206197,
-11.8478560828401));
#66024=CARTESIAN_POINT('Ctrl Pts',(0.626282581243407,0.404955323743999,
-11.8213784186828));
#66025=CARTESIAN_POINT('Ctrl Pts',(0.238575376523109,0.662775532235479,
-11.800196287357));
#66026=CARTESIAN_POINT('Ctrl Pts',(-0.1078208916813,0.6976941672648,-11.7843096888626));
#66027=CARTESIAN_POINT('Ctrl Pts',(-0.426851047433615,0.560357959801784,
-11.7684230903682));
#66028=CARTESIAN_POINT('Ctrl Pts',(-0.719896296594628,0.196619495603219,
-11.7472409590423));
#66029=CARTESIAN_POINT('Ctrl Pts',(-0.679657526711988,-0.308589625758868,
-11.7260588277165));
#66030=CARTESIAN_POINT('Ctrl Pts',(-0.332712891609252,-0.620107353319397,
-11.7048766963906));
#66031=CARTESIAN_POINT('Ctrl Pts',(0.116413504415669,-0.736688237868005,
-11.6836945650647));
#66032=CARTESIAN_POINT('Ctrl Pts',(0.675171437908528,-0.430783745523332,
-11.6572169009074));
#66033=CARTESIAN_POINT('Ctrl Pts',(0.726297966642536,0.336112054414775,
-11.6254437039186));
#66034=CARTESIAN_POINT('Ctrl Pts',(0.215357505998631,0.71407287292108,-11.5989660397613));
#66035=CARTESIAN_POINT('Ctrl Pts',(-0.247283197394635,0.659606503579982,
-11.5777839084354));
#66036=CARTESIAN_POINT('Ctrl Pts',(-0.533793635826822,0.461976473865101,
-11.5618973099411));
#66037=CARTESIAN_POINT('Ctrl Pts',(-0.688110478507896,0.150777350721831,
-11.5460107114466));
#66038=CARTESIAN_POINT('Ctrl Pts',(-0.675964715110877,-0.316165620402174,
-11.5248285801208));
#66039=CARTESIAN_POINT('Ctrl Pts',(-0.318270223098515,-0.675181839024747,
-11.5036464487949));
#66040=CARTESIAN_POINT('Ctrl Pts',(0.147840292895422,-0.688022737605352,
-11.4824643174691));
#66041=CARTESIAN_POINT('Ctrl Pts',(0.565623962158729,-0.486136361723975,
-11.4612821861432));
#66042=CARTESIAN_POINT('Ctrl Pts',(0.793479716880401,0.108734401743206,
-11.4348045219859));
#66043=CARTESIAN_POINT('Ctrl Pts',(0.335993916742615,0.726352298131389,
-11.4030313249971));
#66044=CARTESIAN_POINT('Ctrl Pts',(-0.298112918637422,0.683671975462962,
-11.3765536608398));
#66045=CARTESIAN_POINT('Ctrl Pts',(-0.615475022766798,0.342666648827597,
-11.3553715295139));
#66046=CARTESIAN_POINT('Ctrl Pts',(-0.705914102226468,0.00656161875215415,
-11.3394849310195));
#66047=CARTESIAN_POINT('Ctrl Pts',(-0.622077616086916,-0.330528871792904,
-11.3235983325252));
#66048=CARTESIAN_POINT('Ctrl Pts',(-0.310543480858139,-0.67856592981927,
-11.3024162011993));
#66049=CARTESIAN_POINT('Ctrl Pts',(0.194497940172004,-0.720650396469946,
-11.2812340698734));
#66050=CARTESIAN_POINT('Ctrl Pts',(0.558075706772724,-0.428699840487657,
-11.2600519385476));
#66051=CARTESIAN_POINT('Ctrl Pts',(0.745814935827746,-0.00437062783121209,
-11.2388698072217));
#66052=CARTESIAN_POINT('Ctrl Pts',(0.534393477883215,0.596537379583458,
-11.2123921430644));
#66053=CARTESIAN_POINT('Ctrl Pts',(-0.21411444420791,0.771125527228726,
-11.1806189460756));
#66054=CARTESIAN_POINT('Ctrl Pts',(-0.669795637756652,0.328104380872136,
-11.1541412819183));
#66055=CARTESIAN_POINT('Ctrl Pts',(-0.690935495823123,-0.137251874422689,
-11.1329591505924));
#66056=CARTESIAN_POINT('Ctrl Pts',(-0.542288925423647,-0.451973998913277,
-11.117072552098));
#66057=CARTESIAN_POINT('Ctrl Pts',(-0.260173180138369,-0.654629522639962,
-11.1011859536036));
#66058=CARTESIAN_POINT('Ctrl Pts',(0.20257790968715,-0.718227794756728,
-11.0800038222778));
#66059=CARTESIAN_POINT('Ctrl Pts',(0.61475932399721,-0.423364401158974,
-11.0588216909519));
#66060=CARTESIAN_POINT('Ctrl Pts',(0.702880058995295,0.0345205795692396,
-11.0376395596261));
#66061=CARTESIAN_POINT('Ctrl Pts',(0.571282631286294,0.479473853373007,
-11.0164574283002));
#66062=CARTESIAN_POINT('Ctrl Pts',(0.0211398831226441,0.800616225032851,
-10.9899797641429));
#66063=CARTESIAN_POINT('Ctrl Pts',(-0.66238604146316,0.449137290861845,
-10.9582065671541));
#66064=CARTESIAN_POINT('Ctrl Pts',(-0.722911249857644,-0.183515683067351,
-10.9317289029968));
#66065=CARTESIAN_POINT('Ctrl Pts',(-0.437774356145965,-0.551890885522362,
-10.9105467716709));
#66066=CARTESIAN_POINT('Ctrl Pts',(-0.120741175465174,-0.695542481001687,
-10.8946601731765));
#66067=CARTESIAN_POINT('Ctrl Pts',(0.225474399042472,-0.667376348810361,
-10.8787735746821));
#66068=CARTESIAN_POINT('Ctrl Pts',(0.619349525511595,-0.416287328540213,
-10.8575914433563));
#66069=CARTESIAN_POINT('Ctrl Pts',(0.7426298818878,0.0752814793781906,-10.8364093120304));
#66070=CARTESIAN_POINT('Ctrl Pts',(0.513381745134516,0.481322377944037,
-10.8152271807046));
#66071=CARTESIAN_POINT('Ctrl Pts',(0.12503781439124,0.735271763261725,-10.7940450493787));
#66072=CARTESIAN_POINT('Ctrl Pts',(-0.502168228339166,0.62390728869839,
-10.7675673852214));
#66073=CARTESIAN_POINT('Ctrl Pts',(-0.79561467114833,-0.0864688904838283,
-10.7357941882326));
#66074=CARTESIAN_POINT('Ctrl Pts',(-0.432196993595701,-0.60785231744993,
-10.7093165240753));
#66075=CARTESIAN_POINT('Ctrl Pts',(0.0236003080504614,-0.704040454719466,
-10.6881343927494));
#66076=CARTESIAN_POINT('Ctrl Pts',(0.358233295234271,-0.608298183883769,
-10.672247794255));
#66077=CARTESIAN_POINT('Ctrl Pts',(0.603882212681613,-0.36270672558111,
-10.6563611957606));
#66078=CARTESIAN_POINT('Ctrl Pts',(0.741547131220323,0.0836470372069074,
-10.6351790644348));
#66079=CARTESIAN_POINT('Ctrl Pts',(0.517292027842344,0.53812210560505,-10.6139969331089));
#66080=CARTESIAN_POINT('Ctrl Pts',(0.0797096438481298,0.699198412773276,
-10.5928148017831));
#66081=CARTESIAN_POINT('Ctrl Pts',(-0.380677283636059,0.641360917581681,
-10.5716326704572));
#66082=CARTESIAN_POINT('Ctrl Pts',(-0.786635906925367,0.150456586362906,
-10.5451550062999));
#66083=CARTESIAN_POINT('Ctrl Pts',(-0.550434349937227,-0.580948879314826,
-10.5133818093111));
#66084=CARTESIAN_POINT('Ctrl Pts',(0.0640780911147829,-0.743083225043802,
-10.4869041451538));
#66085=CARTESIAN_POINT('Ctrl Pts',(0.473750232264011,-0.521335452325531,
-10.4657220138279));
#66086=CARTESIAN_POINT('Ctrl Pts',(0.666825430939749,-0.231736097711846,
-10.4498354153335));
#66087=CARTESIAN_POINT('Ctrl Pts',(0.695072554279996,0.114472878279935,
-10.4339488168391));
#66088=CARTESIAN_POINT('Ctrl Pts',(0.511051301097596,0.5437973356877,-10.4127666855133));
#66089=CARTESIAN_POINT('Ctrl Pts',(0.0459205840941021,0.745021974552772,
-10.3915845541874));
#66090=CARTESIAN_POINT('Ctrl Pts',(-0.39187382810385,0.584522840096347,
-10.3704024228615));
#66091=CARTESIAN_POINT('Ctrl Pts',(-0.705335273549897,0.24240703942756,
-10.3492202915357));
#66092=CARTESIAN_POINT('Ctrl Pts',(-0.696965099795456,-0.394554031928942,
-10.3227426273783));
#66093=CARTESIAN_POINT('Ctrl Pts',(-0.0434573418998398,-0.79911891067786,
-10.2909694303896));
#66094=CARTESIAN_POINT('Ctrl Pts',(0.529876458749172,-0.524890102369867,
-10.2644917662322));
#66095=CARTESIAN_POINT('Ctrl Pts',(0.698575844497316,-0.0906737332777898,
-10.2433096349064));
#66096=CARTESIAN_POINT('Ctrl Pts',(0.658263143903542,0.255043932899648,
-10.227423036412));
#66097=CARTESIAN_POINT('Ctrl Pts',(0.455673622452517,0.537207078672659,
-10.2115364379176));
#66098=CARTESIAN_POINT('Ctrl Pts',(0.0374900855372222,0.745307633223355,
-10.1903543065917));
#66099=CARTESIAN_POINT('Ctrl Pts',(-0.447291532886714,0.597575708356613,
-10.1691721752659));
#66100=CARTESIAN_POINT('Ctrl Pts',(-0.677074909743126,0.191837468559726,
-10.14799004394));
#66101=CARTESIAN_POINT('Ctrl Pts',(-0.694522852254603,-0.271840079042577,
-10.1268079126142));
#66102=CARTESIAN_POINT('Ctrl Pts',(-0.275804889831566,-0.751907505740747,
-10.1003302484568));
#66103=CARTESIAN_POINT('Ctrl Pts',(0.484188776139409,-0.637213310460941,
-10.0685570514681));
#66104=CARTESIAN_POINT('Ctrl Pts',(0.743655850199394,-0.0570496061916968,
-10.0420793873107));
#66105=CARTESIAN_POINT('Ctrl Pts',(0.591145954131398,0.383114078749073,
-10.0208972559849));
#66106=CARTESIAN_POINT('Ctrl Pts',(0.336618815106218,0.62052038455411,-10.0050106574905));
#66107=CARTESIAN_POINT('Ctrl Pts',(-0.000452053710239919,0.704435725401867,
-9.98912405899608));
#66108=CARTESIAN_POINT('Ctrl Pts',(-0.453902103296527,0.592335931104618,
-9.96794192767022));
#66109=CARTESIAN_POINT('Ctrl Pts',(-0.727763581286154,0.165911459410156,
-9.94675979634436));
#66110=CARTESIAN_POINT('Ctrl Pts',(-0.640246728266517,-0.292089326561388,
-9.92557766501851));
#66111=CARTESIAN_POINT('Ctrl Pts',(-0.353382605913268,-0.65679506295015,
-9.90439553369265));
#66112=CARTESIAN_POINT('Ctrl Pts',(0.276533191529025,-0.751639959307012,
-9.87791786953533));
#66113=CARTESIAN_POINT('Ctrl Pts',(0.781545819003339,-0.172237355896938,
-9.84614467254655));
#66114=CARTESIAN_POINT('Ctrl Pts',(0.603738860340227,0.437924730538819,
-9.8196670083892));
#66115=CARTESIAN_POINT('Ctrl Pts',(0.202556190221955,0.674685798149359,
-9.79848487706338));
#66116=CARTESIAN_POINT('Ctrl Pts',(-0.145127604936405,0.690865944026855,
-9.78259827856895));
#66117=CARTESIAN_POINT('Ctrl Pts',(-0.456362724825398,0.536621802543421,
-9.76671168007457));
#66118=CARTESIAN_POINT('Ctrl Pts',(-0.729410114843622,0.157638380537224,
-9.74552954874872));
#66119=CARTESIAN_POINT('Ctrl Pts',(-0.662097903369506,-0.344663326978316,
-9.72434741742285));
#66120=CARTESIAN_POINT('Ctrl Pts',(-0.29890544321878,-0.637093073075865,
-9.70316528609701));
#66121=CARTESIAN_POINT('Ctrl Pts',(0.155832898486876,-0.729366251362731,
-9.68198315477112));
#66122=CARTESIAN_POINT('Ctrl Pts',(0.697347007828662,-0.393878642625726,
-9.65550549061384));
#66123=CARTESIAN_POINT('Ctrl Pts',(0.707185315458073,0.374657848667868,
-9.623732293625));
#66124=CARTESIAN_POINT('Ctrl Pts',(0.176672579446854,0.724614021927542,
-9.59725462946772));
#66125=CARTESIAN_POINT('Ctrl Pts',(-0.282373018168577,0.645364559789301,
-9.57607249814184));
#66126=CARTESIAN_POINT('Ctrl Pts',(-0.557848670468146,0.432622971174229,
-9.56018589964745));
#66127=CARTESIAN_POINT('Ctrl Pts',(-0.695218901859782,0.11358069409847,
-9.54429930115307));
#66128=CARTESIAN_POINT('Ctrl Pts',(-0.657997278472313,-0.352034879206046,
-9.52311716982719));
#66129=CARTESIAN_POINT('Ctrl Pts',(-0.281526301655526,-0.691309904519107,
-9.50193503850135));
#66130=CARTESIAN_POINT('Ctrl Pts',(0.184600760711549,-0.679083652352037,
-9.48075290717548));
#66131=CARTESIAN_POINT('Ctrl Pts',(0.590931414136129,-0.455037454134073,
-9.45957077584963));
#66132=CARTESIAN_POINT('Ctrl Pts',(0.786489778819108,0.151218590977907,
-9.43309311169231));
#66133=CARTESIAN_POINT('Ctrl Pts',(0.296474486791864,0.743358898950881,
-9.40131991470351));
#66134=CARTESIAN_POINT('Ctrl Pts',(-0.334422425230761,0.666663575280057,
-9.3748422505462));
#66135=CARTESIAN_POINT('Ctrl Pts',(-0.633000432686499,0.30909608318511,
-9.35366011922033));
#66136=CARTESIAN_POINT('Ctrl Pts',(-0.705246662148004,-0.0313834328873447,
-9.33777352072594));
#66137=CARTESIAN_POINT('Ctrl Pts',(-0.603416199871352,-0.363481478631069,
-9.32188692223156));
#66138=CARTESIAN_POINT('Ctrl Pts',(-0.273628850822219,-0.694273884466568,
-9.30070479090568));
#66139=CARTESIAN_POINT('Ctrl Pts',(0.23294438000554,-0.709156793970058,
-9.27952265957983));
#66140=CARTESIAN_POINT('Ctrl Pts',(0.580307452228801,-0.398089573632346,
-9.25834052825398));
#66141=CARTESIAN_POINT('Ctrl Pts',(0.744972095404132,0.0357155140929017,
-9.2371583969281));
#66142=CARTESIAN_POINT('Ctrl Pts',(0.501563565304761,0.624393485234313,
-9.2106807327708));
#66143=CARTESIAN_POINT('Ctrl Pts',(-0.255245053230173,0.758504803392499,
-9.17890753578199));
#66144=CARTESIAN_POINT('Ctrl Pts',(-0.68645998202962,0.291635687415495,
-9.15242987162469));
#66145=CARTESIAN_POINT('Ctrl Pts',(-0.682561214906084,-0.174184167844268,
-9.13124774029882));
#66146=CARTESIAN_POINT('Ctrl Pts',(-0.517216387829029,-0.48046329983859,
-9.11536114180443));
#66147=CARTESIAN_POINT('Ctrl Pts',(-0.224617670094119,-0.667665183948138,
-9.09947454331003));
#66148=CARTESIAN_POINT('Ctrl Pts',(0.240882484103758,-0.706303478333916,
-9.07829241198417));
#66149=CARTESIAN_POINT('Ctrl Pts',(0.636622435975274,-0.389715686909015,
-9.05711028065832));
#66150=CARTESIAN_POINT('Ctrl Pts',(0.700009260781494,0.0722432181399054,
-9.03592814933246));
#66151=CARTESIAN_POINT('Ctrl Pts',(0.544690364967499,0.509481527819525,
-9.0147460180066));
#66152=CARTESIAN_POINT('Ctrl Pts',(-0.0219154922400167,0.800595369487078,
-8.98826835384928));
#66153=CARTESIAN_POINT('Ctrl Pts',(-0.685565357771946,0.412891891650819,
-8.95649515686049));
#66154=CARTESIAN_POINT('Ctrl Pts',(-0.712004562954644,-0.22209948994579,
-8.93001749270316));
#66155=CARTESIAN_POINT('Ctrl Pts',(-0.407483346505639,-0.574619229353,-8.90883536137732));
#66156=CARTESIAN_POINT('Ctrl Pts',(-0.0831884995869038,-0.701025996570153,
-8.89294876288291));
#66157=CARTESIAN_POINT('Ctrl Pts',(0.261013149201355,-0.654295064568733,
-8.87706216438852));
#66158=CARTESIAN_POINT('Ctrl Pts',(0.640825685227696,-0.382402165013538,
-8.85588003306267));
#66159=CARTESIAN_POINT('Ctrl Pts',(0.737511168356077,0.11508135887323,-8.8346979017368));
#66160=CARTESIAN_POINT('Ctrl Pts',(0.486773807622215,0.508215808451524,
-8.81351577041096));
#66161=CARTESIAN_POINT('Ctrl Pts',(0.0853438924577135,0.740928769112059,
-8.79233363908507));
#66162=CARTESIAN_POINT('Ctrl Pts',(-0.534971139146889,0.596019391231656,
-8.76585597492778));
#66163=CARTESIAN_POINT('Ctrl Pts',(-0.789818186168672,-0.12909998747171,
-8.73408277793897));
#66164=CARTESIAN_POINT('Ctrl Pts',(-0.398906696132759,-0.630200070519562,
-8.70760511378165));
#66165=CARTESIAN_POINT('Ctrl Pts',(0.061401085864204,-0.701754831174225,
-8.68642298245581));
#66166=CARTESIAN_POINT('Ctrl Pts',(0.390405367007379,-0.588167853373958,
-8.67053638396139));
#66167=CARTESIAN_POINT('Ctrl Pts',(0.622501320628285,-0.329730194842773,
-8.65464978546701));
#66168=CARTESIAN_POINT('Ctrl Pts',(0.735980420215885,0.123376641684858,
-8.63346765414115));
#66169=CARTESIAN_POINT('Ctrl Pts',(0.487626042973425,0.565143596640834,
-8.61228552281528));
#66170=CARTESIAN_POINT('Ctrl Pts',(0.0420197908343311,0.702471625708329,
-8.59110339148945));
#66171=CARTESIAN_POINT('Ctrl Pts',(-0.414593702842348,0.619976678949471,
-8.56992126016356));
#66172=CARTESIAN_POINT('Ctrl Pts',(-0.793584686296887,0.107965643235917,
-8.54344359600627));
#66173=CARTESIAN_POINT('Ctrl Pts',(-0.518418978391269,-0.609689541333719,
-8.51167039901745));
#66174=CARTESIAN_POINT('Ctrl Pts',(0.10391852221122,-0.738565922476695,
-8.48519273486015));
#66175=CARTESIAN_POINT('Ctrl Pts',(0.501082034024498,-0.495122945943268,
-8.46401060353428));
#66176=CARTESIAN_POINT('Ctrl Pts',(0.678315270358112,-0.195566276054168,
-8.44812400503989));
#66177=CARTESIAN_POINT('Ctrl Pts',(0.687916430292161,0.151660411805788,
-8.43223740654549));
#66178=CARTESIAN_POINT('Ctrl Pts',(0.481089349371821,0.570475251501399,
-8.41105527521963));
#66179=CARTESIAN_POINT('Ctrl Pts',(0.00581701517587562,0.746413159680681,
-8.38987314389378));
#66180=CARTESIAN_POINT('Ctrl Pts',(-0.422719610264708,0.562619035266954,
-8.36869101256792));
#66181=CARTESIAN_POINT('Ctrl Pts',(-0.717342918101181,0.204152292977149,
-8.34750888124207));
#66182=CARTESIAN_POINT('Ctrl Pts',(-0.674754780631321,-0.43143854772082,
-8.32103121708474));
#66183=CARTESIAN_POINT('Ctrl Pts',(-0.000450182530976969,-0.800299550983042,
-8.28925802009595));
#66184=CARTESIAN_POINT('Ctrl Pts',(0.55731818268824,-0.495656256237618,
-8.26278035593863));
#66185=CARTESIAN_POINT('Ctrl Pts',(0.70243916327569,-0.0530014935470479,
-8.24159822461277));
#66186=CARTESIAN_POINT('Ctrl Pts',(0.643605972302399,0.290050214182614,
-8.22571162611838));
#66187=CARTESIAN_POINT('Ctrl Pts',(0.426145850537514,0.56091854100633,-8.20982502762398));
#66188=CARTESIAN_POINT('Ctrl Pts',(-0.00261665234877711,0.746245353610373,
-8.18864289629813));
#66189=CARTESIAN_POINT('Ctrl Pts',(-0.478758691882225,0.5726749143775,-8.16746076497226));
#66190=CARTESIAN_POINT('Ctrl Pts',(-0.686405800501428,0.155174497856633,
-8.14627863364641));
#66191=CARTESIAN_POINT('Ctrl Pts',(-0.678910665854216,-0.308770673262746,
-8.12509650232055));
#66192=CARTESIAN_POINT('Ctrl Pts',(-0.234999107869971,-0.765642641017721,
-8.09861883816322));
#66193=CARTESIAN_POINT('Ctrl Pts',(0.517732728409698,-0.610272394838091,
-8.06684564117445));
#66194=CARTESIAN_POINT('Ctrl Pts',(0.745647079045141,-0.0170033706618007,
-8.04036797701711));
#66195=CARTESIAN_POINT('Ctrl Pts',(0.569703324557914,0.414328442674807,
-8.01918584569126));
#66196=CARTESIAN_POINT('Ctrl Pts',(0.302785852511827,0.637713495113113,
-8.00329924719686));
#66197=CARTESIAN_POINT('Ctrl Pts',(-0.0383075228840123,0.70339350954178,
-7.98741264870248));
#66198=CARTESIAN_POINT('Ctrl Pts',(-0.485078126151442,0.567087459025494,
-7.96623051737661));
#66199=CARTESIAN_POINT('Ctrl Pts',(-0.735627971573747,0.126561961300988,
-7.94504838605076));
#66200=CARTESIAN_POINT('Ctrl Pts',(-0.62362478459429,-0.326073880871788,
-7.92386625472489));
#66201=CARTESIAN_POINT('Ctrl Pts',(-0.317576031167041,-0.674836636013439,
-7.90268412339904));
#66202=CARTESIAN_POINT('Ctrl Pts',(0.316526456894863,-0.73569303145392,
-7.87620645924171));
#66203=CARTESIAN_POINT('Ctrl Pts',(0.789672444363271,-0.129988478648325,
-7.84443326225293));
#66204=CARTESIAN_POINT('Ctrl Pts',(0.579332529080104,0.469736630306881,
-7.81795559809561));
#66205=CARTESIAN_POINT('Ctrl Pts',(0.166006120765101,0.684596161463233,
-7.79677346676974));
#66206=CARTESIAN_POINT('Ctrl Pts',(-0.182044780093774,0.68206852468891,
-7.78088686827537));
#66207=CARTESIAN_POINT('Ctrl Pts',(-0.484541134815908,0.511321605495331,
-7.76500026978095));
#66208=CARTESIAN_POINT('Ctrl Pts',(-0.736827533578104,0.118212353059201,
-7.74381813845511));
#66209=CARTESIAN_POINT('Ctrl Pts',(-0.642619076480737,-0.379746185172546,
-7.72263600712924));
#66210=CARTESIAN_POINT('Ctrl Pts',(-0.264236366826861,-0.652235532758837,
-7.70145387580339));
#66211=CARTESIAN_POINT('Ctrl Pts',(0.194803596959322,-0.719937899745148,
-7.68027174447751));
#66212=CARTESIAN_POINT('Ctrl Pts',(0.717506225022208,-0.355834303431602,
-7.65379408032022));
#66213=CARTESIAN_POINT('Ctrl Pts',(0.686029441622246,0.412120345524747,
-7.62202088333141));
#66214=CARTESIAN_POINT('Ctrl Pts',(0.137476787506733,0.733061262105183,
-7.59554321917409));
#66215=CARTESIAN_POINT('Ctrl Pts',(-0.316646643148811,0.629257371672559,
-7.57436108784824));
#66216=CARTESIAN_POINT('Ctrl Pts',(-0.580291571614595,0.402019236161356,
-7.55847448935384));
#66217=CARTESIAN_POINT('Ctrl Pts',(-0.700318083314065,0.0760557542749098,
-7.54258789085945));
#66218=CARTESIAN_POINT('Ctrl Pts',(-0.638128232498241,-0.386886719264509,
-7.52140575953358));
#66219=CARTESIAN_POINT('Ctrl Pts',(-0.243968745432271,-0.705440071063631,
-7.50022362820774));
#66220=CARTESIAN_POINT('Ctrl Pts',(0.22082772031363,-0.66818198545617,-7.47904149688187));
#66221=CARTESIAN_POINT('Ctrl Pts',(0.614531056354557,-0.422623475038358,
-7.45785936555602));
#66222=CARTESIAN_POINT('Ctrl Pts',(0.777226853872599,0.193265755020321,
-7.43138170139868));
#66223=CARTESIAN_POINT('Ctrl Pts',(0.256098235933003,0.758217163825756,
-7.39960850440991));
#66224=CARTESIAN_POINT('Ctrl Pts',(-0.369765439283066,0.64772849328574,
-7.37313084025257));
#66225=CARTESIAN_POINT('Ctrl Pts',(-0.64869644763536,0.27463221815172,-7.35194870892673));
#66226=CARTESIAN_POINT('Ctrl Pts',(-0.70254103328265,-0.0692377850948682,
-7.33606211043233));
#66227=CARTESIAN_POINT('Ctrl Pts',(-0.583010888431519,-0.39538361061797,
-7.32017551193793));
#66228=CARTESIAN_POINT('Ctrl Pts',(-0.235923423345702,-0.707975361839259,
-7.29899338061208));
#66229=CARTESIAN_POINT('Ctrl Pts',(0.270717601992387,-0.695613702123204,
-7.27781124928622));
#66230=CARTESIAN_POINT('Ctrl Pts',(0.600862087662645,-0.366328813167557,
-7.25662911796036));
#66231=CARTESIAN_POINT('Ctrl Pts',(0.741976258067605,0.0756984368513641,
-7.23544698663451));
#66232=CARTESIAN_POINT('Ctrl Pts',(0.467284115457725,0.650445070613317,
-7.20896932247717));
#66233=CARTESIAN_POINT('Ctrl Pts',(-0.295637994600642,0.743691972604572,
-7.1771961254884));
#66234=CARTESIAN_POINT('Ctrl Pts',(-0.701140431554866,0.254324156032159,
-7.15071846133106));
#66235=CARTESIAN_POINT('Ctrl Pts',(-0.672214306820377,-0.210613062576066,
-7.12953633000522));
#66236=CARTESIAN_POINT('Ctrl Pts',(-0.49064907573534,-0.507564044048387,
-7.11364973151081));
#66237=CARTESIAN_POINT('Ctrl Pts',(-0.188413006671554,-0.678771268169181,
-7.09776313301643));
#66238=CARTESIAN_POINT('Ctrl Pts',(0.278490899227765,-0.692337918723144,
-7.07658100169056));
#66239=CARTESIAN_POINT('Ctrl Pts',(0.656645685556425,-0.354940679903258,
-7.05539887036471));
#66240=CARTESIAN_POINT('Ctrl Pts',(0.695115409901483,0.109757071136956,
-7.03421673903885));
#66241=CARTESIAN_POINT('Ctrl Pts',(0.516523923338716,0.538016781798218,
-7.01303460771299));
#66242=CARTESIAN_POINT('Ctrl Pts',(-0.0649075310191635,0.798260763698985,
-6.98655694355567));
#66243=CARTESIAN_POINT('Ctrl Pts',(-0.706763364828739,0.375453219594602,
-6.95478374656687));
#66244=CARTESIAN_POINT('Ctrl Pts',(-0.699040156518267,-0.260041421079877,
-6.92830608240956));
#66245=CARTESIAN_POINT('Ctrl Pts',(-0.376014694915819,-0.595686902348158,
-6.90712395108369));
#66246=CARTESIAN_POINT('Ctrl Pts',(-0.0453954058664428,-0.704483521068271,
-6.89123735258931));
#66247=CARTESIAN_POINT('Ctrl Pts',(0.295797561700471,-0.639322843379747,
-6.8753507540949));
#66248=CARTESIAN_POINT('Ctrl Pts',(0.660449835001555,-0.347411845079441,
-6.85416862276907));
#66249=CARTESIAN_POINT('Ctrl Pts',(0.730261020256401,0.154548648981848,
-6.83298649144319));
#66250=CARTESIAN_POINT('Ctrl Pts',(0.458759075795143,0.533640476468047,
-6.81180436011734));
#66251=CARTESIAN_POINT('Ctrl Pts',(0.0454033235137405,0.744444463400547,
-6.79062222879148));
#66252=CARTESIAN_POINT('Ctrl Pts',(-0.566227963559903,0.566408975674883,
-6.76414456463416));
#66253=CARTESIAN_POINT('Ctrl Pts',(-0.781739097417529,-0.171357980727822,
-6.73237136764536));
#66254=CARTESIAN_POINT('Ctrl Pts',(-0.36446354353643,-0.650726522050533,
-6.70589370348805));
#66255=CARTESIAN_POINT('Ctrl Pts',(0.0990244122389695,-0.697441110221215,
-6.68471157216218));
#66256=CARTESIAN_POINT('Ctrl Pts',(0.421449152886381,-0.566337695957096,
-6.6688249736678));
#66257=CARTESIAN_POINT('Ctrl Pts',(0.639321376606824,-0.295800731727484,
-6.6529383751734));
#66258=CARTESIAN_POINT('Ctrl Pts',(0.72828669883045,0.162749683301894,-6.63175624384754));
#66259=CARTESIAN_POINT('Ctrl Pts',(0.456550800284682,0.590531801388853,
-6.61057411252168));
#66260=CARTESIAN_POINT('Ctrl Pts',(0.00420849966872835,0.703714670097329,
-6.58939198119583));
#66261=CARTESIAN_POINT('Ctrl Pts',(-0.447311932305929,0.59680068373128,
-6.56820984986996));
#66262=CARTESIAN_POINT('Ctrl Pts',(-0.798239973579876,0.0651626776248776,
-6.54173218571265));
#66263=CARTESIAN_POINT('Ctrl Pts',(-0.484905362068866,-0.63666818193181,
-6.50995898872385));
#66264=CARTESIAN_POINT('Ctrl Pts',(0.143458633831261,-0.731914130435804,
-6.48348132456653));
#66265=CARTESIAN_POINT('Ctrl Pts',(0.526965677843967,-0.467479525104637,
-6.46229919324067));
#66266=CARTESIAN_POINT('Ctrl Pts',(0.687844780422188,-0.158831240600472,
-6.44641259474628));
#66267=CARTESIAN_POINT('Ctrl Pts',(0.678772152266887,0.188409603808886,
-6.43052599625188));
#66268=CARTESIAN_POINT('Ctrl Pts',(0.449737145934374,0.595504557883058,
-6.40934386492603));
#66269=CARTESIAN_POINT('Ctrl Pts',(-0.0343035843211689,0.745647019873919,
-6.38816173360018));
#66270=CARTESIAN_POINT('Ctrl Pts',(-0.452343460848582,0.539089431506795,
-6.36697960227431));
#66271=CARTESIAN_POINT('Ctrl Pts',(-0.727278014373636,0.165307092403316,
-6.34579747094845));
#66272=CARTESIAN_POINT('Ctrl Pts',(-0.650593119328475,-0.467075239707729,
-6.31931980679114));
#66273=CARTESIAN_POINT('Ctrl Pts',(0.042556028366106,-0.799168971730803,
-6.28754660980234));
#66274=CARTESIAN_POINT('Ctrl Pts',(0.58315304606446,-0.46498710724797,-6.26106894564502));
#66275=CARTESIAN_POINT('Ctrl Pts',(0.704267131783399,-0.0151800071787377,
-6.23988681431916));
#66276=CARTESIAN_POINT('Ctrl Pts',(0.627100262560229,0.324226811612303,
-6.22400021582477));
#66277=CARTESIAN_POINT('Ctrl Pts',(0.395365052280528,0.582992949678207,
-6.20811361733038));
#66278=CARTESIAN_POINT('Ctrl Pts',(-0.0426668885056882,0.745062854587275,
-6.18693148600451));
#66279=CARTESIAN_POINT('Ctrl Pts',(-0.508936057342763,0.546049163939659,
-6.16574935467866));
#66280=CARTESIAN_POINT('Ctrl Pts',(-0.693643268548973,0.118144784487239,
-6.1445672233528));
#66281=CARTESIAN_POINT('Ctrl Pts',(-0.661592512142315,-0.344999832528101,
-6.12338509202694));
#66282=CARTESIAN_POINT('Ctrl Pts',(-0.192973643036106,-0.776760719460778,
-6.09690742786962));
#66283=CARTESIAN_POINT('Ctrl Pts',(0.548852666849259,-0.58226923395591,
-6.06513423088083));
#66284=CARTESIAN_POINT('Ctrl Pts',(0.786505655010167,0.145511346935457,
-6.03336103389204));
#66285=CARTESIAN_POINT('Ctrl Pts',(0.303954112232331,0.739849035349103,
-6.00158783690326));
#66286=CARTESIAN_POINT('Ctrl Pts',(-0.457122405947255,0.656746386895383,
-5.96981463991447));
#66287=CARTESIAN_POINT('Ctrl Pts',(-0.799835382276926,-0.0293155839405517,
-5.93804144292568));
#66288=CARTESIAN_POINT('Ctrl Pts',(-0.473532610433715,-0.576625011097358,
-5.91156377876836));
#66289=CARTESIAN_POINT('Ctrl Pts',(-0.0268458389766041,-0.703120526676957,
-5.8903816474425));
#66290=CARTESIAN_POINT('Ctrl Pts',(0.429873304441071,-0.610241380137162,
-5.86919951611663));
#66291=CARTESIAN_POINT('Ctrl Pts',(0.72041369487452,-0.194790217664389,
-5.84801738479079));
#66292=CARTESIAN_POINT('Ctrl Pts',(0.651769364779252,0.267190941228426,
-5.82683525346492));
#66293=CARTESIAN_POINT('Ctrl Pts',(0.446117917906169,0.547134871850125,
-5.81094865497054));
#66294=CARTESIAN_POINT('Ctrl Pts',(0.129797396400296,0.692369309990026,
-5.79506205647613));
#66295=CARTESIAN_POINT('Ctrl Pts',(-0.335295695534132,0.666226148989499,
-5.77387992515028));
#66296=CARTESIAN_POINT('Ctrl Pts',(-0.773388981349555,0.205794908719004,
-5.74740226099296));
#66297=CARTESIAN_POINT('Ctrl Pts',(-0.590746005142289,-0.540786319976765,
-5.71562906400416));
#66298=CARTESIAN_POINT('Ctrl Pts',(0.0124024706309206,-0.745725099290851,
-5.68915139984685));
#66299=CARTESIAN_POINT('Ctrl Pts',(0.434685861821545,-0.553425896816594,
-5.66796926852099));
#66300=CARTESIAN_POINT('Ctrl Pts',(0.72270319551117,-0.18672521346106,-5.64678713719512));
#66301=CARTESIAN_POINT('Ctrl Pts',(0.675182030054888,0.317833927049418,
-5.62560500586928));
#66302=CARTESIAN_POINT('Ctrl Pts',(0.323809686428931,0.625601391043243,
-5.6044228745434));
#66303=CARTESIAN_POINT('Ctrl Pts',(-0.0141641249760513,0.705802509565102,
-5.58853627604902));
#66304=CARTESIAN_POINT('Ctrl Pts',(-0.349275640818321,0.611748689208698,
-5.57264967755462));
#66305=CARTESIAN_POINT('Ctrl Pts',(-0.686843080444304,0.290732276842646,
-5.55146754622876));
#66306=CARTESIAN_POINT('Ctrl Pts',(-0.72269141693145,-0.343797469364027,
-5.52498988207144));
#66307=CARTESIAN_POINT('Ctrl Pts',(-0.100182069364385,-0.794604796709607,
-5.49321668508265));
#66308=CARTESIAN_POINT('Ctrl Pts',(0.492200104289347,-0.56035531426314,
-5.46673902092533));
#66309=CARTESIAN_POINT('Ctrl Pts',(0.689575122107159,-0.140421506011553,
-5.44555688959948));
#66310=CARTESIAN_POINT('Ctrl Pts',(0.671714796398658,0.325523691904682,
-5.42437475827361));
#66311=CARTESIAN_POINT('Ctrl Pts',(0.308866959837698,0.679330682531593,
-5.40319262694776));
#66312=CARTESIAN_POINT('Ctrl Pts',(-0.158179798246442,0.686446681763176,
-5.3820104956219));
#66313=CARTESIAN_POINT('Ctrl Pts',(-0.467698735375229,0.528786977202589,
-5.36612389712751));
#66314=CARTESIAN_POINT('Ctrl Pts',(-0.662231679827364,0.240164815655626,
-5.35023729863311));
#66315=CARTESIAN_POINT('Ctrl Pts',(-0.711711733586907,-0.223036071840036,
-5.32905516730725));
#66316=CARTESIAN_POINT('Ctrl Pts',(-0.328270635324783,-0.729875307140714,
-5.30257750314993));
#66317=CARTESIAN_POINT('Ctrl Pts',(0.438031486668258,-0.670493587687057,
-5.27080430616114));
#66318=CARTESIAN_POINT('Ctrl Pts',(0.737897769931333,-0.108470742618401,
-5.24432664200382));
#66319=CARTESIAN_POINT('Ctrl Pts',(0.616490027294739,0.339370143052669,
-5.22314451067796));
#66320=CARTESIAN_POINT('Ctrl Pts',(0.301246298432971,0.682947370072152,
-5.2019623793521));
#66321=CARTESIAN_POINT('Ctrl Pts',(-0.204350803094626,0.717725381973961,
-5.18078024802625));
#66322=CARTESIAN_POINT('Ctrl Pts',(-0.564936112187733,0.420805281242191,
-5.15959811670039));
#66323=CARTESIAN_POINT('Ctrl Pts',(-0.698787211838258,0.100270668202826,
-5.14371151820599));
#66324=CARTESIAN_POINT('Ctrl Pts',(-0.660218179971166,-0.245645865540907,
-5.1278249197116));
#66325=CARTESIAN_POINT('Ctrl Pts',(-0.398077205723047,-0.630724360863014,
-5.10664278838574));
#66326=CARTESIAN_POINT('Ctrl Pts',(0.222281684997194,-0.768811047320993,
-5.08016512422842));
#66327=CARTESIAN_POINT('Ctrl Pts',(0.767909224957921,-0.227483310747878,
-5.04839192723964));
#66328=CARTESIAN_POINT('Ctrl Pts',(0.632637701696453,0.39500450537932,-5.0219142630823));
#66329=CARTESIAN_POINT('Ctrl Pts',(0.250190952797296,0.657751119258226,
-5.00073213175645));
#66330=CARTESIAN_POINT('Ctrl Pts',(-0.212500472627088,0.715548734708769,
-4.97955000043058));
#66331=CARTESIAN_POINT('Ctrl Pts',(-0.620375570452808,0.414756707287463,
-4.95836786910474));
#66332=CARTESIAN_POINT('Ctrl Pts',(-0.702998434927052,-0.0449788401932196,
-4.93718573777888));
#66333=CARTESIAN_POINT('Ctrl Pts',(-0.597519655454011,-0.375936212244599,
-4.92129913928448));
#66334=CARTESIAN_POINT('Ctrl Pts',(-0.344192787318138,-0.61462286125708,
-4.90541254079009));
#66335=CARTESIAN_POINT('Ctrl Pts',(0.104890152807889,-0.738428559135105,
-4.88423040946423));
#66336=CARTESIAN_POINT('Ctrl Pts',(0.66711275320734,-0.442086132417752,
-4.85775274530691));
#66337=CARTESIAN_POINT('Ctrl Pts',(0.732555231440372,0.323722207044275,
-4.82597954831811));
#66338=CARTESIAN_POINT('Ctrl Pts',(0.226483522681462,0.710608355447316,
-4.7995018841608));
#66339=CARTESIAN_POINT('Ctrl Pts',(-0.235103534183009,0.66329358202965,
-4.77831975283493));
#66340=CARTESIAN_POINT('Ctrl Pts',(-0.6251781158456,0.407821978414359,-4.75713762150909));
#66341=CARTESIAN_POINT('Ctrl Pts',(-0.741338321875117,-0.0854778753477755,
-4.73595549018322));
#66342=CARTESIAN_POINT('Ctrl Pts',(-0.506701789827963,-0.489370199092825,
-4.71477335885737));
#66343=CARTESIAN_POINT('Ctrl Pts',(-0.212060776109364,-0.673340925212919,
-4.69888676036297));
#66344=CARTESIAN_POINT('Ctrl Pts',(0.13553701687756,-0.691273935193279,
-4.68300016186857));
#66345=CARTESIAN_POINT('Ctrl Pts',(0.557969828113902,-0.494922571739213,
-4.66181803054273));
#66346=CARTESIAN_POINT('Ctrl Pts',(0.794652742927993,0.0949030669946144,
-4.63534036638539));
#66347=CARTESIAN_POINT('Ctrl Pts',(0.348784514783706,0.720959497261372,
-4.6035671693966));
#66348=CARTESIAN_POINT('Ctrl Pts',(-0.287390379613016,0.68823381970347,
-4.57708950523929));
#66349=CARTESIAN_POINT('Ctrl Pts',(-0.608578462087337,0.353361434271592,
-4.55590737391342));
#66350=CARTESIAN_POINT('Ctrl Pts',(-0.740509564330208,-0.0938724014049983,
-4.53472524258757));
#66351=CARTESIAN_POINT('Ctrl Pts',(-0.509706951025825,-0.545057610469336,
-4.51354311126171));
#66352=CARTESIAN_POINT('Ctrl Pts',(-0.0694084667398682,-0.701008102891709,
-4.49236097993585));
#66353=CARTESIAN_POINT('Ctrl Pts',(0.274258103338072,-0.650492326691175,
-4.47647438144146));
#66354=CARTESIAN_POINT('Ctrl Pts',(0.550802926396446,-0.439142428711666,
-4.46058778294706));
#66355=CARTESIAN_POINT('Ctrl Pts',(0.745668804766385,-0.0160223188298255,
-4.4394056516212));
#66356=CARTESIAN_POINT('Ctrl Pts',(0.544241292482002,0.586754624630679,
-4.41292798746388));
#66357=CARTESIAN_POINT('Ctrl Pts',(-0.200874523336002,0.775295208497259,
-4.3811547904751));
#66358=CARTESIAN_POINT('Ctrl Pts',(-0.664576138776499,0.338522638307489,
-4.35467712631776));
#66359=CARTESIAN_POINT('Ctrl Pts',(-0.69260229547609,-0.124635901923627,
-4.33349499499192));
#66360=CARTESIAN_POINT('Ctrl Pts',(-0.503641062853606,-0.550919342933017,
-4.31231286366604));
#66361=CARTESIAN_POINT('Ctrl Pts',(-0.0356495923251104,-0.745397934811761,
-4.29113073234021));
#66362=CARTESIAN_POINT('Ctrl Pts',(0.400896797976255,-0.579233677324962,
-4.26994860101433));
#66363=CARTESIAN_POINT('Ctrl Pts',(0.630134791455414,-0.318257629803494,
-4.25406200251995));
#66364=CARTESIAN_POINT('Ctrl Pts',(0.704096847355287,0.0218532827285811,
-4.23817540402554));
#66365=CARTESIAN_POINT('Ctrl Pts',(0.578714001944864,0.47049844320186,-4.21699327269969));
#66366=CARTESIAN_POINT('Ctrl Pts',(0.0349786870852126,0.799534905690655,
-4.19051560854237));
#66367=CARTESIAN_POINT('Ctrl Pts',(-0.65499394863327,0.460886278487515,
-4.15874241155358));
#66368=CARTESIAN_POINT('Ctrl Pts',(-0.725677279864578,-0.172196127616421,
-4.13226474739626));
#66369=CARTESIAN_POINT('Ctrl Pts',(-0.447211755898116,-0.54335411393822,
-4.1110826160704));
#66370=CARTESIAN_POINT('Ctrl Pts',(-0.027231621354319,-0.745938926057937,
-4.08990048474455));
#66371=CARTESIAN_POINT('Ctrl Pts',(0.455363367272391,-0.591213310405756,
-4.06871835341868));
#66372=CARTESIAN_POINT('Ctrl Pts',(0.680528182180706,-0.181965075860278,
-4.04753622209283));
#66373=CARTESIAN_POINT('Ctrl Pts',(0.686307798878026,0.165346241353982,
-4.03164962359843));
#66374=CARTESIAN_POINT('Ctrl Pts',(0.522509375349723,0.472455171517164,
-4.01576302510404));
#66375=CARTESIAN_POINT('Ctrl Pts',(0.136512190381233,0.733241503857858,
-3.99458089377818));
#66376=CARTESIAN_POINT('Ctrl Pts',(-0.490920424353534,0.632041700301898,
-3.96810322962086));
#66377=CARTESIAN_POINT('Ctrl Pts',(-0.797586221486274,-0.072728630810176,
-3.93633003263207));
#66378=CARTESIAN_POINT('Ctrl Pts',(-0.441632977912428,-0.601015252466975,
-3.90985236847475));
#66379=CARTESIAN_POINT('Ctrl Pts',(0.0108809088601417,-0.703643129412517,
-3.88867023714889));
#66380=CARTESIAN_POINT('Ctrl Pts',(0.462129679432592,-0.586176255061214,
-3.86748810582303));
#66381=CARTESIAN_POINT('Ctrl Pts',(0.729797145596839,-0.15583677657501,
-3.84630597449717));
#66382=CARTESIAN_POINT('Ctrl Pts',(0.636487863470664,0.301849457891777,
-3.82512384317132));
#66383=CARTESIAN_POINT('Ctrl Pts',(0.416060211528914,0.570308403158517,
-3.80923724467692));
#66384=CARTESIAN_POINT('Ctrl Pts',(0.0924068473382293,0.698348703003505,
-3.79335064618252));
#66385=CARTESIAN_POINT('Ctrl Pts',(-0.370617326288914,0.647241437607997,
-3.77216851485667));
#66386=CARTESIAN_POINT('Ctrl Pts',(-0.783328765084108,0.163937853346245,
-3.74569085069934));
#66387=CARTESIAN_POINT('Ctrl Pts',(-0.560831837890227,-0.571752467465549,
-3.71391765371057));
#66388=CARTESIAN_POINT('Ctrl Pts',(0.0524600799429356,-0.743980484213214,
-3.68743998955323));
#66389=CARTESIAN_POINT('Ctrl Pts',(0.463798413511565,-0.529266548509558,
-3.66625785822738));
#66390=CARTESIAN_POINT('Ctrl Pts',(0.731693616604151,-0.147617390678711,
-3.64507572690151));
#66391=CARTESIAN_POINT('Ctrl Pts',(0.65712599706795,0.353658590496596,-3.62389359557566));
#66392=CARTESIAN_POINT('Ctrl Pts',(0.289722226326614,0.642098845309166,
-3.6027114642498));
#66393=CARTESIAN_POINT('Ctrl Pts',(-0.0520732543285767,0.704021413391895,
-3.58682486575541));
#66394=CARTESIAN_POINT('Ctrl Pts',(-0.381646074532144,0.592094764557056,
-3.57093826726101));
#66395=CARTESIAN_POINT('Ctrl Pts',(-0.7014744353342,0.253401455550246,-3.54975613593516));
#66396=CARTESIAN_POINT('Ctrl Pts',(-0.703171557501552,-0.382137847757598,
-3.52327847177783));
#66397=CARTESIAN_POINT('Ctrl Pts',(-0.0573355312236082,-0.798840329041782,
-3.49150527478905));
#66398=CARTESIAN_POINT('Ctrl Pts',(0.521602160227078,-0.533094932750431,
-3.46502761063172));
#66399=CARTESIAN_POINT('Ctrl Pts',(0.696124873969488,-0.103161075934814,
-3.44384547930587));
#66400=CARTESIAN_POINT('Ctrl Pts',(0.653250630478223,0.361151016044349,
-3.42266334798001));
#66401=CARTESIAN_POINT('Ctrl Pts',(0.271913654699282,0.69494743617245,-3.40148121665415));
#66402=CARTESIAN_POINT('Ctrl Pts',(-0.194840623075141,0.676954228271529,
-3.38029908532829));
#66403=CARTESIAN_POINT('Ctrl Pts',(-0.495439723982,0.50288890843937,-3.36441248683389));
#66404=CARTESIAN_POINT('Ctrl Pts',(-0.674181113544814,0.204229680901535,
-3.3485258883395));
#66405=CARTESIAN_POINT('Ctrl Pts',(-0.698697418738935,-0.260960913069297,
-3.32734375701365));
#66406=CARTESIAN_POINT('Ctrl Pts',(-0.28857304180409,-0.746461769625146,
-3.30086609285632));
#66407=CARTESIAN_POINT('Ctrl Pts',(0.473430607192205,-0.645985057580972,
-3.26909289586753));
#66408=CARTESIAN_POINT('Ctrl Pts',(0.742660672680755,-0.0686596397537776,
-3.24261523171021));
#66409=CARTESIAN_POINT('Ctrl Pts',(0.597361558428951,0.372009699145598,
-3.22143310038435));
#66410=CARTESIAN_POINT('Ctrl Pts',(0.264109646042611,0.698149366165507,
-3.2002509690585));
#66411=CARTESIAN_POINT('Ctrl Pts',(-0.242625816165684,0.705706516892486,
-3.17906883773263));
#66412=CARTESIAN_POINT('Ctrl Pts',(-0.586733693445035,0.38983774644249,
-3.15788670640678));
#66413=CARTESIAN_POINT('Ctrl Pts',(-0.703165961016561,0.0625732019186072,
-3.14200010791238));
#66414=CARTESIAN_POINT('Ctrl Pts',(-0.646063232064753,-0.280770790139778,
-3.12611350941799));
#66415=CARTESIAN_POINT('Ctrl Pts',(-0.363607076602154,-0.651205478284122,
-3.10493137809214));
#66416=CARTESIAN_POINT('Ctrl Pts',(0.263276112884758,-0.755754763367232,
-3.0784537139348));
#66417=CARTESIAN_POINT('Ctrl Pts',(0.779024453182575,-0.18588742772943,
-3.04668051694603));
#66418=CARTESIAN_POINT('Ctrl Pts',(0.610496128531625,0.428431439002367,
-3.0202028527887));
#66419=CARTESIAN_POINT('Ctrl Pts',(0.214482113777081,0.670245828496365,
-2.99902072146284));
#66420=CARTESIAN_POINT('Ctrl Pts',(-0.250646737033531,0.703095054615309,
-2.97783859013698));
#66421=CARTESIAN_POINT('Ctrl Pts',(-0.64176799247962,0.380818616250913,
-2.95665645881112));
#66422=CARTESIAN_POINT('Ctrl Pts',(-0.699565442495169,-0.0826927278637582,
-2.93547432748527));
#66423=CARTESIAN_POINT('Ctrl Pts',(-0.576453551727282,-0.407503468735792,
-2.91958772899087));
#66424=CARTESIAN_POINT('Ctrl Pts',(-0.310665810973606,-0.632231516387613,
-2.90370113049648));
#66425=CARTESIAN_POINT('Ctrl Pts',(0.144421469649071,-0.731724757136735,
-2.88251899917062));
#66426=CARTESIAN_POINT('Ctrl Pts',(0.689906312612689,-0.405596910472863,
-2.85604133501329));
#66427=CARTESIAN_POINT('Ctrl Pts',(0.714099960658798,0.362621677001496,
-2.82426813802451));
#66428=CARTESIAN_POINT('Ctrl Pts',(0.187968412483645,0.721752656237666,
-2.79779047386719));
#66429=CARTESIAN_POINT('Ctrl Pts',(-0.270408963645806,0.649700731204041,
-2.77660834254133));
#66430=CARTESIAN_POINT('Ctrl Pts',(-0.646190928271226,0.373635821128039,
-2.75542621121547));
#66431=CARTESIAN_POINT('Ctrl Pts',(-0.735673524021166,-0.125193612891662,
-2.73424407988961));
#66432=CARTESIAN_POINT('Ctrl Pts',(-0.479671017962049,-0.51589302195539,
-2.71306194856376));
#66433=CARTESIAN_POINT('Ctrl Pts',(-0.17556924533772,-0.683764004918535,
-2.69717535006935));
#66434=CARTESIAN_POINT('Ctrl Pts',(0.172489975910581,-0.682991321051767,
-2.68128875157497));
#66435=CARTESIAN_POINT('Ctrl Pts',(0.583760512301853,-0.464222301682604,
-2.6601066202491));
#66436=CARTESIAN_POINT('Ctrl Pts',(0.78840439834167,0.137470282764965,-2.63362895609179));
#66437=CARTESIAN_POINT('Ctrl Pts',(0.309536410753203,0.738661251767208,
-2.601855759103));
#66438=CARTESIAN_POINT('Ctrl Pts',(-0.323960533014889,0.671795053514425,
-2.57537809494567));
#66439=CARTESIAN_POINT('Ctrl Pts',(-0.626688571274547,0.320146032898944,
-2.55419596361981));
#66440=CARTESIAN_POINT('Ctrl Pts',(-0.734394845236606,-0.133531471571163,
-2.53301383229396));
#66441=CARTESIAN_POINT('Ctrl Pts',(-0.47967921519751,-0.571661460273545,
-2.51183170096809));
#66442=CARTESIAN_POINT('Ctrl Pts',(-0.0316362470218281,-0.703725119240024,
-2.49064956964224));
#66443=CARTESIAN_POINT('Ctrl Pts',(0.308819018868513,-0.634813821459323,
-2.47476297114784));
#66444=CARTESIAN_POINT('Ctrl Pts',(0.573606362075548,-0.408907908713105,
-2.45887637265346));
#66445=CARTESIAN_POINT('Ctrl Pts',(0.745452333195922,0.0240728069648603,
-2.43769424132759));
#66446=CARTESIAN_POINT('Ctrl Pts',(0.511922871354516,0.615154084561029,
-2.41121657717027));
#66447=CARTESIAN_POINT('Ctrl Pts',(-0.242248341456588,0.763379967975192,
-2.37944338018148));
#66448=CARTESIAN_POINT('Ctrl Pts',(-0.681807898729322,0.302319384274405,
-2.35296571602416));
#66449=CARTESIAN_POINT('Ctrl Pts',(-0.684903583824367,-0.161675998873061,
-2.3317835846983));
#66450=CARTESIAN_POINT('Ctrl Pts',(-0.473307084952599,-0.57718874377774,
-2.31060145337244));
#66451=CARTESIAN_POINT('Ctrl Pts',(0.0044593387890197,-0.746236617268379,
-2.28941932204658));
#66452=CARTESIAN_POINT('Ctrl Pts',(0.431445304074627,-0.5568526242795,-2.26823719072073));
#66453=CARTESIAN_POINT('Ctrl Pts',(0.646327285527458,-0.283934524694336,
-2.25235059222633));
#66454=CARTESIAN_POINT('Ctrl Pts',(0.701905026833796,0.0596596155461771,
-2.23646399373194));
#66455=CARTESIAN_POINT('Ctrl Pts',(0.552593332470904,0.500918446467205,
-2.21528186240608));
#66456=CARTESIAN_POINT('Ctrl Pts',(-0.00803857589287147,0.800259305016558,
-2.18880419824876));
#66457=CARTESIAN_POINT('Ctrl Pts',(-0.678815333020211,0.42502115018071,
-2.15703100125997));
#66458=CARTESIAN_POINT('Ctrl Pts',(-0.715374904833764,-0.210944936919148,
-2.13055333710265));
#66459=CARTESIAN_POINT('Ctrl Pts',(-0.417365872073619,-0.566601956028473,
-2.10937120577679));
#66460=CARTESIAN_POINT('Ctrl Pts',(0.0128942183109048,-0.74632444804134,
-2.08818907445093));
#66461=CARTESIAN_POINT('Ctrl Pts',(0.486476949341432,-0.565887932734067,
-2.06700694312507));
#66462=CARTESIAN_POINT('Ctrl Pts',(0.689323544065248,-0.145130793329111,
-2.04582481179921));
#66463=CARTESIAN_POINT('Ctrl Pts',(0.676430423898524,0.201989247127572,
-2.02993821330482));
#66464=CARTESIAN_POINT('Ctrl Pts',(0.496364768725477,0.499851930865303,
-2.01405161481042));
#66465=CARTESIAN_POINT('Ctrl Pts',(0.0969107931718748,0.739518072307371,
-1.99286948348457));
#66466=CARTESIAN_POINT('Ctrl Pts',(-0.524176728798627,0.604746501398676,
-1.96639181932724));
#66467=CARTESIAN_POINT('Ctrl Pts',(-0.792525284190483,-0.115485533133239,
-1.93461862233846));
#66468=CARTESIAN_POINT('Ctrl Pts',(-0.408696466689488,-0.62387997162377,
-1.90814095818113));
#66469=CARTESIAN_POINT('Ctrl Pts',(0.0486787143220458,-0.702041615945249,
-1.88695882685528));
#66470=CARTESIAN_POINT('Ctrl Pts',(0.492962794513711,-0.560494536846958,
-1.86577669552942));
#66471=CARTESIAN_POINT('Ctrl Pts',(0.737117187516088,-0.116392553554602,
-1.84459456420356));
#66472=CARTESIAN_POINT('Ctrl Pts',(0.619346845481977,0.335617908590315,
-1.8234124328777));
#66473=CARTESIAN_POINT('Ctrl Pts',(0.384810828458858,0.591843223017294,
-1.80752583438331));
#66474=CARTESIAN_POINT('Ctrl Pts',(0.0547443097277555,0.702305486931504,
-1.79163923588892));
#66475=CARTESIAN_POINT('Ctrl Pts',(-0.404864299349843,0.626389320003439,
-1.77045710456306));
#66476=CARTESIAN_POINT('Ctrl Pts',(-0.791006801773371,0.121605154151588,
-1.74397944040573));
#66477=CARTESIAN_POINT('Ctrl Pts',(-0.529295653645387,-0.601065175730866,
-1.71220624341695));
#66478=CARTESIAN_POINT('Ctrl Pts',(0.0923655176653327,-0.740086232829771,
-1.68572857925962));
#66479=CARTESIAN_POINT('Ctrl Pts',(0.491570810089264,-0.5035773887053,-1.66454644793377));
#66480=CARTESIAN_POINT('Ctrl Pts',(0.738569211247283,-0.10808312915354,
-1.64336431660791));
#66481=CARTESIAN_POINT('Ctrl Pts',(0.637170952451161,0.388461261913037,
-1.62218218528205));
#66482=CARTESIAN_POINT('Ctrl Pts',(0.254797411454479,0.656740568787333,
-1.60100005395619));
#66483=CARTESIAN_POINT('Ctrl Pts',(-0.0898318649340317,0.700205691474415,
-1.5851134554618));
#66484=CARTESIAN_POINT('Ctrl Pts',(-0.412913548481974,0.570729653953337,
-1.56922685696741));
#66485=CARTESIAN_POINT('Ctrl Pts',(-0.714078494834342,0.215338302021576,
-1.54804472564154));
#66486=CARTESIAN_POINT('Ctrl Pts',(-0.68161951116076,-0.419373837969105,
-1.52156706148423));
#66487=CARTESIAN_POINT('Ctrl Pts',(-0.0143232884913037,-0.800767180802928,
-1.48979386449544));
#66488=CARTESIAN_POINT('Ctrl Pts',(0.549496765312817,-0.504293888311659,
-1.46331620033811));
#66489=CARTESIAN_POINT('Ctrl Pts',(0.700662799746577,-0.0656025060371282,
-1.44213406901226));
#66490=CARTESIAN_POINT('Ctrl Pts',(0.632898545584985,0.395734599961226,
-1.4209519376864));
#66491=CARTESIAN_POINT('Ctrl Pts',(0.234174509286621,0.708555766228003,
-1.39976980636054));
#66492=CARTESIAN_POINT('Ctrl Pts',(-0.230938351402798,0.665505351914144,
-1.37858767503468));
#66493=CARTESIAN_POINT('Ctrl Pts',(-0.521748873394984,0.475537472174135,
-1.36270107654029));
#66494=CARTESIAN_POINT('Ctrl Pts',(-0.684182138924209,0.167704314788749,
-1.34681447804589));
#66495=CARTESIAN_POINT('Ctrl Pts',(-0.683663842477407,-0.298131567586256,
-1.32563234672004));
#66496=CARTESIAN_POINT('Ctrl Pts',(-0.248041461525952,-0.760890929984079,
-1.29915468256271));
#66497=CARTESIAN_POINT('Ctrl Pts',(0.507461495749466,-0.619609606749274,
-1.26738148557393));
#66498=CARTESIAN_POINT('Ctrl Pts',(0.74527725860231,-0.0286501079923499,
-1.2409038214166));
#66499=CARTESIAN_POINT('Ctrl Pts',(0.576506692556375,0.403574133443626,
-1.21972169009074));
#66500=CARTESIAN_POINT('Ctrl Pts',(0.226209707001196,0.711333684755956,
-1.19853955876488));
#66501=CARTESIAN_POINT('Ctrl Pts',(-0.280199631649522,0.691648133864366,
-1.17735742743902));
#66502=CARTESIAN_POINT('Ctrl Pts',(-0.606835592617558,0.35774356613014,
-1.15617529611317));
#66503=CARTESIAN_POINT('Ctrl Pts',(-0.70551253454806,0.0246948967655601,
-1.14028869761877));
#66504=CARTESIAN_POINT('Ctrl Pts',(-0.630041137511382,-0.315084276765811,
-1.12440209912438));
#66505=CARTESIAN_POINT('Ctrl Pts',(-0.328086109575231,-0.669804587776323,
-1.10321996779852));
#66506=CARTESIAN_POINT('Ctrl Pts',(0.303509663064016,-0.740514320182075,
-1.0767423036412));
#66507=CARTESIAN_POINT('Ctrl Pts',(0.787888271911223,-0.143754323166431,
-1.04496910665241));
#66508=CARTESIAN_POINT('Ctrl Pts',(0.586590198965058,0.460620189913425,
-1.01849144249509));
#66509=CARTESIAN_POINT('Ctrl Pts',(0.178153413511559,0.680803502488938,
-0.99730931116923));
#66510=CARTESIAN_POINT('Ctrl Pts',(-0.288068623095297,0.688609403797382,
-0.976127179843373));
#66511=CARTESIAN_POINT('Ctrl Pts',(-0.661305681260653,0.345779945321747,
-0.954945048517514));
#66512=CARTESIAN_POINT('Ctrl Pts',(-0.694110680048501,-0.120167630490676,
-0.933762917191655));
#66513=CARTESIAN_POINT('Ctrl Pts',(-0.553721475905218,-0.437893025123882,
-0.917876318697262));
#66514=CARTESIAN_POINT('Ctrl Pts',(-0.276240998940245,-0.648012999040435,
-0.901989720202866));
#66515=CARTESIAN_POINT('Ctrl Pts',(0.18353540309995,-0.722906243515896,
-0.880807588877012));
#66516=CARTESIAN_POINT('Ctrl Pts',(0.710706017243741,-0.367935498444747,
-0.854329924719684));
#66517=CARTESIAN_POINT('Ctrl Pts',(0.693580914570762,0.4004731568877,-0.8225567277309));
#66518=CARTESIAN_POINT('Ctrl Pts',(0.148910066612057,0.730811065154998,
-0.796079063573575));
#66519=CARTESIAN_POINT('Ctrl Pts',(-0.304932901189276,0.634230221210176,
-0.774896932247717));
#66520=CARTESIAN_POINT('Ctrl Pts',(-0.665336225024664,0.338369842529393,
-0.75371480092186));
#66521=CARTESIAN_POINT('Ctrl Pts',(-0.727882602416646,-0.164547536335721,
-0.732532669595999));
#66522=CARTESIAN_POINT('Ctrl Pts',(-0.451253979159214,-0.540924894803379,
-0.711350538270144));
#66523=CARTESIAN_POINT('Ctrl Pts',(-0.138570312837484,-0.69221098153884,
-0.695463939775748));
#66524=CARTESIAN_POINT('Ctrl Pts',(0.208944432324475,-0.672734836372497,
-0.679577341281356));
#66525=CARTESIAN_POINT('Ctrl Pts',(0.607864107453516,-0.432180412746452,
-0.658395209955497));
#66526=CARTESIAN_POINT('Ctrl Pts',(0.77987753494969,0.179640205882728,-0.631917545798173));
#66527=CARTESIAN_POINT('Ctrl Pts',(0.269393736650696,0.754228245212569,
-0.600144348809387));
#66528=CARTESIAN_POINT('Ctrl Pts',(-0.359594431187155,0.653414779307557,
-0.573666684652064));
#66529=CARTESIAN_POINT('Ctrl Pts',(-0.642987523708695,0.28600539159311,
-0.552484553326205));
#66530=CARTESIAN_POINT('Ctrl Pts',(-0.726157707116663,-0.172804615259813,
-0.531302422000348));
#66531=CARTESIAN_POINT('Ctrl Pts',(-0.448265169876774,-0.596613218990799,
-0.510120290674488));
#66532=CARTESIAN_POINT('Ctrl Pts',(0.00622737937602623,-0.704408304798551,
-0.488938159348631));
#66533=CARTESIAN_POINT('Ctrl Pts',(0.342487484376452,-0.61730076227034,
-0.473051560854236));
#66534=CARTESIAN_POINT('Ctrl Pts',(0.594751965918543,-0.377491481115471,
-0.457164962359842));
#66535=CARTESIAN_POINT('Ctrl Pts',(0.743081667418538,0.0640980403615866,
-0.435982831033984));
#66536=CARTESIAN_POINT('Ctrl Pts',(0.478124579859611,0.641776390658052,
-0.409505166876661));
#66537=CARTESIAN_POINT('Ctrl Pts',(-0.282921364094237,0.749257370810349,
-0.377731969887874));
#66538=CARTESIAN_POINT('Ctrl Pts',(-0.697070363894654,0.265244362057293,
-0.351254305730551));
#66539=CARTESIAN_POINT('Ctrl Pts',(-0.675223937332315,-0.198251437163076,
-0.330072174404692));
#66540=CARTESIAN_POINT('Ctrl Pts',(-0.441609192873322,-0.601783375902012,
-0.308890043078835));
#66541=CARTESIAN_POINT('Ctrl Pts',(0.0445634358699717,-0.744932214423158,
-0.287707911752975));
#66542=CARTESIAN_POINT('Ctrl Pts',(0.460736965378437,-0.532845482801779,
-0.266525780427117));
#66543=CARTESIAN_POINT('Ctrl Pts',(0.660672578510412,-0.248825721585754,
-0.250639181932725));
#66544=CARTESIAN_POINT('Ctrl Pts',(0.697646902447653,0.0973571564825142,
-0.234752583438329));
#66545=CARTESIAN_POINT('Ctrl Pts',(0.524957262296379,0.529753299715826,
-0.213570452112473));
#66546=CARTESIAN_POINT('Ctrl Pts',(-0.0512014684653643,0.798955362640304,
-0.187092787955149));
#66547=CARTESIAN_POINT('Ctrl Pts',(-0.700379789122524,0.387430595988897,
-0.155319590966363));
#66548=CARTESIAN_POINT('Ctrl Pts',(-0.703501109104381,-0.248248768190496,
-0.128841926809038));
#66549=CARTESIAN_POINT('Ctrl Pts',(-0.385645525478233,-0.58933640490133,
-0.107659795483182));
#66550=CARTESIAN_POINT('Ctrl Pts',(-0.0580733210265062,-0.703415543027182,
-0.0917731969887855));
#66551=CARTESIAN_POINT('Ctrl Pts',(0.286592368567594,-0.644628272737791,
-0.0758865984943943));
#66552=CARTESIAN_POINT('Ctrl Pts',(0.468570466391673,-0.501037465313089,
-0.065295532831463));
#66553=CARTESIAN_POINT('Ctrl Pts',(0.537060862935828,-0.411689834101626,
-0.0599999999999987));
#66554=CARTESIAN_POINT('Ctrl Pts',(-0.309090610374417,0.644553868208713,
-11.9529325805302));
#66555=CARTESIAN_POINT('Ctrl Pts',(-0.416321215482797,0.593132296143871,
-11.9476370476987));
#66556=CARTESIAN_POINT('Ctrl Pts',(-0.604253502485025,0.436152983457259,
-11.9370459820358));
#66557=CARTESIAN_POINT('Ctrl Pts',(-0.739811829461958,0.0925825907650836,
-11.9211593835414));
#66558=CARTESIAN_POINT('Ctrl Pts',(-0.692947007893374,-0.270822984187043,
-11.905272785047));
#66559=CARTESIAN_POINT('Ctrl Pts',(-0.409285919167933,-0.673437402061984,
-11.8840906537212));
#66560=CARTESIAN_POINT('Ctrl Pts',(0.248575292524515,-0.80813422424943,
-11.8576129895638));
#66561=CARTESIAN_POINT('Ctrl Pts',(0.814874281174704,-0.226283406359347,
-11.8258397925751));
#66562=CARTESIAN_POINT('Ctrl Pts',(0.661574797042729,0.427775327210025,
-11.7993621284177));
#66563=CARTESIAN_POINT('Ctrl Pts',(0.252019553201191,0.700124195300235,
-11.7781799970919));
#66564=CARTESIAN_POINT('Ctrl Pts',(-0.113896804202068,0.737010561893185,
-11.7622933985975));
#66565=CARTESIAN_POINT('Ctrl Pts',(-0.450904916615657,0.591935197672468,
-11.7464068001031));
#66566=CARTESIAN_POINT('Ctrl Pts',(-0.760463823480222,0.207699378513882,
-11.7252246687772));
#66567=CARTESIAN_POINT('Ctrl Pts',(-0.717957522306204,-0.32597923867788,
-11.7040425374514));
#66568=CARTESIAN_POINT('Ctrl Pts',(-0.351461896485877,-0.655051583268549,
-11.6828604061255));
#66569=CARTESIAN_POINT('Ctrl Pts',(0.122973627023043,-0.778202022613627,
-11.6616782747997));
#66570=CARTESIAN_POINT('Ctrl Pts',(0.71321863385788,-0.455059229729923,
-11.6352006106423));
#66571=CARTESIAN_POINT('Ctrl Pts',(0.767226239823105,0.355052608587047,
-11.6034274136535));
#66572=CARTESIAN_POINT('Ctrl Pts',(0.227493311469381,0.75431223879576,-11.5769497494962));
#66573=CARTESIAN_POINT('Ctrl Pts',(-0.261218076357254,0.696776585846632,
-11.5557676181703));
#66574=CARTESIAN_POINT('Ctrl Pts',(-0.563873923467153,0.488009727699941,
-11.539881019676));
#66575=CARTESIAN_POINT('Ctrl Pts',(-0.726886814028964,0.159273941491993,
-11.5239944211816));
#66576=CARTESIAN_POINT('Ctrl Pts',(-0.714056613740822,-0.333982155042871,
-11.5028122898557));
#66577=CARTESIAN_POINT('Ctrl Pts',(-0.336205356107924,-0.713229621096794,
-11.4816301585299));
#66578=CARTESIAN_POINT('Ctrl Pts',(0.156171374865428,-0.726794128759501,
-11.460448027204));
#66579=CARTESIAN_POINT('Ctrl Pts',(0.59749794928794,-0.513531071236394,
-11.4392658958781));
#66580=CARTESIAN_POINT('Ctrl Pts',(0.838193809590663,0.114861792295151,
-11.4127882317208));
#66581=CARTESIAN_POINT('Ctrl Pts',(0.35492781363207,0.767283632994828,-11.381015034732));
#66582=CARTESIAN_POINT('Ctrl Pts',(-0.314912149164092,0.722198192887193,
-11.3545373705747));
#66583=CARTESIAN_POINT('Ctrl Pts',(-0.650158212070062,0.361976566873907,
-11.3333552392488));
#66584=CARTESIAN_POINT('Ctrl Pts',(-0.745693705839447,0.00693137846112073,
-11.3174686407545));
#66585=CARTESIAN_POINT('Ctrl Pts',(-0.657132874094063,-0.3491548029949,
-11.30158204226));
#66586=CARTESIAN_POINT('Ctrl Pts',(-0.328043197231767,-0.71680441185038,
-11.2803999109342));
#66587=CARTESIAN_POINT('Ctrl Pts',(0.205458269395073,-0.761260418319186,
-11.2592177796083));
#66588=CARTESIAN_POINT('Ctrl Pts',(0.589524335340204,-0.452857892678056,
-11.2380356482825));
#66589=CARTESIAN_POINT('Ctrl Pts',(0.787843027379244,-0.00461692103046995,
-11.2168535169566));
#66590=CARTESIAN_POINT('Ctrl Pts',(0.564507567765378,0.630153396638974,
-11.1903758527993));
#66591=CARTESIAN_POINT('Ctrl Pts',(-0.226180200780229,0.814579918793154,
-11.1586026558105));
#66592=CARTESIAN_POINT('Ctrl Pts',(-0.70753989713274,0.34659368739482,-11.1321249916532));
#66593=CARTESIAN_POINT('Ctrl Pts',(-0.729871026448289,-0.144986278853025,
-11.1109428603273));
#66594=CARTESIAN_POINT('Ctrl Pts',(-0.572847938806445,-0.477443594241456,
-11.0950562618329));
#66595=CARTESIAN_POINT('Ctrl Pts',(-0.274834434169087,-0.691519142555255,
-11.0791696633386));
#66596=CARTESIAN_POINT('Ctrl Pts',(0.213993560575424,-0.758701298387166,
-11.0579875320127));
#66597=CARTESIAN_POINT('Ctrl Pts',(0.649402182312231,-0.447221791185339,
-11.0368054006868));
#66598=CARTESIAN_POINT('Ctrl Pts',(0.742488688495841,0.0364658799499072,
-11.015623269361));
#66599=CARTESIAN_POINT('Ctrl Pts',(0.603475495194033,0.506493117855511,
-10.9944411380351));
#66600=CARTESIAN_POINT('Ctrl Pts',(0.0223311557836704,0.845732473564332,
-10.9679634738778));
#66601=CARTESIAN_POINT('Ctrl Pts',(-0.699712755981378,0.474447032290606,
-10.936190276889));
#66602=CARTESIAN_POINT('Ctrl Pts',(-0.763648675099599,-0.193857141194035,
-10.9097126127317));
#66603=CARTESIAN_POINT('Ctrl Pts',(-0.462443774570201,-0.582990987637431,
-10.8885304814058));
#66604=CARTESIAN_POINT('Ctrl Pts',(-0.127545170575338,-0.734737624012674,
-10.8726438829114));
#66605=CARTESIAN_POINT('Ctrl Pts',(0.23818031069733,-0.704984276648341,
-10.856757284417));
#66606=CARTESIAN_POINT('Ctrl Pts',(0.654251050420993,-0.439745912050845,
-10.8355751530912));
#66607=CARTESIAN_POINT('Ctrl Pts',(0.784478489585921,0.0795237340656153,
-10.8143930217653));
#66608=CARTESIAN_POINT('Ctrl Pts',(0.54231178387317,0.508445810305424,-10.7932108904395));
#66609=CARTESIAN_POINT('Ctrl Pts',(0.132083933285029,0.776705726966545,
-10.7720287591136));
#66610=CARTESIAN_POINT('Ctrl Pts',(-0.530466364057635,0.659065652240602,
-10.7455510949563));
#66611=CARTESIAN_POINT('Ctrl Pts',(-0.84044907259622,-0.0913415770861792,
-10.7137778979675));
#66612=CARTESIAN_POINT('Ctrl Pts',(-0.456552117021781,-0.642105952796128,
-10.6873002338102));
#66613=CARTESIAN_POINT('Ctrl Pts',(0.0249302303405187,-0.743714474728285,
-10.6661181024843));
#66614=CARTESIAN_POINT('Ctrl Pts',(0.378420423442174,-0.642576944652335,
-10.6502315039899));
#66615=CARTESIAN_POINT('Ctrl Pts',(0.637912125065641,-0.383145940105722,
-10.6343449054955));
#66616=CARTESIAN_POINT('Ctrl Pts',(0.78333472385694,0.0883607070047231,
-10.6131627741697));
#66617=CARTESIAN_POINT('Ctrl Pts',(0.546442418456161,0.568446310758132,
-10.5919806428438));
#66618=CARTESIAN_POINT('Ctrl Pts',(0.0842014340339106,0.738599574499925,
-10.5707985115179));
#66619=CARTESIAN_POINT('Ctrl Pts',(-0.402129173320327,0.677502826340514,
-10.5496163801921));
#66620=CARTESIAN_POINT('Ctrl Pts',(-0.83096433791511,0.158935101450751,
-10.5231387160348));
#66621=CARTESIAN_POINT('Ctrl Pts',(-0.581452373499001,-0.613686454702083,
-10.491365519046));
#66622=CARTESIAN_POINT('Ctrl Pts',(0.0676890135440266,-0.784957379491861,
-10.4648878548887));
#66623=CARTESIAN_POINT('Ctrl Pts',(0.500446959800122,-0.550713697607039,
-10.4437057235628));
#66624=CARTESIAN_POINT('Ctrl Pts',(0.704402313506879,-0.244794868007973,
-10.4278191250684));
#66625=CARTESIAN_POINT('Ctrl Pts',(0.734241216025536,0.120923642909903,
-10.411932526574));
#66626=CARTESIAN_POINT('Ctrl Pts',(0.539850014877955,0.574441350860708,
-10.3907503952481));
#66627=CARTESIAN_POINT('Ctrl Pts',(0.048508296433538,0.787005381226751,
-10.3695682639223));
#66628=CARTESIAN_POINT('Ctrl Pts',(-0.413956664385384,0.617461814977869,
-10.3483861325964));
#66629=CARTESIAN_POINT('Ctrl Pts',(-0.745082259064963,0.256067137605208,
-10.3272040012706));
#66630=CARTESIAN_POINT('Ctrl Pts',(-0.736240410083894,-0.416787902798724,
-10.3007263371133));
#66631=CARTESIAN_POINT('Ctrl Pts',(-0.0459062458519896,-0.844150782694781,
-10.2689531401245));
#66632=CARTESIAN_POINT('Ctrl Pts',(0.559736006003475,-0.554468658948882,
-10.2424754759671));
#66633=CARTESIAN_POINT('Ctrl Pts',(0.737941923316341,-0.0957833707768819,
-10.2212933446413));
#66634=CARTESIAN_POINT('Ctrl Pts',(0.695357525294872,0.269416144083229,
-10.2054067461469));
#66635=CARTESIAN_POINT('Ctrl Pts',(0.481351698610594,0.567479720316027,
-10.1895201476525));
#66636=CARTESIAN_POINT('Ctrl Pts',(0.0396027232325981,0.787307137307268,
-10.1683380163266));
#66637=CARTESIAN_POINT('Ctrl Pts',(-0.4724972623396,0.631250237215267,-10.1471558850008));
#66638=CARTESIAN_POINT('Ctrl Pts',(-0.715229369954264,0.20264787514224,
-10.1259737536749));
#66639=CARTESIAN_POINT('Ctrl Pts',(-0.733660537244455,-0.287158785038608,
-10.1047916223491));
#66640=CARTESIAN_POINT('Ctrl Pts',(-0.291347020463876,-0.794278925206177,
-10.0783139581917));
#66641=CARTESIAN_POINT('Ctrl Pts',(0.511473735496293,-0.673121493662104,
-10.046540761203));
#66642=CARTESIAN_POINT('Ctrl Pts',(0.785562273165169,-0.0602644601142881,
-10.0200630970456));
#66643=CARTESIAN_POINT('Ctrl Pts',(0.624458154098192,0.404703286477242,
-9.99888096571979));
#66644=CARTESIAN_POINT('Ctrl Pts',(0.355587926208178,0.655487889599687,
-9.98299436722537));
#66645=CARTESIAN_POINT('Ctrl Pts',(-0.000477527797489372,0.744132019666176,
-9.96710776873098));
#66646=CARTESIAN_POINT('Ctrl Pts',(-0.479480350977519,0.625715188539386,
-9.94592563740513));
#66647=CARTESIAN_POINT('Ctrl Pts',(-0.768774444642223,0.175260886017933,
-9.92474350607927));
#66648=CARTESIAN_POINT('Ctrl Pts',(-0.676325850336198,-0.308549116206573,
-9.90356137475341));
#66649=CARTESIAN_POINT('Ctrl Pts',(-0.373296388542898,-0.693806715184786,
-9.88237924342755));
#66650=CARTESIAN_POINT('Ctrl Pts',(0.292116363348639,-0.793996302021506,
-9.85590157927023));
#66651=CARTESIAN_POINT('Ctrl Pts',(0.825587413847927,-0.181943258815281,
-9.82412838228143));
#66652=CARTESIAN_POINT('Ctrl Pts',(0.637760694546856,0.462602622846441,
-9.79765071812413));
#66653=CARTESIAN_POINT('Ctrl Pts',(0.213970617176942,0.712705627373687,
-9.77646858679825));
#66654=CARTESIAN_POINT('Ctrl Pts',(-0.153305821775376,0.729797555275886,
-9.76058198830387));
#66655=CARTESIAN_POINT('Ctrl Pts',(-0.482079633214187,0.566861462762583,
-9.74469538980946));
#66656=CARTESIAN_POINT('Ctrl Pts',(-0.770513763500401,0.166521603399833,
-9.72351325848364));
#66657=CARTESIAN_POINT('Ctrl Pts',(-0.699408380757533,-0.364085761639854,
-9.70233112715773));
#66658=CARTESIAN_POINT('Ctrl Pts',(-0.315749334014388,-0.672994480671505,
-9.68114899583192));
#66659=CARTESIAN_POINT('Ctrl Pts',(0.16461437899866,-0.770467428228838,
-9.65996686450602));
#66660=CARTESIAN_POINT('Ctrl Pts',(0.736643839361908,-0.416074454022362,
-9.63348920034873));
#66661=CARTESIAN_POINT('Ctrl Pts',(0.747036554356828,0.395770531731598,
-9.60171600335992));
#66662=CARTESIAN_POINT('Ctrl Pts',(0.186628415656226,0.765447401617473,
-9.5752383392026));
#66663=CARTESIAN_POINT('Ctrl Pts',(-0.298285275337462,0.68173208140886,
-9.55405620787676));
#66664=CARTESIAN_POINT('Ctrl Pts',(-0.589284505107621,0.457002099247858,
-9.53816960938235));
#66665=CARTESIAN_POINT('Ctrl Pts',(-0.734395810570078,0.119981182451158,
-9.52228301088797));
#66666=CARTESIAN_POINT('Ctrl Pts',(-0.69507667784042,-0.371872714869924,
-9.5011008795621));
#66667=CARTESIAN_POINT('Ctrl Pts',(-0.297390844736814,-0.730266533787131,
-9.47991874823625));
#66668=CARTESIAN_POINT('Ctrl Pts',(0.195003365029303,-0.717351309033507,
-9.45873661691039));
#66669=CARTESIAN_POINT('Ctrl Pts',(0.624231524365783,-0.480679680996236,
-9.43755448558453));
#66670=CARTESIAN_POINT('Ctrl Pts',(0.830809975211841,0.159740046476628,
-9.41107682142721));
#66671=CARTESIAN_POINT('Ctrl Pts',(0.313181388564641,0.785248588148464,
-9.37930362443842));
#66672=CARTESIAN_POINT('Ctrl Pts',(-0.353267765581714,0.704231336972586,
-9.35282596028109));
#66673=CARTESIAN_POINT('Ctrl Pts',(-0.668671212204437,0.326514235944241,
-9.33164382895525));
#66674=CARTESIAN_POINT('Ctrl Pts',(-0.744988654241857,-0.0331519490798406,
-9.31575723046083));
#66675=CARTESIAN_POINT('Ctrl Pts',(-0.637419851546266,-0.383964351965119,
-9.29987063196646));
#66676=CARTESIAN_POINT('Ctrl Pts',(-0.289048357513512,-0.733397539647596,
-9.27868850064058));
#66677=CARTESIAN_POINT('Ctrl Pts',(0.246071239309372,-0.749119129436365,
-9.25750636931473));
#66678=CARTESIAN_POINT('Ctrl Pts',(0.613008881978574,-0.42052267900818,
-9.23632423798887));
#66679=CARTESIAN_POINT('Ctrl Pts',(0.786952691293118,0.0377281513089534,
-9.21514210666303));
#66680=CARTESIAN_POINT('Ctrl Pts',(0.529827627109992,0.659579246877018,
-9.18866444250567));
#66681=CARTESIAN_POINT('Ctrl Pts',(-0.269628597927286,0.801247993140825,
-9.15689124551692));
#66682=CARTESIAN_POINT('Ctrl Pts',(-0.72514330893185,0.30806991363108,-9.13041358135957));
#66683=CARTESIAN_POINT('Ctrl Pts',(-0.721024838858224,-0.18399977732235,
-9.10923145003374));
#66684=CARTESIAN_POINT('Ctrl Pts',(-0.546362515984092,-0.507538321513182,
-9.09334485153932));
#66685=CARTESIAN_POINT('Ctrl Pts',(-0.237275303441589,-0.705289388196051,
-9.07745825304495));
#66686=CARTESIAN_POINT('Ctrl Pts',(0.254456670686461,-0.746105024031849,
-9.05627612171907));
#66687=CARTESIAN_POINT('Ctrl Pts',(0.672497322274279,-0.411676907825386,
-9.03509399039321));
#66688=CARTESIAN_POINT('Ctrl Pts',(0.73945611533713,0.0763142610221662,
-9.01391185906737));
#66689=CARTESIAN_POINT('Ctrl Pts',(0.575384704040563,0.538191781887113,
-8.99272972774149));
#66690=CARTESIAN_POINT('Ctrl Pts',(-0.023150471951528,0.845710442768847,
-8.96625206358419));
#66691=CARTESIAN_POINT('Ctrl Pts',(-0.724198270894036,0.436159135828339,
-8.93447886659538));
#66692=CARTESIAN_POINT('Ctrl Pts',(-0.75212737562495,-0.234615219047742,
-8.90800120243808));
#66693=CARTESIAN_POINT('Ctrl Pts',(-0.43044580886719,-0.607000116914215,
-8.88681907111221));
#66694=CARTESIAN_POINT('Ctrl Pts',(-0.0878763299167745,-0.740530146123197,
-8.87093247261782));
#66695=CARTESIAN_POINT('Ctrl Pts',(0.275721737088013,-0.691165837134929,
-8.85504587412342));
#66696=CARTESIAN_POINT('Ctrl Pts',(0.676937432624418,-0.403951255047272,
-8.83386374279756));
#66697=CARTESIAN_POINT('Ctrl Pts',(0.779071326801438,0.121566412543086,
-8.81268161147172));
#66698=CARTESIAN_POINT('Ctrl Pts',(0.514204438424602,0.536854736822985,
-8.79149948014584));
#66699=CARTESIAN_POINT('Ctrl Pts',(0.090153183279391,0.782681515866618,
-8.77031734882));
#66700=CARTESIAN_POINT('Ctrl Pts',(-0.565117781341099,0.629606218657323,
-8.74383968466265));
#66701=CARTESIAN_POINT('Ctrl Pts',(-0.834325944652335,-0.136375017552418,
-8.71206648767389));
#66702=CARTESIAN_POINT('Ctrl Pts',(-0.421385847917164,-0.665713044297937,
-8.68558882351655));
#66703=CARTESIAN_POINT('Ctrl Pts',(0.0648611539509664,-0.741300051944791,
-8.6644066921907));
#66704=CARTESIAN_POINT('Ctrl Pts',(0.412405452710403,-0.621312231693223,
-8.6485200936963));
#66705=CARTESIAN_POINT('Ctrl Pts',(0.657580455193039,-0.348311119078007,
-8.63263349520191));
#66706=CARTESIAN_POINT('Ctrl Pts',(0.777454318089235,0.130329150334099,
-8.61145136387606));
#66707=CARTESIAN_POINT('Ctrl Pts',(0.515104698860376,0.596990514258567,
-8.59026923255019));
#66708=CARTESIAN_POINT('Ctrl Pts',(0.0443876860470674,0.742057239215564,
-8.56908710122434));
#66709=CARTESIAN_POINT('Ctrl Pts',(-0.437956847320566,0.654913545149056,
-8.54790496989848));
#66710=CARTESIAN_POINT('Ctrl Pts',(-0.838304694233625,0.114049712782297,
-8.52142730574116));
#66711=CARTESIAN_POINT('Ctrl Pts',(-0.547632874814056,-0.644046707743566,
-8.48965410875236));
#66712=CARTESIAN_POINT('Ctrl Pts',(0.109774528782839,-0.780185518324841,
-8.46317644459505));
#66713=CARTESIAN_POINT('Ctrl Pts',(0.529318960625381,-0.523024066585532,
-8.44199431326918));
#66714=CARTESIAN_POINT('Ctrl Pts',(0.716539627251363,-0.206586808038074,
-8.4261077147748));
#66715=CARTESIAN_POINT('Ctrl Pts',(0.726681830826818,0.160206764749315,
-8.41022111628039));
#66716=CARTESIAN_POINT('Ctrl Pts',(0.508199650129457,0.602622618021181,
-8.38903898495455));
#66717=CARTESIAN_POINT('Ctrl Pts',(0.00614481505570648,0.788474962285219,
-8.36785685362867));
#66718=CARTESIAN_POINT('Ctrl Pts',(-0.446540665096658,0.594323689044844,
-8.34667472230284));
#66719=CARTESIAN_POINT('Ctrl Pts',(-0.757766557247427,0.215656663361126,
-8.32549259097696));
#66720=CARTESIAN_POINT('Ctrl Pts',(-0.712778497149809,-0.455750931277951,
-8.29901492681964));
#66721=CARTESIAN_POINT('Ctrl Pts',(-0.000475551173634113,-0.845397954328917,
-8.26724172983087));
#66722=CARTESIAN_POINT('Ctrl Pts',(0.588724123331353,-0.523587429930306,
-8.24076406567352));
#66723=CARTESIAN_POINT('Ctrl Pts',(0.742022947463043,-0.0559882286151282,
-8.21958193434769));
#66724=CARTESIAN_POINT('Ctrl Pts',(0.679874394168988,0.306395095963096,
-8.20369533585327));
#66725=CARTESIAN_POINT('Ctrl Pts',(0.450159980531817,0.592527368695197,
-8.18780873735889));
#66726=CARTESIAN_POINT('Ctrl Pts',(-0.00276410569037474,0.78829770002337,
-8.16662660603303));
#66727=CARTESIAN_POINT('Ctrl Pts',(-0.505737655653165,0.604946236088125,
-8.14544447470717));
#66728=CARTESIAN_POINT('Ctrl Pts',(-0.725086074171385,0.163918876239337,
-8.12426234338131));
#66729=CARTESIAN_POINT('Ctrl Pts',(-0.717168574417189,-0.326170488553287,
-8.10308021205545));
#66730=CARTESIAN_POINT('Ctrl Pts',(-0.248241755000774,-0.808788061505605,
-8.07660254789813));
#66731=CARTESIAN_POINT('Ctrl Pts',(0.546907953339569,-0.644662406152521,
-8.04482935090935));
#66732=CARTESIAN_POINT('Ctrl Pts',(0.787665711547366,-0.017961542970373,
-8.01835168675202));
#66733=CARTESIAN_POINT('Ctrl Pts',(0.601807191524753,0.437676639237566,
-7.99716955542616));
#66734=CARTESIAN_POINT('Ctrl Pts',(0.319848411758804,0.673649864671741,
-7.98128295693177));
#66735=CARTESIAN_POINT('Ctrl Pts',(-0.0404662247302287,0.743031072958151,
-7.96539635843737));
#66736=CARTESIAN_POINT('Ctrl Pts',(-0.512413202074689,0.599043916989371,
-7.94421422711151));
#66737=CARTESIAN_POINT('Ctrl Pts',(-0.777082008295114,0.133693968774884,
-7.92303209578568));
#66738=CARTESIAN_POINT('Ctrl Pts',(-0.658767228492401,-0.344448764853758,
-7.90184996445978));
#66739=CARTESIAN_POINT('Ctrl Pts',(-0.335472045139475,-0.712864965238586,
-7.88066783313396));
#66740=CARTESIAN_POINT('Ctrl Pts',(0.334363325358902,-0.777150734423377,
-7.8541901689766));
#66741=CARTESIAN_POINT('Ctrl Pts',(0.834171990018743,-0.137313576898307,
-7.82241697198784));
#66742=CARTESIAN_POINT('Ctrl Pts',(0.6119790200543,0.496207183731426,-7.7959393078305));
#66743=CARTESIAN_POINT('Ctrl Pts',(0.175360881720452,0.723174458528111,
-7.77475717650466));
#66744=CARTESIAN_POINT('Ctrl Pts',(-0.19230335003752,0.720504384609304,
-7.75887057801025));
#66745=CARTESIAN_POINT('Ctrl Pts',(-0.511845950255046,0.540135551443124,
-7.74298397951587));
#66746=CARTESIAN_POINT('Ctrl Pts',(-0.7783491679022,0.124873844212295,-7.72180184819));
#66747=CARTESIAN_POINT('Ctrl Pts',(-0.678831884888873,-0.401145605685725,
-7.70061971686414));
#66748=CARTESIAN_POINT('Ctrl Pts',(-0.279126589163162,-0.68899024678654,
-7.67943758553829));
#66749=CARTESIAN_POINT('Ctrl Pts',(0.205781150524281,-0.760507771047459,
-7.65825545421242));
#66750=CARTESIAN_POINT('Ctrl Pts',(0.757939066824373,-0.375886243884045,
-7.63177779005511));
#66751=CARTESIAN_POINT('Ctrl Pts',(0.724688506752804,0.435344111609228,
-7.60000459306631));
#66752=CARTESIAN_POINT('Ctrl Pts',(0.145223866217483,0.774370659861374,
-7.573526928909));
#66753=CARTESIAN_POINT('Ctrl Pts',(-0.334490284337073,0.664717222576117,
-7.55234479758313));
#66754=CARTESIAN_POINT('Ctrl Pts',(-0.612992106461524,0.424673785502175,
-7.53645819908875));
#66755=CARTESIAN_POINT('Ctrl Pts',(-0.73978234060737,0.0803416408267936,
-7.52057160059435));
#66756=CARTESIAN_POINT('Ctrl Pts',(-0.674087973298083,-0.408688522468257,
-7.49938946926849));
#66757=CARTESIAN_POINT('Ctrl Pts',(-0.257716848716532,-0.745192962118112,
-7.47820733794264));
#66758=CARTESIAN_POINT('Ctrl Pts',(0.233271782775553,-0.705835312452951,
-7.45702520661677));
#66759=CARTESIAN_POINT('Ctrl Pts',(0.649161051353326,-0.446439112467214,
-7.43584307529092));
#66760=CARTESIAN_POINT('Ctrl Pts',(0.821025066809404,0.204156648264201,
-7.40936541113359));
#66761=CARTESIAN_POINT('Ctrl Pts',(0.270529859099672,0.800944144536901,
-7.37759221414481));
#66762=CARTESIAN_POINT('Ctrl Pts',(-0.390602425763559,0.684229227058386,
-7.35111454998748));
#66763=CARTESIAN_POINT('Ctrl Pts',(-0.685251727478478,0.29010826650229,
-7.32993241866163));
#66764=CARTESIAN_POINT('Ctrl Pts',(-0.742130558038833,-0.073139466103157,
-7.31404582016723));
#66765=CARTESIAN_POINT('Ctrl Pts',(-0.615864661958205,-0.417664229826262,
-7.29815922167284));
#66766=CARTESIAN_POINT('Ctrl Pts',(-0.249218157413321,-0.747871121355755,
-7.27697709034698));
#66767=CARTESIAN_POINT('Ctrl Pts',(0.285973054269614,-0.734812858579961,
-7.25579495902112));
#66768=CARTESIAN_POINT('Ctrl Pts',(0.634721810251999,-0.386972139223568,
-7.23461282769526));
#66769=CARTESIAN_POINT('Ctrl Pts',(0.783788032819058,0.079964187886226,
-7.2134306963694));
#66770=CARTESIAN_POINT('Ctrl Pts',(0.493616465001244,0.687098888690364,
-7.18695303221208));
#66771=CARTESIAN_POINT('Ctrl Pts',(-0.312297758445966,0.785600431136631,
-7.15517983522329));
#66772=CARTESIAN_POINT('Ctrl Pts',(-0.740651029737173,0.268655806418843,
-7.12870217106597));
#66773=CARTESIAN_POINT('Ctrl Pts',(-0.710094862802953,-0.222481509627331,
-7.10752003974011));
#66774=CARTESIAN_POINT('Ctrl Pts',(-0.518298085273821,-0.536166244254872,
-7.09163344124572));
#66775=CARTESIAN_POINT('Ctrl Pts',(-0.199030438307018,-0.717021321407235,
-7.07574684275133));
#66776=CARTESIAN_POINT('Ctrl Pts',(0.294184391603376,-0.731352478548719,
-7.05456471142545));
#66777=CARTESIAN_POINT('Ctrl Pts',(0.693648920090533,-0.374942262968557,
-7.03338258009962));
#66778=CARTESIAN_POINT('Ctrl Pts',(0.734286486642884,0.115942091056241,
-7.01220044877374));
#66779=CARTESIAN_POINT('Ctrl Pts',(0.545631029801399,0.568335051754265,
-6.9910183174479));
#66780=CARTESIAN_POINT('Ctrl Pts',(-0.068565193966149,0.843244277499859,
-6.96454065329056));
#66781=CARTESIAN_POINT('Ctrl Pts',(-0.746590826006241,0.396610723324246,
-6.93276745630179));
#66782=CARTESIAN_POINT('Ctrl Pts',(-0.738432400203635,-0.274695250236871,
-6.90628979214445));
#66783=CARTESIAN_POINT('Ctrl Pts',(-0.397203838848781,-0.629254993392277,
-6.88510766081861));
#66784=CARTESIAN_POINT('Ctrl Pts',(-0.0479535234128937,-0.744182508709381,
-6.86922106232419));
#66785=CARTESIAN_POINT('Ctrl Pts',(0.312466317455657,-0.675349902777122,
-6.85333446382982));
#66786=CARTESIAN_POINT('Ctrl Pts',(0.697667440599412,-0.366989163968669,
-6.83215233250394));
#66787=CARTESIAN_POINT('Ctrl Pts',(0.771412619053169,0.16325775958901,-6.81097020117811));
#66788=CARTESIAN_POINT('Ctrl Pts',(0.484611023123308,0.56371213328692,-6.78978806985223));
#66789=CARTESIAN_POINT('Ctrl Pts',(0.047961887234688,0.786395326221602,
-6.76860593852638));
#66790=CARTESIAN_POINT('Ctrl Pts',(-0.598135987318,0.598327199810221,-6.74212827436906));
#66791=CARTESIAN_POINT('Ctrl Pts',(-0.825791583868712,-0.18101432918127,
-6.71035507738028));
#66792=CARTESIAN_POINT('Ctrl Pts',(-0.385001758097536,-0.687396200451901,
-6.68387741322294));
#66793=CARTESIAN_POINT('Ctrl Pts',(0.104604626396011,-0.736743244603411,
-6.6626952818971));
#66794=CARTESIAN_POINT('Ctrl Pts',(0.445198615026306,-0.598251903344638,
-6.64680868340269));
#66795=CARTESIAN_POINT('Ctrl Pts',(0.675348353348783,-0.312469666119661,
-6.63092208490831));
#66796=CARTESIAN_POINT('Ctrl Pts',(0.769327040856058,0.171920937806506,
-6.60973995358243));
#66797=CARTESIAN_POINT('Ctrl Pts',(0.482278307083611,0.623809392679397,
-6.5885578222566));
#66798=CARTESIAN_POINT('Ctrl Pts',(0.0044456566373652,0.743370331522448,
-6.56737569093072));
#66799=CARTESIAN_POINT('Ctrl Pts',(-0.472518811304924,0.630431538476766,
-6.54619355960487));
#66800=CARTESIAN_POINT('Ctrl Pts',(-0.843222315817966,0.0688347185687733,
-6.51971589544755));
#66801=CARTESIAN_POINT('Ctrl Pts',(-0.512230702407081,-0.672545646102564,
-6.48794269845875));
#66802=CARTESIAN_POINT('Ctrl Pts',(0.151542800970993,-0.77315888513845,
-6.46146503430144));
#66803=CARTESIAN_POINT('Ctrl Pts',(0.556661197052577,-0.493822886353796,
-6.44028290297557));
#66804=CARTESIAN_POINT('Ctrl Pts',(0.726606143350278,-0.16778168339867,
-6.42439630448119));
#66805=CARTESIAN_POINT('Ctrl Pts',(0.717022255325511,0.199026843686629,
-6.40850970598679));
#66806=CARTESIAN_POINT('Ctrl Pts',(0.475080690338507,0.629062373469418,
-6.38732757466093));
#66807=CARTESIAN_POINT('Ctrl Pts',(-0.036236656606484,0.78766564904173,
-6.36614544333508));
#66808=CARTESIAN_POINT('Ctrl Pts',(-0.477833876060214,0.56946814731603,
-6.34496331200921));
#66809=CARTESIAN_POINT('Ctrl Pts',(-0.768261515109739,0.174622461779635,
-6.32378118068336));
#66810=CARTESIAN_POINT('Ctrl Pts',(-0.687255280232435,-0.493395818705134,
-6.29730351652604));
#66811=CARTESIAN_POINT('Ctrl Pts',(0.0449541415847475,-0.844203664783362,
-6.26553031953724));
#66812=CARTESIAN_POINT('Ctrl Pts',(0.616014830444453,-0.491190016005719,
-6.23905265537993));
#66813=CARTESIAN_POINT('Ctrl Pts',(0.743953925476331,-0.0160354294836368,
-6.21787052405406));
#66814=CARTESIAN_POINT('Ctrl Pts',(0.662438556258499,0.342497609724965,
-6.20198392555968));
#66815=CARTESIAN_POINT('Ctrl Pts',(0.417644625691115,0.61584571232203,-6.18609732706527));
#66816=CARTESIAN_POINT('Ctrl Pts',(-0.0450712489042535,0.787048564929024,
-6.16491519573942));
#66817=CARTESIAN_POINT('Ctrl Pts',(-0.537615573110493,0.576820073921749,
-6.14373306441357));
#66818=CARTESIAN_POINT('Ctrl Pts',(-0.732731387322439,0.124802468022666,
-6.1225509330877));
#66819=CARTESIAN_POINT('Ctrl Pts',(-0.698874509772504,-0.364441229918025,
-6.10136880176184));
#66820=CARTESIAN_POINT('Ctrl Pts',(-0.203848075213461,-0.820532664836046,
-6.07489113760452));
#66821=CARTESIAN_POINT('Ctrl Pts',(0.579781559557804,-0.615081213840891,
-6.04311794061573));
#66822=CARTESIAN_POINT('Ctrl Pts',(0.830826746056493,0.153711188366667,
-6.01134474362695));
#66823=CARTESIAN_POINT('Ctrl Pts',(0.321082505138741,0.781540937050481,
-5.97957154663815));
#66824=CARTESIAN_POINT('Ctrl Pts',(-0.482882123813584,0.693755296141619,
-5.94779834964938));
#66825=CARTESIAN_POINT('Ctrl Pts',(-0.844907628832503,-0.0309675729080316,
-5.91602515266057));
#66826=CARTESIAN_POINT('Ctrl Pts',(-0.500217074565313,-0.609118928278575,
-5.88954748850327));
#66827=CARTESIAN_POINT('Ctrl Pts',(-0.0283586531132722,-0.742742706989181,
-5.86836535717739));
#66828=CARTESIAN_POINT('Ctrl Pts',(0.4540974835594,-0.644629643714152,-5.84718322585155));
#66829=CARTESIAN_POINT('Ctrl Pts',(0.761010378138235,-0.205767017280531,
-5.82600109452568));
#66830=CARTESIAN_POINT('Ctrl Pts',(0.688497809353763,0.282247659457379,
-5.80481896319983));
#66831=CARTESIAN_POINT('Ctrl Pts',(0.47125751192046,0.577966963540043,-5.78893236470543));
#66832=CARTESIAN_POINT('Ctrl Pts',(0.137111726801814,0.731385638773274,
-5.77304576621104));
#66833=CARTESIAN_POINT('Ctrl Pts',(-0.354190246329251,0.703769260877763,
-5.75186363488517));
#66834=CARTESIAN_POINT('Ctrl Pts',(-0.816970922862985,0.217391843627321,
-5.72538597072787));
#66835=CARTESIAN_POINT('Ctrl Pts',(-0.624035667222098,-0.571260658681954,
-5.69361277373906));
#66836=CARTESIAN_POINT('Ctrl Pts',(0.0131013734634179,-0.787748128382458,
-5.66713510958175));
#66837=CARTESIAN_POINT('Ctrl Pts',(0.459181237710636,-0.584612499740476,
-5.64595297825589));
#66838=CARTESIAN_POINT('Ctrl Pts',(0.763428896494617,-0.19724753473581,
-5.62477084693002));
#66839=CARTESIAN_POINT('Ctrl Pts',(0.713229822891815,0.335744473945888,
-5.60358871560418));
#66840=CARTESIAN_POINT('Ctrl Pts',(0.342056978743302,0.660855220477942,
-5.58240658427831));
#66841=CARTESIAN_POINT('Ctrl Pts',(-0.0149623003848158,0.745575824719156,
-5.56651998578392));
#66842=CARTESIAN_POINT('Ctrl Pts',(-0.368957988145881,0.646221892521559,
-5.55063338728953));
#66843=CARTESIAN_POINT('Ctrl Pts',(-0.725547995671562,0.307115594152496,
-5.52945125596367));
#66844=CARTESIAN_POINT('Ctrl Pts',(-0.763416454169478,-0.363171111300542,
-5.50297359180634));
#66845=CARTESIAN_POINT('Ctrl Pts',(-0.105827519704371,-0.839382289810237,
-5.47120039481756));
#66846=CARTESIAN_POINT('Ctrl Pts',(0.519936517239823,-0.591932403052683,
-5.44472273066023));
#66847=CARTESIAN_POINT('Ctrl Pts',(0.7284339930835,-0.148334525216346,-5.42354059933438));
#66848=CARTESIAN_POINT('Ctrl Pts',(0.709567204017975,0.343867571690883,
-5.40235846800852));
#66849=CARTESIAN_POINT('Ctrl Pts',(0.326272201059984,0.717612259834014,
-5.38117633668267));
#66850=CARTESIAN_POINT('Ctrl Pts',(-0.167093531027814,0.725129259170048,
-5.3599942053568));
#66851=CARTESIAN_POINT('Ctrl Pts',(-0.494054449540532,0.558585130097485,
-5.34410760686241));
#66852=CARTESIAN_POINT('Ctrl Pts',(-0.699549695773513,0.253698560254875,
-5.32822100836801));
#66853=CARTESIAN_POINT('Ctrl Pts',(-0.751818044764839,-0.235604579114837,
-5.30703887704216));
#66854=CARTESIAN_POINT('Ctrl Pts',(-0.346769310602394,-0.771005170269097,
-5.28056121288483));
#66855=CARTESIAN_POINT('Ctrl Pts',(0.462715394887025,-0.708277177870474,
-5.24878801589604));
#66856=CARTESIAN_POINT('Ctrl Pts',(0.779479714111498,-0.114583275476619,
-5.22231035173873));
#66857=CARTESIAN_POINT('Ctrl Pts',(0.651230414035533,0.358494296722582,
-5.20112822041286));
#66858=CARTESIAN_POINT('Ctrl Pts',(0.318222100876526,0.721432754603103,
-5.17994608908701));
#66859=CARTESIAN_POINT('Ctrl Pts',(-0.21586635990173,0.758170573687571,
-5.15876395776115));
#66860=CARTESIAN_POINT('Ctrl Pts',(-0.596771337661512,0.444518459989074,
-5.13758182643529));
#66861=CARTESIAN_POINT('Ctrl Pts',(-0.738165201609358,0.105921111256041,
-5.12169522794089));
#66862=CARTESIAN_POINT('Ctrl Pts',(-0.697422731366996,-0.259488477736339,
-5.1058086294465));
#66863=CARTESIAN_POINT('Ctrl Pts',(-0.420509614143643,-0.666266879400412,
-5.08462649812064));
#66864=CARTESIAN_POINT('Ctrl Pts',(0.234807681137167,-0.812135013536203,
-5.05814883396333));
#66865=CARTESIAN_POINT('Ctrl Pts',(0.811182371766064,-0.240302428401924,
-5.02637563697453));
#66866=CARTESIAN_POINT('Ctrl Pts',(0.668288040632482,0.417263761285658,
-4.99989797281721));
#66867=CARTESIAN_POINT('Ctrl Pts',(0.264289689312711,0.694816647086003,
-4.97871584149136));
#66868=CARTESIAN_POINT('Ctrl Pts',(-0.22447527882807,0.755871268204979,
-4.95753371016549));
#66869=CARTESIAN_POINT('Ctrl Pts',(-0.655334914948076,0.438129037376436,
-4.93635157883964));
#66870=CARTESIAN_POINT('Ctrl Pts',(-0.742613735136722,-0.0475134834709792,
-4.91516944751378));
#66871=CARTESIAN_POINT('Ctrl Pts',(-0.631191025624889,-0.397120933529679,
-4.89928284901938));
#66872=CARTESIAN_POINT('Ctrl Pts',(-0.363588706173925,-0.649258029636888,
-4.88339625052499));
#66873=CARTESIAN_POINT('Ctrl Pts',(0.110800912613465,-0.780040414297433,
-4.86221411919913));
#66874=CARTESIAN_POINT('Ctrl Pts',(0.704705826931277,-0.466998527643861,
-4.83573645504181));
#66875=CARTESIAN_POINT('Ctrl Pts',(0.773836113405174,0.341964569728843,
-4.80396325805302));
#66876=CARTESIAN_POINT('Ctrl Pts',(0.239246300374524,0.750652489166442,
-4.7774855938957));
#66877=CARTESIAN_POINT('Ctrl Pts',(-0.248352065935438,0.700671438186571,
-4.75630346256984));
#66878=CARTESIAN_POINT('Ctrl Pts',(-0.660408092917064,0.430803523328669,
-4.73512133124398));
#66879=CARTESIAN_POINT('Ctrl Pts',(-0.783114147707591,-0.0902947163604663,
-4.71393919991813));
#66880=CARTESIAN_POINT('Ctrl Pts',(-0.535255400367477,-0.516947141497766,
-4.69275706859226));
#66881=CARTESIAN_POINT('Ctrl Pts',(-0.224010804574387,-0.711284968286846,
-4.67687047009788));
#66882=CARTESIAN_POINT('Ctrl Pts',(0.143174785820403,-0.730228537521291,
-4.66098387160347));
#66883=CARTESIAN_POINT('Ctrl Pts',(0.589412490217385,-0.522812400913593,
-4.63980174027763));
#66884=CARTESIAN_POINT('Ctrl Pts',(0.839432937889302,0.100251035500731,
-4.61332407612029));
#66885=CARTESIAN_POINT('Ctrl Pts',(0.368439186224119,0.761586937528716,
-4.58155087913152));
#66886=CARTESIAN_POINT('Ctrl Pts',(-0.303585374651586,0.72701710573571,
-4.55507321497418));
#66887=CARTESIAN_POINT('Ctrl Pts',(-0.642873017066318,0.373274023838906,
-4.53389108364834));
#66888=CARTESIAN_POINT('Ctrl Pts',(-0.782238688097199,-0.0991622899429063,
-4.51270895232246));
#66889=CARTESIAN_POINT('Ctrl Pts',(-0.538429908120204,-0.575772644525661,
-4.49152682099662));
#66890=CARTESIAN_POINT('Ctrl Pts',(-0.0733197659837324,-0.740511244101904,
-4.47034468967075));
#66891=CARTESIAN_POINT('Ctrl Pts',(0.2897130696067,-0.687148807738141,-4.45445809117637));
#66892=CARTESIAN_POINT('Ctrl Pts',(0.581841719943463,-0.46388894062958,
-4.43857149268196));
#66893=CARTESIAN_POINT('Ctrl Pts',(0.787688661554364,-0.0169252069998933,
-4.41738936135611));
#66894=CARTESIAN_POINT('Ctrl Pts',(0.57491032546554,0.619819364819736,-4.39091169719878));
#66895=CARTESIAN_POINT('Ctrl Pts',(-0.212194185160404,0.818984569539605,
-4.35913850021));
#66896=CARTESIAN_POINT('Ctrl Pts',(-0.702026269447928,0.357599033471425,
-4.33266083605267));
#66897=CARTESIAN_POINT('Ctrl Pts',(-0.731631753435033,-0.13165937228476,
-4.31147870472682));
#66898=CARTESIAN_POINT('Ctrl Pts',(-0.532022195600957,-0.581964696773512,
-4.29029657340095));
#66899=CARTESIAN_POINT('Ctrl Pts',(-0.0376585147239648,-0.787402527562103,
-4.2691144420751));
#66900=CARTESIAN_POINT('Ctrl Pts',(0.423488095788453,-0.61187459781456,
-4.24793231074924));
#66901=CARTESIAN_POINT('Ctrl Pts',(0.665644086634238,-0.336192053156755,
-4.23204571225485));
#66902=CARTESIAN_POINT('Ctrl Pts',(0.743774045196498,0.0230847568156815,
-4.21615911376045));
#66903=CARTESIAN_POINT('Ctrl Pts',(0.611325637737408,0.497011926233411,
-4.1949769824346));
#66904=CARTESIAN_POINT('Ctrl Pts',(0.0369498026964951,0.844590219818537,
-4.16849931827727));
#66905=CARTESIAN_POINT('Ctrl Pts',(-0.691904104647108,0.486858097737258,
-4.13672612128848));
#66906=CARTESIAN_POINT('Ctrl Pts',(-0.766570576163524,-0.181899707242741,
-4.11024845713116));
#66907=CARTESIAN_POINT('Ctrl Pts',(-0.472412989765752,-0.573973152721816,
-4.08906632580531));
#66908=CARTESIAN_POINT('Ctrl Pts',(-0.0287661750624402,-0.787974004694965,
-4.06788419447945));
#66909=CARTESIAN_POINT('Ctrl Pts',(0.481023959960447,-0.624529306026845,
-4.04670206315358));
#66910=CARTESIAN_POINT('Ctrl Pts',(0.718877240868205,-0.192219154318652,
-4.02551993182774));
#66911=CARTESIAN_POINT('Ctrl Pts',(0.724982549969908,0.174663816848276,
-4.00963333333333));
#66912=CARTESIAN_POINT('Ctrl Pts',(0.551953773428615,0.499078919914592,
-3.99374673483894));
#66913=CARTESIAN_POINT('Ctrl Pts',(0.144204912207516,0.774561058579967,
-3.97256460351308));
#66914=CARTESIAN_POINT('Ctrl Pts',(-0.518584724903316,0.667658453424645,
-3.94608693935576));
#66915=CARTESIAN_POINT('Ctrl Pts',(-0.842531723549237,-0.0768270276205641,
-3.91431374236698));
#66916=CARTESIAN_POINT('Ctrl Pts',(-0.466519837019428,-0.634883606184656,
-3.88783607820964));
#66917=CARTESIAN_POINT('Ctrl Pts',(0.0114940687900335,-0.743294759383846,
-3.86665394688379));
#66918=CARTESIAN_POINT('Ctrl Pts',(0.4881715666929,-0.619208403023853,-3.84547181555793));
#66919=CARTESIAN_POINT('Ctrl Pts',(0.770922604173408,-0.164618475624371,
-3.82428968423208));
#66920=CARTESIAN_POINT('Ctrl Pts',(0.672355166352795,0.318859249519227,
-3.80310755290621));
#66921=CARTESIAN_POINT('Ctrl Pts',(0.439505996563567,0.60244636745652,-3.78722095441182));
#66922=CARTESIAN_POINT('Ctrl Pts',(0.0976141491142113,0.737701981966911,
-3.77133435591743));
#66923=CARTESIAN_POINT('Ctrl Pts',(-0.39150231822405,0.683714724865923,
-3.75015222459157));
#66924=CARTESIAN_POINT('Ctrl Pts',(-0.827470832334805,0.173176063494873,
-3.72367456043424));
#66925=CARTESIAN_POINT('Ctrl Pts',(-0.592435779693381,-0.603971807536539,
-3.69190136344546));
#66926=CARTESIAN_POINT('Ctrl Pts',(0.0554163053237293,-0.785905200923715,
-3.66542369928814));
#66927=CARTESIAN_POINT('Ctrl Pts',(0.489934337114234,-0.559091726160631,
-3.64424156796228));
#66928=CARTESIAN_POINT('Ctrl Pts',(0.772925944932573,-0.155935911684361,
-3.62305943663642));
#66929=CARTESIAN_POINT('Ctrl Pts',(0.694156298070137,0.373587925382995,
-3.60187730531056));
#66930=CARTESIAN_POINT('Ctrl Pts',(0.306048625366906,0.678282337700377,
-3.5806951739847));
#66931=CARTESIAN_POINT('Ctrl Pts',(-0.0550076813495416,0.743694360385653,
-3.56480857549031));
#66932=CARTESIAN_POINT('Ctrl Pts',(-0.403152557427834,0.625460431797726,
-3.54892197699592));
#66933=CARTESIAN_POINT('Ctrl Pts',(-0.741003855265364,0.267681110008094,
-3.52773984567005));
#66934=CARTESIAN_POINT('Ctrl Pts',(-0.742796613497877,-0.403672043010809,
-3.50126218151274));
#66935=CARTESIAN_POINT('Ctrl Pts',(-0.0605664975661023,-0.843856502453133,
-3.46948898452395));
#66936=CARTESIAN_POINT('Ctrl Pts',(0.550995435006661,-0.563135847142134,
-3.44301132036662));
#66937=CARTESIAN_POINT('Ctrl Pts',(0.735352835932997,-0.10897439896662,
-3.42182918904077));
#66938=CARTESIAN_POINT('Ctrl Pts',(0.690062547194971,0.381502563374796,
-3.4006470577149));
#66939=CARTESIAN_POINT('Ctrl Pts',(0.287236506823574,0.734109047274443,
-3.37946492638905));
#66940=CARTESIAN_POINT('Ctrl Pts',(-0.205820263132216,0.715101887851966,
-3.35828279506319));
#66941=CARTESIAN_POINT('Ctrl Pts',(-0.523358695669893,0.531227655853493,
-3.3423961965688));
#66942=CARTESIAN_POINT('Ctrl Pts',(-0.712172502830834,0.215738412242388,
-3.3265095980744));
#66943=CARTESIAN_POINT('Ctrl Pts',(-0.738070348497915,-0.275666557350466,
-3.30532746674855));
#66944=CARTESIAN_POINT('Ctrl Pts',(-0.304834682108662,-0.788526311492612,
-3.27884980259122));
#66945=CARTESIAN_POINT('Ctrl Pts',(0.500109323247009,-0.682387545432416,
-3.24707660560244));
#66946=CARTESIAN_POINT('Ctrl Pts',(0.784511015498687,-0.0725287411713208,
-3.22059894144511));
#66947=CARTESIAN_POINT('Ctrl Pts',(0.631024019531475,0.392973153942071,
-3.19941681011926));
#66948=CARTESIAN_POINT('Ctrl Pts',(0.278992727421459,0.737491412118594,
-3.17823467879339));
#66949=CARTESIAN_POINT('Ctrl Pts',(-0.256298242829113,0.745474422676672,
-3.15705254746754));
#66950=CARTESIAN_POINT('Ctrl Pts',(-0.619797254121925,0.411805845645958,
-3.13587041614168));
#66951=CARTESIAN_POINT('Ctrl Pts',(-0.742790701640324,0.0660993209764941,
-3.11998381764728));
#66952=CARTESIAN_POINT('Ctrl Pts',(-0.682470125197199,-0.296592758708842,
-3.1040972191529));
#66953=CARTESIAN_POINT('Ctrl Pts',(-0.384097027620931,-0.687902146781113,
-3.08291508782703));
#66954=CARTESIAN_POINT('Ctrl Pts',(0.278112223083316,-0.798342983124478,
-3.05643742366971));
#66955=CARTESIAN_POINT('Ctrl Pts',(0.82292396426287,-0.196362538183184,
-3.02466422668092));
#66956=CARTESIAN_POINT('Ctrl Pts',(0.644898747665643,0.452574366258134,
-2.9981865625236));
#66957=CARTESIAN_POINT('Ctrl Pts',(0.226568589229536,0.708015456977724,
-2.97700443119774));
#66958=CARTESIAN_POINT('Ctrl Pts',(-0.264771157858471,0.742715799528351,
-2.95582229987188));
#66959=CARTESIAN_POINT('Ctrl Pts',(-0.677932840683997,0.402278470297038,
-2.93464016854602));
#66960=CARTESIAN_POINT('Ctrl Pts',(-0.738987287045408,-0.0873526205132272,
-2.91345803722017));
#66961=CARTESIAN_POINT('Ctrl Pts',(-0.608937806846517,-0.43046706502338,
-2.89757143872577));
#66962=CARTESIAN_POINT('Ctrl Pts',(-0.328172420882141,-0.667858966008211,
-2.88168484023138));
#66963=CARTESIAN_POINT('Ctrl Pts',(0.152559894420231,-0.772958840293439,
-2.86050270890552));
#66964=CARTESIAN_POINT('Ctrl Pts',(0.728783846804567,-0.428453068572477,
-2.8340250447482));
#66965=CARTESIAN_POINT('Ctrl Pts',(0.754340852979042,0.383056098876796,
-2.80225184775941));
#66966=CARTESIAN_POINT('Ctrl Pts',(0.198560790390178,0.76242479252337,-2.77577418360209));
#66967=CARTESIAN_POINT('Ctrl Pts',(-0.285647023564601,0.686312604338228,
-2.75459205227623));
#66968=CARTESIAN_POINT('Ctrl Pts',(-0.682605017328055,0.394690910994047,
-2.73340992095037));
#66969=CARTESIAN_POINT('Ctrl Pts',(-0.777130127709657,-0.132248511327643,
-2.71222778962451));
#66970=CARTESIAN_POINT('Ctrl Pts',(-0.506701393044462,-0.544964575924034,
-2.69104565829866));
#66971=CARTESIAN_POINT('Ctrl Pts',(-0.185462906569463,-0.722295408377821,
-2.67515905980426));
#66972=CARTESIAN_POINT('Ctrl Pts',(0.182210114447717,-0.721479182304072,
-2.65927246130987));
#66973=CARTESIAN_POINT('Ctrl Pts',(0.616656528560847,-0.490382112190671,
-2.63809032998401));
#66974=CARTESIAN_POINT('Ctrl Pts',(0.832832487189643,0.145216994921211,
-2.61161266582669));
#66975=CARTESIAN_POINT('Ctrl Pts',(0.326979376809108,0.780286219602388,
-2.5798394688379));
#66976=CARTESIAN_POINT('Ctrl Pts',(-0.342216325821634,0.709651983775012,
-2.55336180468057));
#66977=CARTESIAN_POINT('Ctrl Pts',(-0.662003665385102,0.338186871361864,
-2.53217967335472));
#66978=CARTESIAN_POINT('Ctrl Pts',(-0.775779392941181,-0.14105622421774,
-2.51099754202885));
#66979=CARTESIAN_POINT('Ctrl Pts',(-0.506710052209743,-0.603875671915998,
-2.489815410703));
#66980=CARTESIAN_POINT('Ctrl Pts',(-0.0334190097720498,-0.74338136949423,
-2.46863327937714));
#66981=CARTESIAN_POINT('Ctrl Pts',(0.32622155852598,-0.670586788886994,
-2.45274668088275));
#66982=CARTESIAN_POINT('Ctrl Pts',(0.605930172637336,-0.431950647867195,
-2.43686008238835));
#66983=CARTESIAN_POINT('Ctrl Pts',(0.787459991398773,0.0254293554683121,
-2.4156779510625));
#66984=CARTESIAN_POINT('Ctrl Pts',(0.540770699778186,0.649819188385389,
-2.38920028690517));
#66985=CARTESIAN_POINT('Ctrl Pts',(-0.255899496701508,0.806397882529322,
-2.35742708991639));
#66986=CARTESIAN_POINT('Ctrl Pts',(-0.720229071880726,0.319355657148115,
-2.33094942575906));
#66987=CARTESIAN_POINT('Ctrl Pts',(-0.723499204724565,-0.170786749215974,
-2.3097672944332));
#66988=CARTESIAN_POINT('Ctrl Pts',(-0.49997884029397,-0.609714428368757,
-2.28858516310735));
#66989=CARTESIAN_POINT('Ctrl Pts',(0.00471063101971821,-0.788288471371872,
-2.26740303178148));
#66990=CARTESIAN_POINT('Ctrl Pts',(0.455758068365152,-0.588232329819882,
-2.24622090045563));
#66991=CARTESIAN_POINT('Ctrl Pts',(0.682749058575273,-0.299934775728751,
-2.23033430196123));
#66992=CARTESIAN_POINT('Ctrl Pts',(0.741458711415728,0.0630215484650262,
-2.21444770346684));
#66993=CARTESIAN_POINT('Ctrl Pts',(0.583733018808828,0.529146154597792,
-2.19326557214099));
#66994=CARTESIAN_POINT('Ctrl Pts',(-0.00849156494869494,0.845355440425599,
-2.16678790798366));
#66995=CARTESIAN_POINT('Ctrl Pts',(-0.717067869396526,0.448971901168643,
-2.13501471099488));
#66996=CARTESIAN_POINT('Ctrl Pts',(-0.755687642685574,-0.222832085721485,
-2.10853704683755));
#66997=CARTESIAN_POINT('Ctrl Pts',(-0.440885233565745,-0.598531054974189,
-2.08735491551169));
#66998=CARTESIAN_POINT('Ctrl Pts',(0.0136208320613828,-0.788381251576107,
-2.06617278418583));
#66999=CARTESIAN_POINT('Ctrl Pts',(0.513890851614579,-0.597776795107706,
-2.04499065285998));
#67000=CARTESIAN_POINT('Ctrl Pts',(0.728168238139964,-0.153309189840012,
-2.02380852153411));
#67001=CARTESIAN_POINT('Ctrl Pts',(0.714548566105297,0.213371725759888,
-2.00792192303973));
#67002=CARTESIAN_POINT('Ctrl Pts',(0.524335868445759,0.528019538811239,
-1.99203532454533));
#67003=CARTESIAN_POINT('Ctrl Pts',(0.102371900870404,0.781191323611233,
-1.97085319321948));
#67004=CARTESIAN_POINT('Ctrl Pts',(-0.553715085418805,0.638825118097339,
-1.94437552906215));
#67005=CARTESIAN_POINT('Ctrl Pts',(-0.837185592801576,-0.121993362792136,
-1.91260233207336));
#67006=CARTESIAN_POINT('Ctrl Pts',(-0.431727290682992,-0.659036795796866,
-1.88612466791603));
#67007=CARTESIAN_POINT('Ctrl Pts',(0.051421852550958,-0.741602997583657,
-1.86494253659018));
#67008=CARTESIAN_POINT('Ctrl Pts',(0.520742186510374,-0.592079471094158,
-1.84376040526432));
#67009=CARTESIAN_POINT('Ctrl Pts',(0.778655144391046,-0.122951495540993,
-1.82257827393846));
#67010=CARTESIAN_POINT('Ctrl Pts',(0.654248219366565,0.354530616704593,
-1.8013961426126));
#67011=CARTESIAN_POINT('Ctrl Pts',(0.406495651263466,0.625194715413342,
-1.78550954411821));
#67012=CARTESIAN_POINT('Ctrl Pts',(0.0578292558056736,0.741881738202362,
-1.76962294562382));
#67013=CARTESIAN_POINT('Ctrl Pts',(-0.427679173417961,0.661687550735103,
-1.74844081429796));
#67014=CARTESIAN_POINT('Ctrl Pts',(-0.835581541009314,0.12845783610561,
-1.72196315014064));
#67015=CARTESIAN_POINT('Ctrl Pts',(-0.559122471426269,-0.63493634271952,
-1.69018995315185));
#67016=CARTESIAN_POINT('Ctrl Pts',(0.0975704904356342,-0.781791501060753,
-1.66371228899453));
#67017=CARTESIAN_POINT('Ctrl Pts',(0.519271761113482,-0.53195493329317,
-1.64253015766867));
#67018=CARTESIAN_POINT('Ctrl Pts',(0.780188992423923,-0.114173819255057,
-1.62134802634281));
#67019=CARTESIAN_POINT('Ctrl Pts',(0.673076748697835,0.410351793592717,
-1.60016589501695));
#67020=CARTESIAN_POINT('Ctrl Pts',(0.269155730685218,0.69374915017214,-1.57898376369109));
#67021=CARTESIAN_POINT('Ctrl Pts',(-0.0948940615492358,0.73966361527357,
-1.5630971651967));
#67022=CARTESIAN_POINT('Ctrl Pts',(-0.436182013063224,0.602891356535583,
-1.54721056670231));
#67023=CARTESIAN_POINT('Ctrl Pts',(-0.754318177514541,0.227473025311658,
-1.52602843537645));
#67024=CARTESIAN_POINT('Ctrl Pts',(-0.720030068313977,-0.443006352162364,
-1.49955077121913));
#67025=CARTESIAN_POINT('Ctrl Pts',(-0.0151304330670991,-0.84589193597945,
-1.46777757423034));
#67026=CARTESIAN_POINT('Ctrl Pts',(0.580461954196043,-0.53271180901645,
-1.44129991007302));
#67027=CARTESIAN_POINT('Ctrl Pts',(0.740146482467141,-0.0692993321494254,
-1.42011777874716));
#67028=CARTESIAN_POINT('Ctrl Pts',(0.668563583570739,0.418034998087244,
-1.3989356474213));
#67029=CARTESIAN_POINT('Ctrl Pts',(0.247370688717346,0.748484232636805,
-1.37775351609544));
#67030=CARTESIAN_POINT('Ctrl Pts',(-0.24395216717569,0.703007845514929,
-1.35657138476958));
#67031=CARTESIAN_POINT('Ctrl Pts',(-0.551150415740897,0.502334914081758,
-1.34068478627519));
#67032=CARTESIAN_POINT('Ctrl Pts',(-0.722737105030778,0.177154772210434,
-1.32479818778079));
#67033=CARTESIAN_POINT('Ctrl Pts',(-0.722189601592419,-0.314931849016698,
-1.30361605645494));
#67034=CARTESIAN_POINT('Ctrl Pts',(-0.262019070115917,-0.803768582508686,
-1.27713839229761));
#67035=CARTESIAN_POINT('Ctrl Pts',(0.536057917164077,-0.654525787731523,
-1.24536519530883));
#67036=CARTESIAN_POINT('Ctrl Pts',(0.7872750510185,-0.0302645961231062,
-1.2188875311515));
#67037=CARTESIAN_POINT('Ctrl Pts',(0.608993942262501,0.426316304206648,
-1.19770539982565));
#67038=CARTESIAN_POINT('Ctrl Pts',(0.238957054659373,0.751418692162539,
-1.17652326849978));
#67039=CARTESIAN_POINT('Ctrl Pts',(-0.295989414350265,0.730623822999904,
-1.15534113717393));
#67040=CARTESIAN_POINT('Ctrl Pts',(-0.641031933583759,0.377903097170594,
-1.13415900584807));
#67041=CARTESIAN_POINT('Ctrl Pts',(-0.745269509057839,0.0260865012135712,
-1.11827240735367));
#67042=CARTESIAN_POINT('Ctrl Pts',(-0.665545155112125,-0.332839875633884,
-1.10238580885928));
#67043=CARTESIAN_POINT('Ctrl Pts',(-0.34657438647555,-0.707549351503058,
-1.08120367753342));
#67044=CARTESIAN_POINT('Ctrl Pts',(0.320613010413704,-0.782243711950361,
-1.0547260133761));
#67045=CARTESIAN_POINT('Ctrl Pts',(0.832287276052231,-0.151855152963071,
-1.02295281638731));
#67046=CARTESIAN_POINT('Ctrl Pts',(0.619645673454765,0.48657701456549,-0.996475152229989));
#67047=CARTESIAN_POINT('Ctrl Pts',(0.18819269753976,0.719168075999973,-0.975293020904133));
#67048=CARTESIAN_POINT('Ctrl Pts',(-0.304301838445365,0.727413854708367,
-0.954110889578274));
#67049=CARTESIAN_POINT('Ctrl Pts',(-0.698571515424613,0.36526530355274,
-0.932928758252416));
#67050=CARTESIAN_POINT('Ctrl Pts',(-0.733225138349833,-0.126939305249656,
-0.911746626926556));
#67051=CARTESIAN_POINT('Ctrl Pts',(-0.584924735273482,-0.462569130771008,
-0.895860028432164));
#67052=CARTESIAN_POINT('Ctrl Pts',(-0.291807705151121,-0.684529765254048,
-0.879973429937768));
#67053=CARTESIAN_POINT('Ctrl Pts',(0.193877972488015,-0.763643386640963,
-0.858791298611913));
#67054=CARTESIAN_POINT('Ctrl Pts',(0.750755654391034,-0.388669364275005,
-0.832313634454587));
#67055=CARTESIAN_POINT('Ctrl Pts',(0.732665519578818,0.423040581718017,
-0.800540437465801));
#67056=CARTESIAN_POINT('Ctrl Pts',(0.157301432367607,0.771993660029016,
-0.774062773308477));
#67057=CARTESIAN_POINT('Ctrl Pts',(-0.322116450716943,0.669970301652722,
-0.752880641982619));
#67058=CARTESIAN_POINT('Ctrl Pts',(-0.702829188003266,0.357437627360335,
-0.731698510656762));
#67059=CARTESIAN_POINT('Ctrl Pts',(-0.768900172839997,-0.173820103281627,
-0.710516379330902));
#67060=CARTESIAN_POINT('Ctrl Pts',(-0.47668300000339,-0.571407042463865,
-0.689334248005046));
#67061=CARTESIAN_POINT('Ctrl Pts',(-0.146379013782528,-0.731218388212433,
-0.673447649510651));
#67062=CARTESIAN_POINT('Ctrl Pts',(0.220718848884244,-0.710644725186344,
-0.657561051016257));
#67063=CARTESIAN_POINT('Ctrl Pts',(0.642118407188864,-0.45653460181011,
-0.6363789196904));
#67064=CARTESIAN_POINT('Ctrl Pts',(0.823825118811679,0.189763273491745,
-0.609901255533075));
#67065=CARTESIAN_POINT('Ctrl Pts',(0.28457458659541,0.796730442765568,-0.578128058544289));
#67066=CARTESIAN_POINT('Ctrl Pts',(-0.379858261997401,0.690235946123353,
-0.551650394386966));
#67067=CARTESIAN_POINT('Ctrl Pts',(-0.679221094819627,0.302122339919885,
-0.530468263061107));
#67068=CARTESIAN_POINT('Ctrl Pts',(-0.767078076405924,-0.182542484323307,
-0.50928613173525));
#67069=CARTESIAN_POINT('Ctrl Pts',(-0.473525765627643,-0.630233509741301,
-0.488104000409389));
#67070=CARTESIAN_POINT('Ctrl Pts',(0.00657830405987886,-0.744103053859658,
-0.466921869083533));
#67071=CARTESIAN_POINT('Ctrl Pts',(0.361787306164901,-0.652086835470523,
-0.451035270589137));
#67072=CARTESIAN_POINT('Ctrl Pts',(0.628267371514877,-0.398763844762359,
-0.435148672094745));
#67073=CARTESIAN_POINT('Ctrl Pts',(0.784955734091449,0.0677100869688686,
-0.413966540768886));
#67074=CARTESIAN_POINT('Ctrl Pts',(0.505067810210761,0.677941712115777,
-0.387488876611564));
#67075=CARTESIAN_POINT('Ctrl Pts',(-0.298864521600004,0.791479450126972,
-0.355715679622777));
#67076=CARTESIAN_POINT('Ctrl Pts',(-0.736351606015524,0.280191386843895,
-0.329238015465453));
#67077=CARTESIAN_POINT('Ctrl Pts',(-0.713274091724115,-0.209423283087674,
-0.308055884139594));
#67078=CARTESIAN_POINT('Ctrl Pts',(-0.466494711648086,-0.635695014837649,
-0.286873752813737));
#67079=CARTESIAN_POINT('Ctrl Pts',(0.0470746703232514,-0.786910562942938,
-0.265691621487877));
#67080=CARTESIAN_POINT('Ctrl Pts',(0.486700370550275,-0.562872340213963,
-0.244509490162019));
#67081=CARTESIAN_POINT('Ctrl Pts',(0.69790273612906,-0.262847524723207,
-0.228622891667627));
#67082=CARTESIAN_POINT('Ctrl Pts',(0.736960633613606,0.10284341760348,-0.212736293173231));
#67083=CARTESIAN_POINT('Ctrl Pts',(0.554539603465115,0.559605906724123,
-0.191554161847375));
#67084=CARTESIAN_POINT('Ctrl Pts',(-0.0540867686931964,0.843978018413933,
-0.165076497690051));
#67085=CARTESIAN_POINT('Ctrl Pts',(-0.739847523655629,0.409263047681452,
-0.133303300701265));
#67086=CARTESIAN_POINT('Ctrl Pts',(-0.743144735960948,-0.262238058905764,
-0.10682563654394));
#67087=CARTESIAN_POINT('Ctrl Pts',(-0.407377385049017,-0.622546633323945,
-0.0856435052180836));
#67088=CARTESIAN_POINT('Ctrl Pts',(-0.0613458632290381,-0.74305434807241,
-0.0697569067236874));
#67089=CARTESIAN_POINT('Ctrl Pts',(0.302742394164461,-0.680954303180219,
-0.0538703082292963));
#67090=CARTESIAN_POINT('Ctrl Pts',(0.494975304259394,-0.529271880382184,
-0.043279242566365));
#67091=CARTESIAN_POINT('Ctrl Pts',(0.567325265044049,-0.434889340047722,
-0.0379837097349007));
#67092=CARTESIAN_POINT('Ctrl Pts',(-0.325579286441984,0.678938089483158,
-11.9309162902651));
#67093=CARTESIAN_POINT('Ctrl Pts',(-0.438530190559174,0.624773394152179,
-11.9256207574336));
#67094=CARTESIAN_POINT('Ctrl Pts',(-0.636487869789445,0.459419899431822,
-11.9150296917707));
#67095=CARTESIAN_POINT('Ctrl Pts',(-0.779277659860866,0.0975214801954652,
-11.8991430932763));
#67096=CARTESIAN_POINT('Ctrl Pts',(-0.729912798382054,-0.285270244336759,
-11.8832564947819));
#67097=CARTESIAN_POINT('Ctrl Pts',(-0.431119590957509,-0.709362437639476,
-11.8620743634561));
#67098=CARTESIAN_POINT('Ctrl Pts',(0.261835732470835,-0.851244765286553,
-11.8355966992988));
#67099=CARTESIAN_POINT('Ctrl Pts',(0.85834437572654,-0.238354668512496,
-11.8038235023099));
#67100=CARTESIAN_POINT('Ctrl Pts',(0.69686701284205,0.45059533067605,-11.7773458381526));
#67101=CARTESIAN_POINT('Ctrl Pts',(0.265463729879274,0.737472858364993,
-11.7561637068268));
#67102=CARTESIAN_POINT('Ctrl Pts',(-0.119972716722838,0.776326956521568,
-11.7402771083324));
#67103=CARTESIAN_POINT('Ctrl Pts',(-0.474958785797699,0.623512435543155,
-11.724390509838));
#67104=CARTESIAN_POINT('Ctrl Pts',(-0.801031350365818,0.218779261424542,
-11.7032083785121));
#67105=CARTESIAN_POINT('Ctrl Pts',(-0.756257517900422,-0.34336885159689,
-11.6820262471863));
#67106=CARTESIAN_POINT('Ctrl Pts',(-0.370210901362501,-0.689995813217701,
-11.6608441158604));
#67107=CARTESIAN_POINT('Ctrl Pts',(0.129533749630415,-0.81971580735925,
-11.6396619845346));
#67108=CARTESIAN_POINT('Ctrl Pts',(0.751265829807233,-0.479334713936513,
-11.6131843203772));
#67109=CARTESIAN_POINT('Ctrl Pts',(0.808154513003672,0.373993162759316,
-11.5814111233884));
#67110=CARTESIAN_POINT('Ctrl Pts',(0.239629116940131,0.794551604670445,
-11.5549334592311));
#67111=CARTESIAN_POINT('Ctrl Pts',(-0.275152955319875,0.73394666811328,
-11.5337513279053));
#67112=CARTESIAN_POINT('Ctrl Pts',(-0.593954211107484,0.514042981534784,
-11.5178647294109));
#67113=CARTESIAN_POINT('Ctrl Pts',(-0.765663149550031,0.167770532262155,
-11.5019781309165));
#67114=CARTESIAN_POINT('Ctrl Pts',(-0.752148512370767,-0.351798689683568,
-11.4807959995906));
#67115=CARTESIAN_POINT('Ctrl Pts',(-0.354140489117332,-0.751277403168843,
-11.4596138682647));
#67116=CARTESIAN_POINT('Ctrl Pts',(0.164502456835433,-0.765565519913649,
-11.4384317369389));
#67117=CARTESIAN_POINT('Ctrl Pts',(0.62937193641715,-0.540925780748815,
-11.417249605613));
#67118=CARTESIAN_POINT('Ctrl Pts',(0.882907902300928,0.120989182847097,
-11.3907719414557));
#67119=CARTESIAN_POINT('Ctrl Pts',(0.373861710521524,0.808214967858265,
-11.3589987444669));
#67120=CARTESIAN_POINT('Ctrl Pts',(-0.331711379690762,0.760724410311425,
-11.3325210803096));
#67121=CARTESIAN_POINT('Ctrl Pts',(-0.684841401373326,0.381286484920216,
-11.3113389489838));
#67122=CARTESIAN_POINT('Ctrl Pts',(-0.785473309452427,0.00730113817008764,
-11.2954523504893));
#67123=CARTESIAN_POINT('Ctrl Pts',(-0.69218813210121,-0.367780734196896,
-11.279565751995));
#67124=CARTESIAN_POINT('Ctrl Pts',(-0.345542913605394,-0.755042893881491,
-11.2583836206691));
#67125=CARTESIAN_POINT('Ctrl Pts',(0.216418598618142,-0.801870440168425,
-11.2372014893433));
#67126=CARTESIAN_POINT('Ctrl Pts',(0.620972963907686,-0.477015944868456,
-11.2160193580174));
#67127=CARTESIAN_POINT('Ctrl Pts',(0.82987111893074,-0.00486321422972745,
-11.1948372266915));
#67128=CARTESIAN_POINT('Ctrl Pts',(0.594621657647541,0.663769413694489,
-11.1683595625342));
#67129=CARTESIAN_POINT('Ctrl Pts',(-0.238245957352548,0.858034310357582,
-11.1365863655454));
#67130=CARTESIAN_POINT('Ctrl Pts',(-0.745284156508827,0.365082993917505,
-11.1101087013881));
#67131=CARTESIAN_POINT('Ctrl Pts',(-0.768806557073455,-0.152720683283362,
-11.0889265700622));
#67132=CARTESIAN_POINT('Ctrl Pts',(-0.603406952189243,-0.502913189569635,
-11.0730399715678));
#67133=CARTESIAN_POINT('Ctrl Pts',(-0.289495688199805,-0.728408762470549,
-11.0571533730735));
#67134=CARTESIAN_POINT('Ctrl Pts',(0.225409211463697,-0.799174802017602,
-11.0359712417476));
#67135=CARTESIAN_POINT('Ctrl Pts',(0.684045040627252,-0.471079181211703,
-11.0147891104217));
#67136=CARTESIAN_POINT('Ctrl Pts',(0.782097317996387,0.038411180330575,
-10.9936069790959));
#67137=CARTESIAN_POINT('Ctrl Pts',(0.635668359101772,0.533512382338015,
-10.97242484777));
#67138=CARTESIAN_POINT('Ctrl Pts',(0.0235224284446957,0.890848722095813,
-10.9459471836127));
#67139=CARTESIAN_POINT('Ctrl Pts',(-0.737039470499595,0.499756773719366,
-10.9141739866239));
#67140=CARTESIAN_POINT('Ctrl Pts',(-0.804386100341556,-0.204198599320718,
-10.8876963224666));
#67141=CARTESIAN_POINT('Ctrl Pts',(-0.487113192994437,-0.614091089752501,
-10.8665141911407));
#67142=CARTESIAN_POINT('Ctrl Pts',(-0.134349165685502,-0.773932767023663,
-10.8506275926463));
#67143=CARTESIAN_POINT('Ctrl Pts',(0.250886222352188,-0.742592204486319,
-10.8347409941519));
#67144=CARTESIAN_POINT('Ctrl Pts',(0.689152575330391,-0.463204495561479,
-10.8135588628261));
#67145=CARTESIAN_POINT('Ctrl Pts',(0.826327097284044,0.0837659887530412,
-10.7923767315002));
#67146=CARTESIAN_POINT('Ctrl Pts',(0.571241822611821,0.535569242666811,
-10.7711946001744));
#67147=CARTESIAN_POINT('Ctrl Pts',(0.139130052178819,0.818139690671364,
-10.7500124688485));
#67148=CARTESIAN_POINT('Ctrl Pts',(-0.558764499776105,0.694224015782814,
-10.7235348046912));
#67149=CARTESIAN_POINT('Ctrl Pts',(-0.885283474044109,-0.0962142636885308,
-10.6917616077024));
#67150=CARTESIAN_POINT('Ctrl Pts',(-0.480907240447861,-0.676359588142325,
-10.6652839435451));
#67151=CARTESIAN_POINT('Ctrl Pts',(0.0262601526305759,-0.783388494737106,
-10.6441018122192));
#67152=CARTESIAN_POINT('Ctrl Pts',(0.398607551650078,-0.6768557054209,-10.6282152137248));
#67153=CARTESIAN_POINT('Ctrl Pts',(0.671942037449668,-0.403585154630335,
-10.6123286152304));
#67154=CARTESIAN_POINT('Ctrl Pts',(0.825122316493558,0.0930743768025403,
-10.5911464839046));
#67155=CARTESIAN_POINT('Ctrl Pts',(0.575592809069977,0.598770515911213,
-10.5699643525787));
#67156=CARTESIAN_POINT('Ctrl Pts',(0.0886932242196915,0.778000736226575,
-10.5487822212528));
#67157=CARTESIAN_POINT('Ctrl Pts',(-0.423581063004594,0.713644735099345,
-10.527600089927));
#67158=CARTESIAN_POINT('Ctrl Pts',(-0.875292768904854,0.167413616538596,
-10.5011224257697));
#67159=CARTESIAN_POINT('Ctrl Pts',(-0.612470397060775,-0.646424030089341,
-10.4693492287809));
#67160=CARTESIAN_POINT('Ctrl Pts',(0.0712999359732703,-0.826831533939921,
-10.4428715646235));
#67161=CARTESIAN_POINT('Ctrl Pts',(0.527143687336232,-0.580091942888548,
-10.4216894332977));
#67162=CARTESIAN_POINT('Ctrl Pts',(0.741979196074009,-0.2578536383041,-10.4058028348033));
#67163=CARTESIAN_POINT('Ctrl Pts',(0.773409877771076,0.12737440753987,-10.3899162363089));
#67164=CARTESIAN_POINT('Ctrl Pts',(0.568648728658316,0.605085366033717,
-10.368734104983));
#67165=CARTESIAN_POINT('Ctrl Pts',(0.0510960087729735,0.828988787900728,
-10.3475519736572));
#67166=CARTESIAN_POINT('Ctrl Pts',(-0.436039500666917,0.650400789859394,
-10.3263698423313));
#67167=CARTESIAN_POINT('Ctrl Pts',(-0.784829244580027,0.269727235782853,
-10.3051877110055));
#67168=CARTESIAN_POINT('Ctrl Pts',(-0.775515720372333,-0.439021773668505,
-10.2787100468482));
#67169=CARTESIAN_POINT('Ctrl Pts',(-0.0483551498041389,-0.889182654711702,
-10.2469368498594));
#67170=CARTESIAN_POINT('Ctrl Pts',(0.589595553257777,-0.584047215527897,
-10.220459185702));
#67171=CARTESIAN_POINT('Ctrl Pts',(0.777308002135367,-0.100893008275974,
-10.1992770543762));
#67172=CARTESIAN_POINT('Ctrl Pts',(0.732451906686202,0.28378835526681,-10.1833904558818));
#67173=CARTESIAN_POINT('Ctrl Pts',(0.507029774768671,0.597752361959393,
-10.1675038573874));
#67174=CARTESIAN_POINT('Ctrl Pts',(0.0417153609279727,0.829306641391184,
-10.1463217260615));
#67175=CARTESIAN_POINT('Ctrl Pts',(-0.497702991792484,0.664924766073919,
-10.1251395947357));
#67176=CARTESIAN_POINT('Ctrl Pts',(-0.753383830165404,0.213458281724755,
-10.1039574634098));
#67177=CARTESIAN_POINT('Ctrl Pts',(-0.772798222234306,-0.302477491034639,
-10.082775332084));
#67178=CARTESIAN_POINT('Ctrl Pts',(-0.306889151096186,-0.836650344671608,
-10.0562976679267));
#67179=CARTESIAN_POINT('Ctrl Pts',(0.538758694853179,-0.709029676863268,
-10.0245244709379));
#67180=CARTESIAN_POINT('Ctrl Pts',(0.827468696130943,-0.0634793140368794,
-9.99804680678052));
#67181=CARTESIAN_POINT('Ctrl Pts',(0.657770354064988,0.42629249420541,-9.97686467545469));
#67182=CARTESIAN_POINT('Ctrl Pts',(0.374557037310136,0.690455394645263,
-9.96097807696027));
#67183=CARTESIAN_POINT('Ctrl Pts',(-0.000503001884737476,0.783828313930485,
-9.94509147846589));
#67184=CARTESIAN_POINT('Ctrl Pts',(-0.505058598658514,0.659094445974152,
-9.92390934714003));
#67185=CARTESIAN_POINT('Ctrl Pts',(-0.809785307998288,0.184610312625709,
-9.90272721581418));
#67186=CARTESIAN_POINT('Ctrl Pts',(-0.71240497240588,-0.325008905851757,
-9.88154508448831));
#67187=CARTESIAN_POINT('Ctrl Pts',(-0.393210171172526,-0.730818367419422,
-9.86036295316246));
#67188=CARTESIAN_POINT('Ctrl Pts',(0.307699535168253,-0.836352644735999,
-9.83388528900513));
#67189=CARTESIAN_POINT('Ctrl Pts',(0.869629008692517,-0.191649161733625,
-9.80211209201635));
#67190=CARTESIAN_POINT('Ctrl Pts',(0.671782528753483,0.487280515154063,
-9.77563442785901));
#67191=CARTESIAN_POINT('Ctrl Pts',(0.225385044131932,0.750725456598015,
-9.75445229653317));
#67192=CARTESIAN_POINT('Ctrl Pts',(-0.161484038614348,0.768729166524916,
-9.73856569803877));
#67193=CARTESIAN_POINT('Ctrl Pts',(-0.507796541602976,0.597101122981744,
-9.72267909954437));
#67194=CARTESIAN_POINT('Ctrl Pts',(-0.81161741215718,0.175404826262443,
-9.70149696821852));
#67195=CARTESIAN_POINT('Ctrl Pts',(-0.736718858145562,-0.383508196301391,
-9.68031483689266));
#67196=CARTESIAN_POINT('Ctrl Pts',(-0.332593224809995,-0.708895888267146,
-9.6591327055668));
#67197=CARTESIAN_POINT('Ctrl Pts',(0.173395859510444,-0.811568605094942,
-9.63795057424095));
#67198=CARTESIAN_POINT('Ctrl Pts',(0.775940670895153,-0.438270265418998,
-9.61147291008361));
#67199=CARTESIAN_POINT('Ctrl Pts',(0.786887793255583,0.416883214795328,
-9.57969971309484));
#67200=CARTESIAN_POINT('Ctrl Pts',(0.196584251865598,0.806280781307404,
-9.5532220489375));
#67201=CARTESIAN_POINT('Ctrl Pts',(-0.314197532506346,0.718099603028419,
-9.53203991761166));
#67202=CARTESIAN_POINT('Ctrl Pts',(-0.620720339747097,0.481381227321487,
-9.51615331911726));
#67203=CARTESIAN_POINT('Ctrl Pts',(-0.773572719280374,0.126381670803847,
-9.50026672062285));
#67204=CARTESIAN_POINT('Ctrl Pts',(-0.732156077208528,-0.391710550533803,
-9.47908458929703));
#67205=CARTESIAN_POINT('Ctrl Pts',(-0.313255387818101,-0.769223163055156,
-9.45790245797111));
#67206=CARTESIAN_POINT('Ctrl Pts',(0.205405969347057,-0.755618965714978,
-9.43672032664531));
#67207=CARTESIAN_POINT('Ctrl Pts',(0.657531634595437,-0.506321907858398,
-9.41553819531941));
#67208=CARTESIAN_POINT('Ctrl Pts',(0.875130171604578,0.168261501975349,
-9.38906053116212));
#67209=CARTESIAN_POINT('Ctrl Pts',(0.329888290337415,0.827138277346046,
-9.35728733417332));
#67210=CARTESIAN_POINT('Ctrl Pts',(-0.372113105932665,0.741799098665116,
-9.33080967001599));
#67211=CARTESIAN_POINT('Ctrl Pts',(-0.704341991722376,0.343932388703371,
-9.30962753869014));
#67212=CARTESIAN_POINT('Ctrl Pts',(-0.784730646335707,-0.0349204652723357,
-9.29374094019574));
#67213=CARTESIAN_POINT('Ctrl Pts',(-0.671423503221182,-0.404447225299171,
-9.27785434170135));
#67214=CARTESIAN_POINT('Ctrl Pts',(-0.304467864204802,-0.772521194828622,
-9.25667221037549));
#67215=CARTESIAN_POINT('Ctrl Pts',(0.259198098613203,-0.789081464902673,
-9.23549007904963));
#67216=CARTESIAN_POINT('Ctrl Pts',(0.645710311728348,-0.442955784384013,
-9.21430794772378));
#67217=CARTESIAN_POINT('Ctrl Pts',(0.828933287182104,0.0397407885250041,
-9.19312581639791));
#67218=CARTESIAN_POINT('Ctrl Pts',(0.558091688915222,0.694765008519724,
-9.1666481522406));
#67219=CARTESIAN_POINT('Ctrl Pts',(-0.2840121426244,0.84399118288915,-9.13487495525182));
#67220=CARTESIAN_POINT('Ctrl Pts',(-0.763826635834081,0.324504139846667,
-9.10839729109447));
#67221=CARTESIAN_POINT('Ctrl Pts',(-0.759488462810364,-0.193815386800432,
-9.08721515976864));
#67222=CARTESIAN_POINT('Ctrl Pts',(-0.575508644139153,-0.534613343187773,
-9.07132856127422));
#67223=CARTESIAN_POINT('Ctrl Pts',(-0.249932936789059,-0.742913592443966,
-9.05544196277984));
#67224=CARTESIAN_POINT('Ctrl Pts',(0.268030857269164,-0.785906569729782,
-9.03425983145398));
#67225=CARTESIAN_POINT('Ctrl Pts',(0.708372208573284,-0.433638128741758,
-9.01307770012811));
#67226=CARTESIAN_POINT('Ctrl Pts',(0.778902969892766,0.0803853039044273,
-8.99189556880227));
#67227=CARTESIAN_POINT('Ctrl Pts',(0.606079043113628,0.566902035954701,
-8.9707134374764));
#67228=CARTESIAN_POINT('Ctrl Pts',(-0.0243854516630399,0.890825516050617,
-8.94423577331908));
#67229=CARTESIAN_POINT('Ctrl Pts',(-0.762831184016125,0.459426380005858,
-8.91246257633029));
#67230=CARTESIAN_POINT('Ctrl Pts',(-0.792250188295256,-0.247130948149693,
-8.88598491217298));
#67231=CARTESIAN_POINT('Ctrl Pts',(-0.453408271228742,-0.639381004475433,
-8.86480278084711));
#67232=CARTESIAN_POINT('Ctrl Pts',(-0.0925641602466446,-0.78003429567624,
-8.84891618235272));
#67233=CARTESIAN_POINT('Ctrl Pts',(0.29043032497467,-0.728036609701126,
-8.83302958385833));
#67234=CARTESIAN_POINT('Ctrl Pts',(0.713049180021141,-0.425500345081005,
-8.81184745253247));
#67235=CARTESIAN_POINT('Ctrl Pts',(0.820631485246796,0.128051466212941,
-8.7906653212066));
#67236=CARTESIAN_POINT('Ctrl Pts',(0.541635069226991,0.565493665194448,
-8.76948318988076));
#67237=CARTESIAN_POINT('Ctrl Pts',(0.0949624741010667,0.824434262621175,
-8.74830105855488));
#67238=CARTESIAN_POINT('Ctrl Pts',(-0.595264423535308,0.66319304608299,
-8.72182339439759));
#67239=CARTESIAN_POINT('Ctrl Pts',(-0.878833703135999,-0.143650047633126,
-8.69005019740877));
#67240=CARTESIAN_POINT('Ctrl Pts',(-0.44386499970157,-0.701226018076312,
-8.66357253325146));
#67241=CARTESIAN_POINT('Ctrl Pts',(0.0683212220377295,-0.780845272715357,
-8.6423904019256));
#67242=CARTESIAN_POINT('Ctrl Pts',(0.434405538413424,-0.654456610012488,
-8.6265038034312));
#67243=CARTESIAN_POINT('Ctrl Pts',(0.692659589757795,-0.366892043313242,
-8.61061720493682));
#67244=CARTESIAN_POINT('Ctrl Pts',(0.818928215962582,0.13728165898334,-8.58943507361095));
#67245=CARTESIAN_POINT('Ctrl Pts',(0.542583354747329,0.628837431876301,
-8.56825294228509));
#67246=CARTESIAN_POINT('Ctrl Pts',(0.0467555812598027,0.781642852722799,
-8.54707081095925));
#67247=CARTESIAN_POINT('Ctrl Pts',(-0.461319991798783,0.689850411348641,
-8.52588867963336));
#67248=CARTESIAN_POINT('Ctrl Pts',(-0.883024702170366,0.120133782328678,
-8.49941101547607));
#67249=CARTESIAN_POINT('Ctrl Pts',(-0.576846771236841,-0.678403874153413,
-8.46763781848726));
#67250=CARTESIAN_POINT('Ctrl Pts',(0.115630535354455,-0.821805114172988,
-8.44116015432995));
#67251=CARTESIAN_POINT('Ctrl Pts',(0.557555887226266,-0.550925187227795,
-8.41997802300409));
#67252=CARTESIAN_POINT('Ctrl Pts',(0.754763984144613,-0.217607340021979,
-8.4040914245097));
#67253=CARTESIAN_POINT('Ctrl Pts',(0.765447231361476,0.168753117692842,
-8.3882048260153));
#67254=CARTESIAN_POINT('Ctrl Pts',(0.535309950887092,0.634769984540963,
-8.36702269468945));
#67255=CARTESIAN_POINT('Ctrl Pts',(0.00647261493553671,0.830536764889757,
-8.34584056336357));
#67256=CARTESIAN_POINT('Ctrl Pts',(-0.470361719928608,0.626028342822735,
-8.32465843203774));
#67257=CARTESIAN_POINT('Ctrl Pts',(-0.798190196393674,0.227161033745103,
-8.30347630071186));
#67258=CARTESIAN_POINT('Ctrl Pts',(-0.750802213668294,-0.480063314835082,
-8.27699863655455));
#67259=CARTESIAN_POINT('Ctrl Pts',(-0.000500919816292827,-0.890496357674791,
-8.24522543956576));
#67260=CARTESIAN_POINT('Ctrl Pts',(0.620130063974467,-0.551518603622994,
-8.21874777540842));
#67261=CARTESIAN_POINT('Ctrl Pts',(0.781606731650396,-0.0589749636832082,
-8.19756564408259));
#67262=CARTESIAN_POINT('Ctrl Pts',(0.716142816035578,0.322739977743579,
-8.18167904558817));
#67263=CARTESIAN_POINT('Ctrl Pts',(0.474174110526119,0.624136196384063,
-8.16579244709379));
#67264=CARTESIAN_POINT('Ctrl Pts',(-0.00291155903197221,0.830350046436369,
-8.14461031576793));
#67265=CARTESIAN_POINT('Ctrl Pts',(-0.532716619424106,0.637217557798746,
-8.12342818444207));
#67266=CARTESIAN_POINT('Ctrl Pts',(-0.763766347841342,0.172663254622042,
-8.10224605311622));
#67267=CARTESIAN_POINT('Ctrl Pts',(-0.755426482980161,-0.343570303843829,
-8.08106392179035));
#67268=CARTESIAN_POINT('Ctrl Pts',(-0.261484402131578,-0.851933481993487,
-8.05458625763304));
#67269=CARTESIAN_POINT('Ctrl Pts',(0.57608317826944,-0.679052417466952,
-8.02281306064424));
#67270=CARTESIAN_POINT('Ctrl Pts',(0.829684344049591,-0.0189197152789447,
-7.99633539648693));
#67271=CARTESIAN_POINT('Ctrl Pts',(0.633911058491592,0.461024835800324,
-7.97515326516106));
#67272=CARTESIAN_POINT('Ctrl Pts',(0.336910971005782,0.70958623423037,-7.95926666666668));
#67273=CARTESIAN_POINT('Ctrl Pts',(-0.0426249265764459,0.782668636374523,
-7.94338006817227));
#67274=CARTESIAN_POINT('Ctrl Pts',(-0.539748277997935,0.631000374953247,
-7.92219793684641));
#67275=CARTESIAN_POINT('Ctrl Pts',(-0.818536045016483,0.14082597624878,
-7.90101580552057));
#67276=CARTESIAN_POINT('Ctrl Pts',(-0.69390967239051,-0.362823648835728,
-7.8798336741947));
#67277=CARTESIAN_POINT('Ctrl Pts',(-0.35336805911191,-0.750893294463733,
-7.85865154286885));
#67278=CARTESIAN_POINT('Ctrl Pts',(0.352200193822944,-0.818608437392834,
-7.83217387871152));
#67279=CARTESIAN_POINT('Ctrl Pts',(0.878671535674212,-0.144638675148288,
-7.80040068172274));
#67280=CARTESIAN_POINT('Ctrl Pts',(0.644625511028497,0.522677737155969,
-7.77392301756541));
#67281=CARTESIAN_POINT('Ctrl Pts',(0.184715642675801,0.761752755592991,
-7.75274088623955));
#67282=CARTESIAN_POINT('Ctrl Pts',(-0.202561919981265,0.758940244529698,
-7.73685428774516));
#67283=CARTESIAN_POINT('Ctrl Pts',(-0.539150765694184,0.568949497390918,
-7.72096768925077));
#67284=CARTESIAN_POINT('Ctrl Pts',(-0.819870802226295,0.131535335365389,
-7.6997855579249));
#67285=CARTESIAN_POINT('Ctrl Pts',(-0.71504469329701,-0.422545026198905,
-7.67860342659905));
#67286=CARTESIAN_POINT('Ctrl Pts',(-0.294016811499463,-0.725744960814242,
-7.65742129527319));
#67287=CARTESIAN_POINT('Ctrl Pts',(0.216758704089238,-0.801077642349773,
-7.63623916394733));
#67288=CARTESIAN_POINT('Ctrl Pts',(0.798371908626541,-0.395938184336486,
-7.60976149979001));
#67289=CARTESIAN_POINT('Ctrl Pts',(0.76334757188336,0.458567877693707,-7.57798830280121));
#67290=CARTESIAN_POINT('Ctrl Pts',(0.152970944928233,0.815680057617568,
-7.5515106386439));
#67291=CARTESIAN_POINT('Ctrl Pts',(-0.352333925525334,0.700177073479672,
-7.53032850731803));
#67292=CARTESIAN_POINT('Ctrl Pts',(-0.645692641308453,0.447328334842996,
-7.51444190882366));
#67293=CARTESIAN_POINT('Ctrl Pts',(-0.779246597900674,0.0846275273786758,
-7.49855531032925));
#67294=CARTESIAN_POINT('Ctrl Pts',(-0.710047714097925,-0.430490325672003,
-7.4773731790034));
#67295=CARTESIAN_POINT('Ctrl Pts',(-0.271464952000793,-0.784945853172596,
-7.45619104767753));
#67296=CARTESIAN_POINT('Ctrl Pts',(0.245715845237475,-0.74348863944973,
-7.43500891635168));
#67297=CARTESIAN_POINT('Ctrl Pts',(0.683791046352098,-0.470254749896074,
-7.41382678502581));
#67298=CARTESIAN_POINT('Ctrl Pts',(0.864823279746207,0.215047541508085,
-7.3873491208685));
#67299=CARTESIAN_POINT('Ctrl Pts',(0.284961482266343,0.843671125248044,
-7.35557592387971));
#67300=CARTESIAN_POINT('Ctrl Pts',(-0.411439412244053,0.720729960831034,
-7.32909825972239));
#67301=CARTESIAN_POINT('Ctrl Pts',(-0.721807007321595,0.305584314852858,
-7.30791612839652));
#67302=CARTESIAN_POINT('Ctrl Pts',(-0.781720082795018,-0.0770411471114446,
-7.29202952990214));
#67303=CARTESIAN_POINT('Ctrl Pts',(-0.64871843548489,-0.439944849034556,
-7.27614293140773));
#67304=CARTESIAN_POINT('Ctrl Pts',(-0.262512891480941,-0.787766880872249,
-7.25496080008189));
#67305=CARTESIAN_POINT('Ctrl Pts',(0.301228506546843,-0.774012015036721,
-7.23377866875602));
#67306=CARTESIAN_POINT('Ctrl Pts',(0.668581532841351,-0.407615465279578,
-7.21259653743016));
#67307=CARTESIAN_POINT('Ctrl Pts',(0.825599807570513,0.0842299389210877,
-7.19141440610431));
#67308=CARTESIAN_POINT('Ctrl Pts',(0.519948814544762,0.723752706767411,
-7.16493674194698));
#67309=CARTESIAN_POINT('Ctrl Pts',(-0.328957522291289,0.82750888966869,
-7.1331635449582));
#67310=CARTESIAN_POINT('Ctrl Pts',(-0.780161627919481,0.282987456805527,
-7.10668588080087));
#67311=CARTESIAN_POINT('Ctrl Pts',(-0.747975418785531,-0.234349956678595,
-7.08550374947501));
#67312=CARTESIAN_POINT('Ctrl Pts',(-0.545947094812301,-0.564768444461357,
-7.06961715098063));
#67313=CARTESIAN_POINT('Ctrl Pts',(-0.209647869942482,-0.755271374645289,
-7.05373055248622));
#67314=CARTESIAN_POINT('Ctrl Pts',(0.309877883978987,-0.770367038374293,
-7.03254842116037));
#67315=CARTESIAN_POINT('Ctrl Pts',(0.730652154624641,-0.394943846033858,
-7.01136628983451));
#67316=CARTESIAN_POINT('Ctrl Pts',(0.773457563384284,0.122127110975526,
-6.99018415850865));
#67317=CARTESIAN_POINT('Ctrl Pts',(0.574738136264083,0.59865332171031,-6.96900202718279));
#67318=CARTESIAN_POINT('Ctrl Pts',(-0.0722228569131348,0.888227791300737,
-6.94252436302547));
#67319=CARTESIAN_POINT('Ctrl Pts',(-0.786418287183742,0.417768227053888,
-6.91075116603668));
#67320=CARTESIAN_POINT('Ctrl Pts',(-0.777824643889002,-0.289349079393862,
-6.88427350187936));
#67321=CARTESIAN_POINT('Ctrl Pts',(-0.418392982781744,-0.662823084436399,
-6.8630913705535));
#67322=CARTESIAN_POINT('Ctrl Pts',(-0.0505116409593437,-0.783881496350488,
-6.84720477205911));
#67323=CARTESIAN_POINT('Ctrl Pts',(0.329135073210841,-0.711376962174498,
-6.83131817356472));
#67324=CARTESIAN_POINT('Ctrl Pts',(0.734885046197271,-0.386566482857896,
-6.81013604223886));
#67325=CARTESIAN_POINT('Ctrl Pts',(0.812564217849937,0.171966870196172,
-6.788953910913));
#67326=CARTESIAN_POINT('Ctrl Pts',(0.510462970451474,0.593783790105791,
-6.76777177958714));
#67327=CARTESIAN_POINT('Ctrl Pts',(0.0505204509556357,0.828346189042659,
-6.74658964826128));
#67328=CARTESIAN_POINT('Ctrl Pts',(-0.630044011076097,0.630245423945558,
-6.72011198410397));
#67329=CARTESIAN_POINT('Ctrl Pts',(-0.869844070319895,-0.190670677634717,
-6.68833878711516));
#67330=CARTESIAN_POINT('Ctrl Pts',(-0.405539972658642,-0.724065878853271,
-6.66186112295786));
#67331=CARTESIAN_POINT('Ctrl Pts',(0.110184840553053,-0.776045378985607,
-6.64067899163198));
#67332=CARTESIAN_POINT('Ctrl Pts',(0.46894807716623,-0.63016611073218,-6.6247923931376));
#67333=CARTESIAN_POINT('Ctrl Pts',(0.711375330090743,-0.329138600511838,
-6.6089057946432));
#67334=CARTESIAN_POINT('Ctrl Pts',(0.810367382881666,0.181092192311117,
-6.58772366331735));
#67335=CARTESIAN_POINT('Ctrl Pts',(0.508005813882541,0.65708698396994,-6.56654153199149));
#67336=CARTESIAN_POINT('Ctrl Pts',(0.00468281360600204,0.783025992947568,
-6.54535940066562));
#67337=CARTESIAN_POINT('Ctrl Pts',(-0.497725690303919,0.664062393222252,
-6.52417726933977));
#67338=CARTESIAN_POINT('Ctrl Pts',(-0.888204658056055,0.0725067595126697,
-6.49769960518244));
#67339=CARTESIAN_POINT('Ctrl Pts',(-0.539556042745298,-0.708423110273319,
-6.46592640819366));
#67340=CARTESIAN_POINT('Ctrl Pts',(0.159626968110726,-0.814403639841095,
-6.43944874403633));
#67341=CARTESIAN_POINT('Ctrl Pts',(0.586356716261186,-0.520166247602953,
-6.41826661271048));
#67342=CARTESIAN_POINT('Ctrl Pts',(0.765367506278367,-0.176732126196868,
-6.40238001421609));
#67343=CARTESIAN_POINT('Ctrl Pts',(0.755272358384135,0.209644083564372,
-6.38649341572169));
#67344=CARTESIAN_POINT('Ctrl Pts',(0.50042423474264,0.662620189055778,-6.36531128439583));
#67345=CARTESIAN_POINT('Ctrl Pts',(-0.0381697288917987,0.82968427820954,
-6.34412915306998));
#67346=CARTESIAN_POINT('Ctrl Pts',(-0.503324291271846,0.599846863125267,
-6.32294702174411));
#67347=CARTESIAN_POINT('Ctrl Pts',(-0.80924501584584,0.183937831155953,
-6.30176489041826));
#67348=CARTESIAN_POINT('Ctrl Pts',(-0.723917441136396,-0.519716397702539,
-6.27528722626094));
#67349=CARTESIAN_POINT('Ctrl Pts',(0.0473522548033906,-0.88923835783592,
-6.24351402927214));
#67350=CARTESIAN_POINT('Ctrl Pts',(0.648876614824445,-0.51739292476347,
-6.21703636511482));
#67351=CARTESIAN_POINT('Ctrl Pts',(0.783640719169264,-0.0168908517885347,
-6.19585423378896));
#67352=CARTESIAN_POINT('Ctrl Pts',(0.697776849956767,0.360768407837624,
-6.17996763529457));
#67353=CARTESIAN_POINT('Ctrl Pts',(0.439924199101702,0.648698474965856,
-6.16408103680018));
#67354=CARTESIAN_POINT('Ctrl Pts',(-0.0474756093028199,0.829034275270768,
-6.14289890547431));
#67355=CARTESIAN_POINT('Ctrl Pts',(-0.566295088878221,0.607590983903843,
-6.12171677414848));
#67356=CARTESIAN_POINT('Ctrl Pts',(-0.771819506095907,0.131460151558091,
-6.10053464282259));
#67357=CARTESIAN_POINT('Ctrl Pts',(-0.73615650740269,-0.383882627307947,
-6.07935251149675));
#67358=CARTESIAN_POINT('Ctrl Pts',(-0.214722507390818,-0.864304610211316,
-6.05287484733942));
#67359=CARTESIAN_POINT('Ctrl Pts',(0.610710452266349,-0.647893193725871,
-6.02110165035064));
#67360=CARTESIAN_POINT('Ctrl Pts',(0.87514783710282,0.161911029797875,-5.98932845336184));
#67361=CARTESIAN_POINT('Ctrl Pts',(0.338210898045152,0.823232838751861,
-5.95755525637307));
#67362=CARTESIAN_POINT('Ctrl Pts',(-0.508641841679914,0.730764205387854,
-5.92578205938427));
#67363=CARTESIAN_POINT('Ctrl Pts',(-0.889979875388079,-0.0326195618755111,
-5.89400886239549));
#67364=CARTESIAN_POINT('Ctrl Pts',(-0.526901538696912,-0.641612845459792,
-5.86753119823816));
#67365=CARTESIAN_POINT('Ctrl Pts',(-0.0298714672499406,-0.782364887301405,
-5.84634906691231));
#67366=CARTESIAN_POINT('Ctrl Pts',(0.47832166267773,-0.679017907291142,
-5.82516693558643));
#67367=CARTESIAN_POINT('Ctrl Pts',(0.801607061401948,-0.216743816896674,
-5.8039848042606));
#67368=CARTESIAN_POINT('Ctrl Pts',(0.725226253928277,0.297304377686334,
-5.78280267293472));
#67369=CARTESIAN_POINT('Ctrl Pts',(0.496397105934749,0.608799055229958,
-5.76691607444034));
#67370=CARTESIAN_POINT('Ctrl Pts',(0.144426057203333,0.770401967556523,
-5.75102947594594));
#67371=CARTESIAN_POINT('Ctrl Pts',(-0.373084797124373,0.741312372766026,
-5.72984734462008));
#67372=CARTESIAN_POINT('Ctrl Pts',(-0.860552864376412,0.228988778535637,
-5.70336968046277));
#67373=CARTESIAN_POINT('Ctrl Pts',(-0.657325329301909,-0.601734997387143,
-5.67159648347396));
#67374=CARTESIAN_POINT('Ctrl Pts',(0.0138002762959166,-0.829771157474066,
-5.64511881931665));
#67375=CARTESIAN_POINT('Ctrl Pts',(0.483676613599726,-0.615799102664358,
-5.62393668799079));
#67376=CARTESIAN_POINT('Ctrl Pts',(0.804154597478065,-0.20776985601056,
-5.60275455666493));
#67377=CARTESIAN_POINT('Ctrl Pts',(0.751277615728742,0.353655020842358,
-5.58157242533908));
#67378=CARTESIAN_POINT('Ctrl Pts',(0.360304271057673,0.69610904991264,-5.56039029401322));
#67379=CARTESIAN_POINT('Ctrl Pts',(-0.0157604757935807,0.785349139873212,
-5.54450369551882));
#67380=CARTESIAN_POINT('Ctrl Pts',(-0.388640335473441,0.680695095834419,
-5.52861709702443));
#67381=CARTESIAN_POINT('Ctrl Pts',(-0.764252910898822,0.323498911462347,
-5.50743496569857));
#67382=CARTESIAN_POINT('Ctrl Pts',(-0.804141491407507,-0.382544753237058,
-5.48095730154125));
#67383=CARTESIAN_POINT('Ctrl Pts',(-0.111472970044356,-0.884159782910866,
-5.44918410455246));
#67384=CARTESIAN_POINT('Ctrl Pts',(0.547672930190298,-0.623509491842228,
-5.42270644039513));
#67385=CARTESIAN_POINT('Ctrl Pts',(0.767292864059844,-0.156247544421139,
-5.40152430906929));
#67386=CARTESIAN_POINT('Ctrl Pts',(0.74741961163729,0.362211451477082,-5.38034217774341));
#67387=CARTESIAN_POINT('Ctrl Pts',(0.34367744228227,0.755893837136436,-5.35916004641757));
#67388=CARTESIAN_POINT('Ctrl Pts',(-0.176007263809187,0.76381183657692,
-5.3379779150917));
#67389=CARTESIAN_POINT('Ctrl Pts',(-0.520410163705834,0.588383282992382,
-5.32209131659731));
#67390=CARTESIAN_POINT('Ctrl Pts',(-0.736867711719661,0.267232304854123,
-5.30620471810292));
#67391=CARTESIAN_POINT('Ctrl Pts',(-0.791924355942771,-0.248173086389637,
-5.28502258677705));
#67392=CARTESIAN_POINT('Ctrl Pts',(-0.365267985880006,-0.812135033397483,
-5.25854492261974));
#67393=CARTESIAN_POINT('Ctrl Pts',(0.487399303105791,-0.74606076805389,
-5.22677172563095));
#67394=CARTESIAN_POINT('Ctrl Pts',(0.821061658291666,-0.120695808334838,
-5.20029406147362));
#67395=CARTESIAN_POINT('Ctrl Pts',(0.685970800776325,0.377618450392495,
-5.17911193014777));
#67396=CARTESIAN_POINT('Ctrl Pts',(0.335197903320081,0.759918139134054,
-5.1579297988219));
#67397=CARTESIAN_POINT('Ctrl Pts',(-0.227381916708832,0.798615765401183,
-5.13674766749606));
#67398=CARTESIAN_POINT('Ctrl Pts',(-0.628606563135292,0.468231638735957,
-5.11556553617019));
#67399=CARTESIAN_POINT('Ctrl Pts',(-0.777543191380457,0.111571554309256,
-5.0996789376758));
#67400=CARTESIAN_POINT('Ctrl Pts',(-0.734627282762826,-0.273331089931772,
-5.0837923391814));
#67401=CARTESIAN_POINT('Ctrl Pts',(-0.442942022564239,-0.701809397937808,
-5.06261020785555));
#67402=CARTESIAN_POINT('Ctrl Pts',(0.24733367727714,-0.855458979751414,
-5.03613254369822));
#67403=CARTESIAN_POINT('Ctrl Pts',(0.854455518574205,-0.253121546055969,
-5.00435934670944));
#67404=CARTESIAN_POINT('Ctrl Pts',(0.703938379568512,0.439523017191998,
-4.97788168255211));
#67405=CARTESIAN_POINT('Ctrl Pts',(0.278388425828125,0.731882174913778,
-4.95669955122626));
#67406=CARTESIAN_POINT('Ctrl Pts',(-0.236450085029051,0.796193801701192,
-4.93551741990039));
#67407=CARTESIAN_POINT('Ctrl Pts',(-0.690294259443345,0.461501367465407,
-4.91433528857454));
#67408=CARTESIAN_POINT('Ctrl Pts',(-0.782229035346391,-0.0500481267487367,
-4.89315315724868));
#67409=CARTESIAN_POINT('Ctrl Pts',(-0.664862395795767,-0.418305654814762,
-4.87726655875428));
#67410=CARTESIAN_POINT('Ctrl Pts',(-0.382984625029711,-0.683893198016694,
-4.8613799602599));
#67411=CARTESIAN_POINT('Ctrl Pts',(0.11671167241904,-0.821652269459763,
-4.84019782893403));
#67412=CARTESIAN_POINT('Ctrl Pts',(0.742298900655215,-0.491910922869968,
-4.81372016477672));
#67413=CARTESIAN_POINT('Ctrl Pts',(0.815116995369976,0.36020693241341,-4.78194696778791));
#67414=CARTESIAN_POINT('Ctrl Pts',(0.252009078067586,0.790696622885568,
-4.75546930363061));
#67415=CARTESIAN_POINT('Ctrl Pts',(-0.261600597687866,0.738049294343494,
-4.73428717230474));
#67416=CARTESIAN_POINT('Ctrl Pts',(-0.695638069988528,0.453785068242976,
-4.71310504097889));
#67417=CARTESIAN_POINT('Ctrl Pts',(-0.824889973540065,-0.0951115573731555,
-4.69192290965302));
#67418=CARTESIAN_POINT('Ctrl Pts',(-0.563809010906991,-0.544524083902708,
-4.67074077832718));
#67419=CARTESIAN_POINT('Ctrl Pts',(-0.235960833039409,-0.749229011360774,
-4.65485417983276));
#67420=CARTESIAN_POINT('Ctrl Pts',(0.150812554763246,-0.769183139849302,
-4.63896758133839));
#67421=CARTESIAN_POINT('Ctrl Pts',(0.620855152320868,-0.550702230087972,
-4.61778545001251));
#67422=CARTESIAN_POINT('Ctrl Pts',(0.884213132850611,0.105599004006847,
-4.5913077858552));
#67423=CARTESIAN_POINT('Ctrl Pts',(0.388093857664531,0.802214377796061,
-4.5595345888664));
#67424=CARTESIAN_POINT('Ctrl Pts',(-0.319780369690156,0.765800391767949,
-4.53305692470909));
#67425=CARTESIAN_POINT('Ctrl Pts',(-0.677167572045297,0.393186613406222,
-4.51187479338323));
#67426=CARTESIAN_POINT('Ctrl Pts',(-0.823967811864189,-0.104452178480815,
-4.49069266205737));
#67427=CARTESIAN_POINT('Ctrl Pts',(-0.567152865214582,-0.606487678581986,
-4.46951053073151));
#67428=CARTESIAN_POINT('Ctrl Pts',(-0.077231065227596,-0.780014385312101,
-4.44832839940566));
#67429=CARTESIAN_POINT('Ctrl Pts',(0.305168035875328,-0.723805288785105,
-4.43244180091126));
#67430=CARTESIAN_POINT('Ctrl Pts',(0.612880513490481,-0.488635452547494,
-4.41655520241687));
#67431=CARTESIAN_POINT('Ctrl Pts',(0.829708518342342,-0.0178280951699618,
-4.395373071091));
#67432=CARTESIAN_POINT('Ctrl Pts',(0.605579358449078,0.652884105008795,
-4.36889540693369));
#67433=CARTESIAN_POINT('Ctrl Pts',(-0.223513846984806,0.862673930581949,
-4.33712220994489));
#67434=CARTESIAN_POINT('Ctrl Pts',(-0.739476400119356,0.376675428635363,
-4.31064454578758));
#67435=CARTESIAN_POINT('Ctrl Pts',(-0.770661211393977,-0.138682842645893,
-4.28946241446172));
#67436=CARTESIAN_POINT('Ctrl Pts',(-0.560403328348306,-0.613010050614006,
-4.26828028313586));
#67437=CARTESIAN_POINT('Ctrl Pts',(-0.0396674371228205,-0.829407120312446,
-4.24709815181));
#67438=CARTESIAN_POINT('Ctrl Pts',(0.446079393600652,-0.644515518304158,
-4.22591602048414));
#67439=CARTESIAN_POINT('Ctrl Pts',(0.701153381813063,-0.354126476510017,
-4.21002942198975));
#67440=CARTESIAN_POINT('Ctrl Pts',(0.783451243037709,0.0243162309027824,
-4.19414282349535));
#67441=CARTESIAN_POINT('Ctrl Pts',(0.643937273529952,0.523525409264962,
-4.1729606921695));
#67442=CARTESIAN_POINT('Ctrl Pts',(0.0389209183077788,0.889645533946421,
-4.14648302801217));
#67443=CARTESIAN_POINT('Ctrl Pts',(-0.728814260660947,0.512829916987002,
-4.11470983102339));
#67444=CARTESIAN_POINT('Ctrl Pts',(-0.807463872462469,-0.191603286869062,
-4.08823216686606));
#67445=CARTESIAN_POINT('Ctrl Pts',(-0.497614223633389,-0.604592191505413,
-4.06705003554021));
#67446=CARTESIAN_POINT('Ctrl Pts',(-0.030300728770561,-0.830009083331993,
-4.04586790421435));
#67447=CARTESIAN_POINT('Ctrl Pts',(0.506684552648503,-0.657845301647932,
-4.02468577288849));
#67448=CARTESIAN_POINT('Ctrl Pts',(0.757226299555704,-0.202473232777027,
-4.00350364156263));
#67449=CARTESIAN_POINT('Ctrl Pts',(0.76365730106179,0.18398139234257,-3.98761704306824));
#67450=CARTESIAN_POINT('Ctrl Pts',(0.581398171507507,0.52570266831202,-3.97173044457384));
#67451=CARTESIAN_POINT('Ctrl Pts',(0.1518976340338,0.815880613302076,-3.95054831324798));
#67452=CARTESIAN_POINT('Ctrl Pts',(-0.546249025453097,0.703275206547391,
-3.92407064909066));
#67453=CARTESIAN_POINT('Ctrl Pts',(-0.8874772256122,-0.0809254244309511,
-3.89229745210188));
#67454=CARTESIAN_POINT('Ctrl Pts',(-0.491406696126427,-0.668751959902339,
-3.86581978794455));
#67455=CARTESIAN_POINT('Ctrl Pts',(0.0121072287199249,-0.782946389355173,
-3.8446376566187));
#67456=CARTESIAN_POINT('Ctrl Pts',(0.514213453953207,-0.652240550986492,
-3.82345552529283));
#67457=CARTESIAN_POINT('Ctrl Pts',(0.812048062749978,-0.173400174673731,
-3.80227339396698));
#67458=CARTESIAN_POINT('Ctrl Pts',(0.708222469234925,0.335869041146677,
-3.78109126264112));
#67459=CARTESIAN_POINT('Ctrl Pts',(0.462951781598219,0.634584331754523,
-3.76520466414672));
#67460=CARTESIAN_POINT('Ctrl Pts',(0.102821450890194,0.777055260930318,
-3.74931806565233));
#67461=CARTESIAN_POINT('Ctrl Pts',(-0.412387310159186,0.72018801212385,
-3.72813593432647));
#67462=CARTESIAN_POINT('Ctrl Pts',(-0.871612899585501,0.182414273643501,
-3.70165827016915));
#67463=CARTESIAN_POINT('Ctrl Pts',(-0.624039721496535,-0.636191147607529,
-3.66988507318036));
#67464=CARTESIAN_POINT('Ctrl Pts',(0.0583725307045223,-0.827829917634214,
-3.64340740902304));
#67465=CARTESIAN_POINT('Ctrl Pts',(0.516070260716903,-0.588916903811706,
-3.62222527769718));
#67466=CARTESIAN_POINT('Ctrl Pts',(0.814158273260994,-0.164254432690011,
-3.60104314637132));
#67467=CARTESIAN_POINT('Ctrl Pts',(0.731186599072323,0.393517260269395,
-3.57986101504547));
#67468=CARTESIAN_POINT('Ctrl Pts',(0.322375024407198,0.714465830091588,
-3.5586788837196));
#67469=CARTESIAN_POINT('Ctrl Pts',(-0.057942108370507,0.78336730737941,
-3.54279228522521));
#67470=CARTESIAN_POINT('Ctrl Pts',(-0.424659040323523,0.658826099038399,
-3.52690568673082));
#67471=CARTESIAN_POINT('Ctrl Pts',(-0.780533275196529,0.281960764465941,
-3.50572355540496));
#67472=CARTESIAN_POINT('Ctrl Pts',(-0.782421669494201,-0.425206238264019,
-3.47924589124764));
#67473=CARTESIAN_POINT('Ctrl Pts',(-0.0637974639085965,-0.888872675864485,
-3.44747269425885));
#67474=CARTESIAN_POINT('Ctrl Pts',(0.580388709786245,-0.593176761533836,
-3.42099503010153));
#67475=CARTESIAN_POINT('Ctrl Pts',(0.774580797896507,-0.114787721998427,
-3.39981289877567));
#67476=CARTESIAN_POINT('Ctrl Pts',(0.726874463911719,0.401854110705244,
-3.37863076744981));
#67477=CARTESIAN_POINT('Ctrl Pts',(0.302559358947867,0.773270658376436,
-3.35744863612395));
#67478=CARTESIAN_POINT('Ctrl Pts',(-0.21679990318929,0.753249547432401,
-3.3362665047981));
#67479=CARTESIAN_POINT('Ctrl Pts',(-0.551277667357786,0.559566403267617,
-3.3203799063037));
#67480=CARTESIAN_POINT('Ctrl Pts',(-0.750163892116854,0.227247143583241,
-3.30449330780931));
#67481=CARTESIAN_POINT('Ctrl Pts',(-0.777443278256896,-0.290372201631635,
-3.28331117648345));
#67482=CARTESIAN_POINT('Ctrl Pts',(-0.321096322413234,-0.830590853360081,
-3.25683351232612));
#67483=CARTESIAN_POINT('Ctrl Pts',(0.526788039301812,-0.718790033283858,
-3.22506031533735));
#67484=CARTESIAN_POINT('Ctrl Pts',(0.826361358316619,-0.0763978425888647,
-3.19858265118));
#67485=CARTESIAN_POINT('Ctrl Pts',(0.664686480633999,0.413936608738543,
-3.17740051985416));
#67486=CARTESIAN_POINT('Ctrl Pts',(0.293875808800309,0.77683345807168,-3.15621838852829));
#67487=CARTESIAN_POINT('Ctrl Pts',(-0.269970669492542,0.785242328460858,
-3.13503625720245));
#67488=CARTESIAN_POINT('Ctrl Pts',(-0.652860814798813,0.433773944849426,
-3.11385412587658));
#67489=CARTESIAN_POINT('Ctrl Pts',(-0.782415442264087,0.0696254400343804,
-3.09796752738219));
#67490=CARTESIAN_POINT('Ctrl Pts',(-0.718877018329645,-0.312414727277906,
-3.08208092888779));
#67491=CARTESIAN_POINT('Ctrl Pts',(-0.404586978639708,-0.724598815278104,
-3.06089879756194));
#67492=CARTESIAN_POINT('Ctrl Pts',(0.292948333281876,-0.840931202881724,
-3.03442113340461));
#67493=CARTESIAN_POINT('Ctrl Pts',(0.866823475343164,-0.206837648636938,
-3.00264793641582));
#67494=CARTESIAN_POINT('Ctrl Pts',(0.679301366799664,0.476717293513901,
-2.9761702722585));
#67495=CARTESIAN_POINT('Ctrl Pts',(0.238655064681991,0.745785085459083,
-2.95498814093265));
#67496=CARTESIAN_POINT('Ctrl Pts',(-0.27889557868341,0.782336544441392,
-2.93380600960678));
#67497=CARTESIAN_POINT('Ctrl Pts',(-0.714097688888377,0.423738324343162,
-2.91262387828093));
#67498=CARTESIAN_POINT('Ctrl Pts',(-0.778409131595645,-0.0920125131626953,
-2.89144174695507));
#67499=CARTESIAN_POINT('Ctrl Pts',(-0.641422061965753,-0.45343066131097,
-2.87555514846067));
#67500=CARTESIAN_POINT('Ctrl Pts',(-0.345679030790674,-0.703486415628807,
-2.85966854996628));
#67501=CARTESIAN_POINT('Ctrl Pts',(0.160698319191389,-0.814192923450146,
-2.83848641864043));
#67502=CARTESIAN_POINT('Ctrl Pts',(0.767661380996447,-0.451309226672089,
-2.8120087544831));
#67503=CARTESIAN_POINT('Ctrl Pts',(0.794581745299286,0.403490520752094,
-2.78023555749431));
#67504=CARTESIAN_POINT('Ctrl Pts',(0.209153168296713,0.803096928809075,
-2.75375789333699));
#67505=CARTESIAN_POINT('Ctrl Pts',(-0.300885083483398,0.722924477472416,
-2.73257576201113));
#67506=CARTESIAN_POINT('Ctrl Pts',(-0.719019106384883,0.415746000860054,
-2.71139363068527));
#67507=CARTESIAN_POINT('Ctrl Pts',(-0.818586731398151,-0.139303409763623,
-2.69021149935941));
#67508=CARTESIAN_POINT('Ctrl Pts',(-0.533731768126874,-0.574036129892679,
-2.66902936803356));
#67509=CARTESIAN_POINT('Ctrl Pts',(-0.195356567801208,-0.76082681183711,
-2.65314276953916));
#67510=CARTESIAN_POINT('Ctrl Pts',(0.191930252984854,-0.759967043556375,
-2.63725617104477));
#67511=CARTESIAN_POINT('Ctrl Pts',(0.649552544819839,-0.516541922698741,
-2.61607403971891));
#67512=CARTESIAN_POINT('Ctrl Pts',(0.877260576037617,0.152963707077457,
-2.58959637556159));
#67513=CARTESIAN_POINT('Ctrl Pts',(0.344422342865012,0.82191118743757,-2.5578231785728));
#67514=CARTESIAN_POINT('Ctrl Pts',(-0.360472118628379,0.747508914035598,
-2.53134551441547));
#67515=CARTESIAN_POINT('Ctrl Pts',(-0.69731875949566,0.356227709824785,
-2.51016338308962));
#67516=CARTESIAN_POINT('Ctrl Pts',(-0.817163940645753,-0.148580976864318,
-2.48898125176376));
#67517=CARTESIAN_POINT('Ctrl Pts',(-0.533740889221978,-0.636089883558451,
-2.4677991204379));
#67518=CARTESIAN_POINT('Ctrl Pts',(-0.0352017725222705,-0.783037619748434,
-2.44661698911204));
#67519=CARTESIAN_POINT('Ctrl Pts',(0.343624098183447,-0.706359756314665,
-2.43073039061765));
#67520=CARTESIAN_POINT('Ctrl Pts',(0.638253983199123,-0.454993387021286,
-2.41484379212325));
#67521=CARTESIAN_POINT('Ctrl Pts',(0.829467649601628,0.0267859039717638,
-2.3936616607974));
#67522=CARTESIAN_POINT('Ctrl Pts',(0.569618528201855,0.68448429220975,-2.36718399664007));
#67523=CARTESIAN_POINT('Ctrl Pts',(-0.269550651946428,0.849415797083451,
-2.33541079965129));
#67524=CARTESIAN_POINT('Ctrl Pts',(-0.758650245032131,0.336391930021827,
-2.30893313549396));
#67525=CARTESIAN_POINT('Ctrl Pts',(-0.762094825624762,-0.179897499558888,
-2.28775100416811));
#67526=CARTESIAN_POINT('Ctrl Pts',(-0.526650595635342,-0.642240112959774,
-2.26656887284225));
#67527=CARTESIAN_POINT('Ctrl Pts',(0.00496192325041732,-0.830340325475366,
-2.24538674151639));
#67528=CARTESIAN_POINT('Ctrl Pts',(0.480070832655676,-0.619612035360264,
-2.22420461019054));
#67529=CARTESIAN_POINT('Ctrl Pts',(0.719170831623089,-0.315935026763165,
-2.20831801169613));
#67530=CARTESIAN_POINT('Ctrl Pts',(0.781012395997661,0.066383481383875,
-2.19243141320175));
#67531=CARTESIAN_POINT('Ctrl Pts',(0.614872705146752,0.55737386272838,-2.17124928187588));
#67532=CARTESIAN_POINT('Ctrl Pts',(-0.00894455400451892,0.890451575834638,
-2.14477161771857));
#67533=CARTESIAN_POINT('Ctrl Pts',(-0.75532040577284,0.472922652156577,
-2.11299842072978));
#67534=CARTESIAN_POINT('Ctrl Pts',(-0.796000380537386,-0.234719234523823,
-2.08652075657245));
#67535=CARTESIAN_POINT('Ctrl Pts',(-0.46440459505787,-0.630460153919906,
-2.06533862524659));
#67536=CARTESIAN_POINT('Ctrl Pts',(0.01434744581186,-0.830438055110873,
-2.04415649392074));
#67537=CARTESIAN_POINT('Ctrl Pts',(0.541304753887728,-0.629665657481347,
-2.02297436259488));
#67538=CARTESIAN_POINT('Ctrl Pts',(0.767012932214679,-0.161487586350912,
-2.00179223126902));
#67539=CARTESIAN_POINT('Ctrl Pts',(0.75266670831207,0.224754204392204,-1.98590563277462));
#67540=CARTESIAN_POINT('Ctrl Pts',(0.55230696816604,0.556187146757173,-1.97001903428023));
#67541=CARTESIAN_POINT('Ctrl Pts',(0.107833008568935,0.822864574915098,
-1.94883690295438));
#67542=CARTESIAN_POINT('Ctrl Pts',(-0.583253442038985,0.672903734796001,
-1.92235923879705));
#67543=CARTESIAN_POINT('Ctrl Pts',(-0.881845901412668,-0.128501192451031,
-1.89058604180827));
#67544=CARTESIAN_POINT('Ctrl Pts',(-0.454758114676497,-0.694193619969962,
-1.86410837765094));
#67545=CARTESIAN_POINT('Ctrl Pts',(0.0541649907798706,-0.781164379222065,
-1.84292624632508));
#67546=CARTESIAN_POINT('Ctrl Pts',(0.548521578507037,-0.623664405341359,
-1.82174411499922));
#67547=CARTESIAN_POINT('Ctrl Pts',(0.820193101266005,-0.129510437527382,
-1.80056198367337));
#67548=CARTESIAN_POINT('Ctrl Pts',(0.689149593251153,0.373443324818871,
-1.77937985234751));
#67549=CARTESIAN_POINT('Ctrl Pts',(0.428180474068072,0.658546207809391,
-1.76349325385311));
#67550=CARTESIAN_POINT('Ctrl Pts',(0.0609142018835925,0.781457989473221,
-1.74760665535872));
#67551=CARTESIAN_POINT('Ctrl Pts',(-0.45049404748608,0.696985781466766,
-1.72642452403286));
#67552=CARTESIAN_POINT('Ctrl Pts',(-0.880156280245255,0.135310518059632,
-1.69994685987554));
#67553=CARTESIAN_POINT('Ctrl Pts',(-0.588949289207153,-0.668807509708173,
-1.66817366288675));
#67554=CARTESIAN_POINT('Ctrl Pts',(0.102775463205937,-0.823496769291736,
-1.64169599872943));
#67555=CARTESIAN_POINT('Ctrl Pts',(0.546972712137699,-0.56033247788104,
-1.62051386740357));
#67556=CARTESIAN_POINT('Ctrl Pts',(0.821808773600565,-0.120264509356574,
-1.59933173607771));
#67557=CARTESIAN_POINT('Ctrl Pts',(0.708982544944508,0.432242325272397,
-1.57814960475185));
#67558=CARTESIAN_POINT('Ctrl Pts',(0.283514049915959,0.730757731556947,
-1.556967473426));
#67559=CARTESIAN_POINT('Ctrl Pts',(-0.0999562581644404,0.779121539072725,
-1.5410808749316));
#67560=CARTESIAN_POINT('Ctrl Pts',(-0.459450477644474,0.63505305911783,
-1.52519427643721));
#67561=CARTESIAN_POINT('Ctrl Pts',(-0.79455786019474,0.239607748601739,
-1.50401214511135));
#67562=CARTESIAN_POINT('Ctrl Pts',(-0.758440625467195,-0.466638866355624,
-1.47753448095403));
#67563=CARTESIAN_POINT('Ctrl Pts',(-0.0159375776428949,-0.891016691155971,
-1.44576128396524));
#67564=CARTESIAN_POINT('Ctrl Pts',(0.611427143079269,-0.561129729721242,
-1.41928361980792));
#67565=CARTESIAN_POINT('Ctrl Pts',(0.779630165187704,-0.0729961582617228,
-1.39810148848206));
#67566=CARTESIAN_POINT('Ctrl Pts',(0.704228621556494,0.440335396213263,
-1.3769193571562));
#67567=CARTESIAN_POINT('Ctrl Pts',(0.260566868148073,0.788412699045606,
-1.35573722583034));
#67568=CARTESIAN_POINT('Ctrl Pts',(-0.256965982948583,0.740510339115715,
-1.33455509450448));
#67569=CARTESIAN_POINT('Ctrl Pts',(-0.580551958086807,0.529132355989381,
-1.31866849601009));
#67570=CARTESIAN_POINT('Ctrl Pts',(-0.761292071137348,0.186605229632119,
-1.3027818975157));
#67571=CARTESIAN_POINT('Ctrl Pts',(-0.76071536070743,-0.331732130447139,
-1.28159976618984));
#67572=CARTESIAN_POINT('Ctrl Pts',(-0.275996678705884,-0.846646235033293,
-1.25512210203252));
#67573=CARTESIAN_POINT('Ctrl Pts',(0.564654338578688,-0.689441968713772,
-1.22334890504373));
#67574=CARTESIAN_POINT('Ctrl Pts',(0.829272843434691,-0.0318790842538621,
-1.19687124088641));
#67575=CARTESIAN_POINT('Ctrl Pts',(0.641481191968628,0.44905847496967,-1.17568910956055));
#67576=CARTESIAN_POINT('Ctrl Pts',(0.251704402317549,0.791503699569123,
-1.15450697823469));
#67577=CARTESIAN_POINT('Ctrl Pts',(-0.311779197051007,0.769599512135441,
-1.13332484690883));
#67578=CARTESIAN_POINT('Ctrl Pts',(-0.675228274549961,0.398062628211048,
-1.11214271558297));
#67579=CARTESIAN_POINT('Ctrl Pts',(-0.785026483567616,0.0274781056615818,
-1.09625611708858));
#67580=CARTESIAN_POINT('Ctrl Pts',(-0.70104917271287,-0.350595474501956,
-1.08036951859419));
#67581=CARTESIAN_POINT('Ctrl Pts',(-0.365062663375868,-0.745294115229794,
-1.05918738726832));
#67582=CARTESIAN_POINT('Ctrl Pts',(0.337716357763391,-0.823973103718647,
-1.032709723111));
#67583=CARTESIAN_POINT('Ctrl Pts',(0.876686280193239,-0.15995598275971,
-1.00093652612222));
#67584=CARTESIAN_POINT('Ctrl Pts',(0.652701147944472,0.512533839217553,
-0.974458861964892));
#67585=CARTESIAN_POINT('Ctrl Pts',(0.198231981567963,0.75753264951101,-0.953276730639035));
#67586=CARTESIAN_POINT('Ctrl Pts',(-0.320535053795434,0.766218305619351,
-0.932094599313175));
#67587=CARTESIAN_POINT('Ctrl Pts',(-0.735837349588571,0.384750661783734,
-0.910912467987319));
#67588=CARTESIAN_POINT('Ctrl Pts',(-0.772339596651168,-0.133710980008637,
-0.889730336661458));
#67589=CARTESIAN_POINT('Ctrl Pts',(-0.616127994641744,-0.487245236418133,
-0.873843738167066));
#67590=CARTESIAN_POINT('Ctrl Pts',(-0.307374411361996,-0.721046531467661,
-0.85795713967267));
#67591=CARTESIAN_POINT('Ctrl Pts',(0.20422054187608,-0.80438052976603,-0.836775008346816));
#67592=CARTESIAN_POINT('Ctrl Pts',(0.790805291538328,-0.409403230105263,
-0.810297344189487));
#67593=CARTESIAN_POINT('Ctrl Pts',(0.771750124586875,0.445608006548333,
-0.778524147200705));
#67594=CARTESIAN_POINT('Ctrl Pts',(0.165692798123157,0.813176254903035,
-0.752046483043378));
#67595=CARTESIAN_POINT('Ctrl Pts',(-0.33930000024461,0.705710382095269,
-0.730864351717522));
#67596=CARTESIAN_POINT('Ctrl Pts',(-0.740322150981868,0.376505412191275,
-0.709682220391663));
#67597=CARTESIAN_POINT('Ctrl Pts',(-0.809917743263348,-0.183092670227531,
-0.688500089065804));
#67598=CARTESIAN_POINT('Ctrl Pts',(-0.502112020847565,-0.601889190124352,
-0.667317957739947));
#67599=CARTESIAN_POINT('Ctrl Pts',(-0.154187714727574,-0.770225794886024,
-0.651431359245553));
#67600=CARTESIAN_POINT('Ctrl Pts',(0.232493265444015,-0.748554614000191,
-0.635544760751159));
#67601=CARTESIAN_POINT('Ctrl Pts',(0.676372706924209,-0.480888790873769,
-0.614362629425302));
#67602=CARTESIAN_POINT('Ctrl Pts',(0.86777270267367,0.199886341100763,-0.587884965267977));
#67603=CARTESIAN_POINT('Ctrl Pts',(0.299755436540123,0.839232640318567,
-0.556111768279191));
#67604=CARTESIAN_POINT('Ctrl Pts',(-0.400122092807645,0.72705711293915,
-0.529634104121868));
#67605=CARTESIAN_POINT('Ctrl Pts',(-0.715454665930561,0.318239288246659,
-0.508451972796009));
#67606=CARTESIAN_POINT('Ctrl Pts',(-0.807998445695184,-0.192280353386799,
-0.487269841470152));
#67607=CARTESIAN_POINT('Ctrl Pts',(-0.498786361378514,-0.663853800491803,
-0.466087710144292));
#67608=CARTESIAN_POINT('Ctrl Pts',(0.00692922874373258,-0.783797802920765,
-0.444905578818435));
#67609=CARTESIAN_POINT('Ctrl Pts',(0.381087127953349,-0.686872908670706,
-0.429018980324039));
#67610=CARTESIAN_POINT('Ctrl Pts',(0.661782777111213,-0.420036208409248,
-0.413132381829648));
#67611=CARTESIAN_POINT('Ctrl Pts',(0.826829800764357,0.0713221335761503,
-0.391950250503787));
#67612=CARTESIAN_POINT('Ctrl Pts',(0.532011040561915,0.714107033573504,
-0.365472586346466));
#67613=CARTESIAN_POINT('Ctrl Pts',(-0.314807679105772,0.833701529443594,
-0.333699389357678));
#67614=CARTESIAN_POINT('Ctrl Pts',(-0.775632848136392,0.295138411630498,
-0.307221725200355));
#67615=CARTESIAN_POINT('Ctrl Pts',(-0.751324246115917,-0.220595129012272,
-0.286039593874496));
#67616=CARTESIAN_POINT('Ctrl Pts',(-0.491380230422849,-0.669606653773286,
-0.264857462548639));
#67617=CARTESIAN_POINT('Ctrl Pts',(0.0495859047765307,-0.828888911462718,
-0.243675331222779));
#67618=CARTESIAN_POINT('Ctrl Pts',(0.512663775722113,-0.592899197626148,
-0.222493199896921));
#67619=CARTESIAN_POINT('Ctrl Pts',(0.735132893747708,-0.27686932786066,
-0.206606601402529));
#67620=CARTESIAN_POINT('Ctrl Pts',(0.776274364779559,0.108329678724445,
-0.190720002908133));
#67621=CARTESIAN_POINT('Ctrl Pts',(0.584121944633851,0.58945851373242,-0.169537871582277));
#67622=CARTESIAN_POINT('Ctrl Pts',(-0.0569720689210273,0.889000674187564,
-0.143060207424953));
#67623=CARTESIAN_POINT('Ctrl Pts',(-0.779315258188735,0.431095499374008,
-0.111287010436167));
#67624=CARTESIAN_POINT('Ctrl Pts',(-0.782788362817514,-0.276227349621032,
-0.0848093462788417));
#67625=CARTESIAN_POINT('Ctrl Pts',(-0.429109244619801,-0.655756861746561,
-0.0636272149529857));
#67626=CARTESIAN_POINT('Ctrl Pts',(-0.0646184054315698,-0.782693153117636,
-0.0477406164585894));
#67627=CARTESIAN_POINT('Ctrl Pts',(0.318892419761328,-0.717280333622648,
-0.0318540179641984));
#67628=CARTESIAN_POINT('Ctrl Pts',(0.521380142127114,-0.557506295451278,
-0.021262952301267));
#67629=CARTESIAN_POINT('Ctrl Pts',(0.597589667152271,-0.458088845993819,
-0.0159674194698027));
#67630=CARTESIAN_POINT('Ctrl Pts',(-0.34206796250955,0.713322310757602,
-11.9089));
#67631=CARTESIAN_POINT('Ctrl Pts',(-0.46073916563555,0.656414492160488,
-11.9036044671685));
#67632=CARTESIAN_POINT('Ctrl Pts',(-0.668722237093865,0.482686815406386,
-11.8930134015056));
#67633=CARTESIAN_POINT('Ctrl Pts',(-0.818743490259774,0.102460369625847,
-11.8771268030112));
#67634=CARTESIAN_POINT('Ctrl Pts',(-0.766878588870734,-0.299717504486475,
-11.8612402045168));
#67635=CARTESIAN_POINT('Ctrl Pts',(-0.452953262747085,-0.745287473216968,
-11.840058073191));
#67636=CARTESIAN_POINT('Ctrl Pts',(0.275096172417156,-0.894355306323675,
-11.8135804090336));
#67637=CARTESIAN_POINT('Ctrl Pts',(0.901814470278374,-0.250425930665646,
-11.7818072120449));
#67638=CARTESIAN_POINT('Ctrl Pts',(0.732159228641372,0.473415334142076,
-11.7553295478875));
#67639=CARTESIAN_POINT('Ctrl Pts',(0.278907906557356,0.77482152142975,-11.7341474165617));
#67640=CARTESIAN_POINT('Ctrl Pts',(-0.126048629243606,0.815643351149952,
-11.7182608180673));
#67641=CARTESIAN_POINT('Ctrl Pts',(-0.499012654979741,0.655089673413841,
-11.7023742195729));
#67642=CARTESIAN_POINT('Ctrl Pts',(-0.841598877251412,0.229859144335204,
-11.681192088247));
#67643=CARTESIAN_POINT('Ctrl Pts',(-0.794557513494638,-0.360758464515903,
-11.6600099569212));
#67644=CARTESIAN_POINT('Ctrl Pts',(-0.388959906239125,-0.724940043166852,
-11.6388278255953));
#67645=CARTESIAN_POINT('Ctrl Pts',(0.136093872237789,-0.861229592104873,
-11.6176456942695));
#67646=CARTESIAN_POINT('Ctrl Pts',(0.789313025756584,-0.503610198143102,
-11.5911680301121));
#67647=CARTESIAN_POINT('Ctrl Pts',(0.849082786184241,0.392933716931585,
-11.5593948331234));
#67648=CARTESIAN_POINT('Ctrl Pts',(0.25176492241088,0.834790970545129,-11.532917168966));
#67649=CARTESIAN_POINT('Ctrl Pts',(-0.289087834282494,0.771116750379929,
-11.5117350376402));
#67650=CARTESIAN_POINT('Ctrl Pts',(-0.624034498747816,0.540076235369627,
-11.4958484391458));
#67651=CARTESIAN_POINT('Ctrl Pts',(-0.804439485071099,0.176267123032317,
-11.4799618406514));
#67652=CARTESIAN_POINT('Ctrl Pts',(-0.790240411000712,-0.369615224324265,
-11.4587797093255));
#67653=CARTESIAN_POINT('Ctrl Pts',(-0.372075622126741,-0.789325185240889,
-11.4375975779997));
#67654=CARTESIAN_POINT('Ctrl Pts',(0.172833538805439,-0.804336911067798,
-11.4164154466738));
#67655=CARTESIAN_POINT('Ctrl Pts',(0.661245923546358,-0.568320490261234,
-11.395233315348));
#67656=CARTESIAN_POINT('Ctrl Pts',(0.927621995011193,0.127116573399042,
-11.3687556511906));
#67657=CARTESIAN_POINT('Ctrl Pts',(0.392795607410976,0.849146302721704,
-11.3369824542019));
#67658=CARTESIAN_POINT('Ctrl Pts',(-0.348510610217431,0.799250627735656,
-11.3105047900445));
#67659=CARTESIAN_POINT('Ctrl Pts',(-0.71952459067659,0.400596402966526,
-11.2893226587187));
#67660=CARTESIAN_POINT('Ctrl Pts',(-0.825252913065406,0.00767089787905485,
-11.2734360602243));
#67661=CARTESIAN_POINT('Ctrl Pts',(-0.727243390108357,-0.386406665398893,
-11.2575494617299));
#67662=CARTESIAN_POINT('Ctrl Pts',(-0.363042629979021,-0.793281375912599,
-11.236367330404));
#67663=CARTESIAN_POINT('Ctrl Pts',(0.227378927841211,-0.842480462017667,
-11.2151851990782));
#67664=CARTESIAN_POINT('Ctrl Pts',(0.652421592475167,-0.501173997058855,
-11.1940030677523));
#67665=CARTESIAN_POINT('Ctrl Pts',(0.871899210482239,-0.00510950742898545,
-11.1728209364264));
#67666=CARTESIAN_POINT('Ctrl Pts',(0.624735747529702,0.697385430750005,
-11.1463432722691));
#67667=CARTESIAN_POINT('Ctrl Pts',(-0.250311713924867,0.901488701922009,
-11.1145700752803));
#67668=CARTESIAN_POINT('Ctrl Pts',(-0.783028415884914,0.38357230044019,
-11.088092411123));
#67669=CARTESIAN_POINT('Ctrl Pts',(-0.807742087698623,-0.160455087713699,
-11.0669102797971));
#67670=CARTESIAN_POINT('Ctrl Pts',(-0.633965965572041,-0.528382784897813,
-11.0510236813027));
#67671=CARTESIAN_POINT('Ctrl Pts',(-0.304156942230524,-0.765298382385843,
-11.0351370828084));
#67672=CARTESIAN_POINT('Ctrl Pts',(0.23682486235197,-0.839648305648038,
-11.0139549514825));
#67673=CARTESIAN_POINT('Ctrl Pts',(0.718687898942275,-0.494936571238069,
-10.9927728201567));
#67674=CARTESIAN_POINT('Ctrl Pts',(0.821705947496933,0.0403564807112435,
-10.9715906888308));
#67675=CARTESIAN_POINT('Ctrl Pts',(0.667861223009512,0.560531646820518,
-10.9504085575049));
#67676=CARTESIAN_POINT('Ctrl Pts',(0.0247137011057215,0.935964970627296,
-10.9239308933476));
#67677=CARTESIAN_POINT('Ctrl Pts',(-0.774366185017812,0.525066515148126,
-10.8921576963588));
#67678=CARTESIAN_POINT('Ctrl Pts',(-0.845123525583511,-0.214540057447401,
-10.8656800322015));
#67679=CARTESIAN_POINT('Ctrl Pts',(-0.511782611418673,-0.645191191867571,
-10.8444979008756));
#67680=CARTESIAN_POINT('Ctrl Pts',(-0.141153160795665,-0.81312791003465,
-10.8286113023812));
#67681=CARTESIAN_POINT('Ctrl Pts',(0.263592134007046,-0.780200132324299,
-10.8127247038868));
#67682=CARTESIAN_POINT('Ctrl Pts',(0.72405410023979,-0.486663079072112,
-10.791542572561));
#67683=CARTESIAN_POINT('Ctrl Pts',(0.868175704982164,0.0880082434404666,
-10.7703604412351));
#67684=CARTESIAN_POINT('Ctrl Pts',(0.600171861350475,0.562692675028197,
-10.7491783099093));
#67685=CARTESIAN_POINT('Ctrl Pts',(0.146176171072608,0.859573654376184,
-10.7279961785834));
#67686=CARTESIAN_POINT('Ctrl Pts',(-0.587062635494574,0.729382379325026,
-10.7015185144261));
#67687=CARTESIAN_POINT('Ctrl Pts',(-0.930117875491998,-0.101086950290881,
-10.6697453174373));
#67688=CARTESIAN_POINT('Ctrl Pts',(-0.505262363873941,-0.710613223488523,
-10.64326765328));
#67689=CARTESIAN_POINT('Ctrl Pts',(0.0275900749206337,-0.823062514745925,
-10.6220855219541));
#67690=CARTESIAN_POINT('Ctrl Pts',(0.41879467985798,-0.711134466189467,
-10.6061989234597));
#67691=CARTESIAN_POINT('Ctrl Pts',(0.705971949833696,-0.424024369154948,
-10.5903123249653));
#67692=CARTESIAN_POINT('Ctrl Pts',(0.866909909130173,0.0977880466003558,
-10.5691301936395));
#67693=CARTESIAN_POINT('Ctrl Pts',(0.604743199683794,0.629094721064296,
-10.5479480623136));
#67694=CARTESIAN_POINT('Ctrl Pts',(0.0931850144054718,0.817401897953224,
-10.5267659309878));
#67695=CARTESIAN_POINT('Ctrl Pts',(-0.445032952688861,0.749786643858178,
-10.5055837996619));
#67696=CARTESIAN_POINT('Ctrl Pts',(-0.919621199894597,0.175892131626442,
-10.4791061355046));
#67697=CARTESIAN_POINT('Ctrl Pts',(-0.64348842062255,-0.6791616054766,-10.4473329385158));
#67698=CARTESIAN_POINT('Ctrl Pts',(0.0749108584025137,-0.868705688387979,
-10.4208552743585));
#67699=CARTESIAN_POINT('Ctrl Pts',(0.553840414872343,-0.609470188170057,
-10.3996731430326));
#67700=CARTESIAN_POINT('Ctrl Pts',(0.779556078641138,-0.270912408600226,
-10.3837865445382));
#67701=CARTESIAN_POINT('Ctrl Pts',(0.812578539516615,0.133825172169838,
-10.3678999460438));
#67702=CARTESIAN_POINT('Ctrl Pts',(0.597447442438676,0.635729381206725,
-10.346717814718));
#67703=CARTESIAN_POINT('Ctrl Pts',(0.0536837211124086,0.870972194574707,
-10.3255356833921));
#67704=CARTESIAN_POINT('Ctrl Pts',(-0.458122336948451,0.683339764740917,
-10.3043535520663));
#67705=CARTESIAN_POINT('Ctrl Pts',(-0.824576230095092,0.2833873339605,-10.2831714207404));
#67706=CARTESIAN_POINT('Ctrl Pts',(-0.814791030660772,-0.461255644538286,
-10.2566937565831));
#67707=CARTESIAN_POINT('Ctrl Pts',(-0.0508040537562885,-0.934214526728624,
-10.2249205595943));
#67708=CARTESIAN_POINT('Ctrl Pts',(0.61945510051208,-0.613625772106911,
-10.1984428954369));
#67709=CARTESIAN_POINT('Ctrl Pts',(0.816674080954391,-0.106002645775066,
-10.1772607641111));
#67710=CARTESIAN_POINT('Ctrl Pts',(0.769546288077532,0.298160566450391,
-10.1613741656167));
#67711=CARTESIAN_POINT('Ctrl Pts',(0.532707850926748,0.62802500360276,-10.1454875671223));
#67712=CARTESIAN_POINT('Ctrl Pts',(0.0438279986233484,0.871306145475099,
-10.1243054357965));
#67713=CARTESIAN_POINT('Ctrl Pts',(-0.52290872124537,0.698599294932571,
-10.1031233044706));
#67714=CARTESIAN_POINT('Ctrl Pts',(-0.791538290376542,0.224268688307269,
-10.0819411731447));
#67715=CARTESIAN_POINT('Ctrl Pts',(-0.811935907224159,-0.31779619703067,
-10.0607590418189));
#67716=CARTESIAN_POINT('Ctrl Pts',(-0.322431281728496,-0.879021764137039,
-10.0342813776615));
#67717=CARTESIAN_POINT('Ctrl Pts',(0.566043654210065,-0.74493786006443,
-10.0025081806728));
#67718=CARTESIAN_POINT('Ctrl Pts',(0.869375119096715,-0.0666941679594714,
-9.97603051651542));
#67719=CARTESIAN_POINT('Ctrl Pts',(0.691082554031784,0.447881701933579,
-9.95484838518959));
#67720=CARTESIAN_POINT('Ctrl Pts',(0.393526148412095,0.72542289969084,-9.93896178669518));
#67721=CARTESIAN_POINT('Ctrl Pts',(-0.0005284759719869,0.823524608194793,
-9.92307518820079));
#67722=CARTESIAN_POINT('Ctrl Pts',(-0.530636846339506,0.692473703408921,
-9.90189305687493));
#67723=CARTESIAN_POINT('Ctrl Pts',(-0.850796171354358,0.193959739233485,
-9.88071092554907));
#67724=CARTESIAN_POINT('Ctrl Pts',(-0.74848409447556,-0.341468695496941,
-9.85952879422322));
#67725=CARTESIAN_POINT('Ctrl Pts',(-0.413123953802155,-0.767830019654057,
-9.83834666289735));
#67726=CARTESIAN_POINT('Ctrl Pts',(0.323282706987867,-0.878708987450492,
-9.81186899874004));
#67727=CARTESIAN_POINT('Ctrl Pts',(0.913670603537105,-0.201355064651968,
-9.78009580175124));
#67728=CARTESIAN_POINT('Ctrl Pts',(0.705804362960112,0.511958407461686,
-9.75361813759391));
#67729=CARTESIAN_POINT('Ctrl Pts',(0.23679947108692,0.788745285822342,-9.73243600626808));
#67730=CARTESIAN_POINT('Ctrl Pts',(-0.16966225545332,0.807660777773948,
-9.71654940777366));
#67731=CARTESIAN_POINT('Ctrl Pts',(-0.533513449991765,0.627340783200905,
-9.70066280927929));
#67732=CARTESIAN_POINT('Ctrl Pts',(-0.85272106081396,0.184288049125053,
-9.67948067795341));
#67733=CARTESIAN_POINT('Ctrl Pts',(-0.774029335533589,-0.40293063096293,
-9.65829854662756));
#67734=CARTESIAN_POINT('Ctrl Pts',(-0.349437115605602,-0.744797295862786,
-9.63711641530171));
#67735=CARTESIAN_POINT('Ctrl Pts',(0.18217734002223,-0.852669781961048,
-9.61593428397583));
#67736=CARTESIAN_POINT('Ctrl Pts',(0.815237502428397,-0.460466076815634,
-9.58945661981853));
#67737=CARTESIAN_POINT('Ctrl Pts',(0.82673903215434,0.437995897859057,-9.55768342282973));
#67738=CARTESIAN_POINT('Ctrl Pts',(0.206540088074968,0.847114160997335,
-9.5312057586724));
#67739=CARTESIAN_POINT('Ctrl Pts',(-0.33010978967523,0.754467124647978,
-9.51002362734656));
#67740=CARTESIAN_POINT('Ctrl Pts',(-0.652156174386574,0.505760355395116,
-9.49413702885215));
#67741=CARTESIAN_POINT('Ctrl Pts',(-0.812749627990668,0.132782159156536,
-9.47825043035777));
#67742=CARTESIAN_POINT('Ctrl Pts',(-0.769235476576637,-0.411548386197682,
-9.45706829903191));
#67743=CARTESIAN_POINT('Ctrl Pts',(-0.329119930899387,-0.808179792323179,
-9.43588616770604));
#67744=CARTESIAN_POINT('Ctrl Pts',(0.21580857366481,-0.793886622396449,
-9.4147040363802));
#67745=CARTESIAN_POINT('Ctrl Pts',(0.690831744825092,-0.531964134720561,
-9.39352190505433));
#67746=CARTESIAN_POINT('Ctrl Pts',(0.91945036799731,0.17678295747407,-9.36704424089702));
#67747=CARTESIAN_POINT('Ctrl Pts',(0.346595192110193,0.869027966543628,
-9.33527104390822));
#67748=CARTESIAN_POINT('Ctrl Pts',(-0.390958446283618,0.779366860357645,
-9.3087933797509));
#67749=CARTESIAN_POINT('Ctrl Pts',(-0.740012771240314,0.361350541462502,
-9.28761124842504));
#67750=CARTESIAN_POINT('Ctrl Pts',(-0.82447263842956,-0.0366889814648314,
-9.27172464993064));
#67751=CARTESIAN_POINT('Ctrl Pts',(-0.705427154896096,-0.424930098633222,
-9.25583805143626));
#67752=CARTESIAN_POINT('Ctrl Pts',(-0.319887370896094,-0.81164485000965,
-9.23465592011039));
#67753=CARTESIAN_POINT('Ctrl Pts',(0.272324957917033,-0.82904380036898,
-9.21347378878455));
#67754=CARTESIAN_POINT('Ctrl Pts',(0.678411741478122,-0.465388889759847,
-9.19229165745867));
#67755=CARTESIAN_POINT('Ctrl Pts',(0.870913883071089,0.0417534257410553,
-9.17110952613283));
#67756=CARTESIAN_POINT('Ctrl Pts',(0.586355750720453,0.72995077016243,-9.14463186197549));
#67757=CARTESIAN_POINT('Ctrl Pts',(-0.298395687321513,0.886734372637476,
-9.11285866498671));
#67758=CARTESIAN_POINT('Ctrl Pts',(-0.802509962736313,0.340938366062253,
-9.08638100082939));
#67759=CARTESIAN_POINT('Ctrl Pts',(-0.797952086762503,-0.203630996278515,
-9.06519886950353));
#67760=CARTESIAN_POINT('Ctrl Pts',(-0.604654772294215,-0.561688364862365,
-9.04931227100913));
#67761=CARTESIAN_POINT('Ctrl Pts',(-0.262590570136529,-0.780537796691881,
-9.03342567251473));
#67762=CARTESIAN_POINT('Ctrl Pts',(0.281605043851865,-0.825708115427715,
-9.0122435411889));
#67763=CARTESIAN_POINT('Ctrl Pts',(0.74424709487229,-0.45559934965813,-8.991061409863));
#67764=CARTESIAN_POINT('Ctrl Pts',(0.818349824448401,0.0844563467866882,
-8.96987927853718));
#67765=CARTESIAN_POINT('Ctrl Pts',(0.636773382186694,0.595612290022289,
-8.94869714721129));
#67766=CARTESIAN_POINT('Ctrl Pts',(-0.0256204313745529,0.935940589332386,
-8.92221948305399));
#67767=CARTESIAN_POINT('Ctrl Pts',(-0.801464097138213,0.482693624183378,
-8.89044628606519));
#67768=CARTESIAN_POINT('Ctrl Pts',(-0.832373000965563,-0.259646677251645,
-8.86396862190787));
#67769=CARTESIAN_POINT('Ctrl Pts',(-0.476370733590293,-0.671761892036649,
-8.84278649058203));
#67770=CARTESIAN_POINT('Ctrl Pts',(-0.0972519905765146,-0.819538445229283,
-8.82689989208761));
#67771=CARTESIAN_POINT('Ctrl Pts',(0.305138912861327,-0.764907382267323,
-8.81101329359324));
#67772=CARTESIAN_POINT('Ctrl Pts',(0.749160927417865,-0.447049435114738,
-8.78983116226736));
#67773=CARTESIAN_POINT('Ctrl Pts',(0.862191643692155,0.134536519882796,
-8.76864903094151));
#67774=CARTESIAN_POINT('Ctrl Pts',(0.56906570002938,0.59413259356591,-8.74746689961565));
#67775=CARTESIAN_POINT('Ctrl Pts',(0.0997717649227431,0.866187009375733,
-8.7262847682898));
#67776=CARTESIAN_POINT('Ctrl Pts',(-0.625411065729518,0.696779873508656,
-8.69980710413246));
#67777=CARTESIAN_POINT('Ctrl Pts',(-0.92334146161966,-0.150925077713834,
-8.66803390714369));
#67778=CARTESIAN_POINT('Ctrl Pts',(-0.466344151485975,-0.736738991854688,
-8.64155624298635));
#67779=CARTESIAN_POINT('Ctrl Pts',(0.0717812901244923,-0.820390493485922,
-8.62037411166051));
#67780=CARTESIAN_POINT('Ctrl Pts',(0.456405624116447,-0.687600988331753,
-8.6044875131661));
#67781=CARTESIAN_POINT('Ctrl Pts',(0.72773872432255,-0.385472967548476,
-8.58860091467172));
#67782=CARTESIAN_POINT('Ctrl Pts',(0.860402113835931,0.144234167632582,
-8.56741878334586));
#67783=CARTESIAN_POINT('Ctrl Pts',(0.57006201063428,0.660684349494034,-8.54623665201998));
#67784=CARTESIAN_POINT('Ctrl Pts',(0.0491234764725384,0.821228466230034,
-8.52505452069416));
#67785=CARTESIAN_POINT('Ctrl Pts',(-0.484683136277,0.724787277548224,-8.50387238936827));
#67786=CARTESIAN_POINT('Ctrl Pts',(-0.927744710107105,0.126217851875059,
-8.47739472521096));
#67787=CARTESIAN_POINT('Ctrl Pts',(-0.606060667659628,-0.712761040563262,
-8.44562152822217));
#67788=CARTESIAN_POINT('Ctrl Pts',(0.121486541926073,-0.863424710021134,
-8.41914386406484));
#67789=CARTESIAN_POINT('Ctrl Pts',(0.585792813827149,-0.578826307870058,
-8.397961732739));
#67790=CARTESIAN_POINT('Ctrl Pts',(0.792988341037864,-0.228627872005885,
-8.38207513424459));
#67791=CARTESIAN_POINT('Ctrl Pts',(0.804212631896132,0.177299470636368,
-8.36618853575021));
#67792=CARTESIAN_POINT('Ctrl Pts',(0.562420251644729,0.666917351060745,
-8.34500640442434));
#67793=CARTESIAN_POINT('Ctrl Pts',(0.00680041481536649,0.872598567494293,
-8.32382427309849));
#67794=CARTESIAN_POINT('Ctrl Pts',(-0.494182774760557,0.657732996600626,
-8.30264214177263));
#67795=CARTESIAN_POINT('Ctrl Pts',(-0.838613835539921,0.23866540412908,
-8.28146001044677));
#67796=CARTESIAN_POINT('Ctrl Pts',(-0.78882593018678,-0.504375698392214,
-8.25498234628944));
#67797=CARTESIAN_POINT('Ctrl Pts',(-0.000526288458951071,-0.935594761020664,
-8.22320914930067));
#67798=CARTESIAN_POINT('Ctrl Pts',(0.651536004617581,-0.579449777315683,
-8.19673148514333));
#67799=CARTESIAN_POINT('Ctrl Pts',(0.821190515837749,-0.0619616987512881,
-8.17554935381748));
#67800=CARTESIAN_POINT('Ctrl Pts',(0.752411237902168,0.339084859524061,
-8.15966275532308));
#67801=CARTESIAN_POINT('Ctrl Pts',(0.498188240520423,0.65574502407293,-8.1437761568287));
#67802=CARTESIAN_POINT('Ctrl Pts',(-0.00305901237357047,0.872402392849367,
-8.12259402550283));
#67803=CARTESIAN_POINT('Ctrl Pts',(-0.559695583195045,0.66948887950937,
-8.10141189417697));
#67804=CARTESIAN_POINT('Ctrl Pts',(-0.802446621511299,0.181407633004746,
-8.08022976285112));
#67805=CARTESIAN_POINT('Ctrl Pts',(-0.793684391543133,-0.36097011913437,
-8.05904763152525));
#67806=CARTESIAN_POINT('Ctrl Pts',(-0.274727049262383,-0.895078902481372,
-8.03256996736793));
#67807=CARTESIAN_POINT('Ctrl Pts',(0.605258403199313,-0.713442428781381,
-8.00079677037915));
#67808=CARTESIAN_POINT('Ctrl Pts',(0.871702976551815,-0.0198778875875173,
-7.97431910622182));
#67809=CARTESIAN_POINT('Ctrl Pts',(0.666014925458434,0.484373032363083,
-7.95313697489597));
#67810=CARTESIAN_POINT('Ctrl Pts',(0.353973530252757,0.745522603788999,
-7.93725037640157));
#67811=CARTESIAN_POINT('Ctrl Pts',(-0.0447836284226616,0.822306199790894,
-7.92136377790718));
#67812=CARTESIAN_POINT('Ctrl Pts',(-0.567083353921183,0.662956832917124,
-7.90018164658131));
#67813=CARTESIAN_POINT('Ctrl Pts',(-0.85999008173785,0.147957983722677,
-7.87899951525548));
#67814=CARTESIAN_POINT('Ctrl Pts',(-0.729052116288621,-0.381198532817697,
-7.85781738392959));
#67815=CARTESIAN_POINT('Ctrl Pts',(-0.371264073084344,-0.78892162368888,
-7.83663525260375));
#67816=CARTESIAN_POINT('Ctrl Pts',(0.370037062286983,-0.860066140362291,
-7.81015758844642));
#67817=CARTESIAN_POINT('Ctrl Pts',(0.923171081329685,-0.151963773398269,
-7.77838439145763));
#67818=CARTESIAN_POINT('Ctrl Pts',(0.677272002002691,0.549148290580514,
-7.75190672730032));
#67819=CARTESIAN_POINT('Ctrl Pts',(0.194070403631153,0.80033105265787,-7.73072459597444));
#67820=CARTESIAN_POINT('Ctrl Pts',(-0.212820489925012,0.797376104450092,
-7.71483799748006));
#67821=CARTESIAN_POINT('Ctrl Pts',(-0.56645558113332,0.597763443338712,
-7.69895139898567));
#67822=CARTESIAN_POINT('Ctrl Pts',(-0.861392436550393,0.138196826518483,
-7.6777692676598));
#67823=CARTESIAN_POINT('Ctrl Pts',(-0.751257501705145,-0.443944446712085,
-7.65658713633396));
#67824=CARTESIAN_POINT('Ctrl Pts',(-0.308907033835764,-0.762499674841944,
-7.63540500500809));
#67825=CARTESIAN_POINT('Ctrl Pts',(0.227736257654196,-0.841647513652085,
-7.61422287368224));
#67826=CARTESIAN_POINT('Ctrl Pts',(0.838804750428707,-0.415990124788927,
-7.58774520952491));
#67827=CARTESIAN_POINT('Ctrl Pts',(0.802006637013915,0.481791643778187,
-7.55597201253612));
#67828=CARTESIAN_POINT('Ctrl Pts',(0.160718023638984,0.856989455373761,
-7.5294943483788));
#67829=CARTESIAN_POINT('Ctrl Pts',(-0.370177566713595,0.735636924383227,
-7.50831221705294));
#67830=CARTESIAN_POINT('Ctrl Pts',(-0.678393176155383,0.469982884183816,
-7.49242561855855));
#67831=CARTESIAN_POINT('Ctrl Pts',(-0.818710855193977,0.0889134139305586,
-7.47653902006415));
#67832=CARTESIAN_POINT('Ctrl Pts',(-0.746007454897768,-0.45229212887575,
-7.4553568887383));
#67833=CARTESIAN_POINT('Ctrl Pts',(-0.285213055285053,-0.824698744227078,
-7.43417475741243));
#67834=CARTESIAN_POINT('Ctrl Pts',(0.258159907699396,-0.78114196644651,
-7.41299262608659));
#67835=CARTESIAN_POINT('Ctrl Pts',(0.71842104135087,-0.494070387324931,
-7.39181049476071));
#67836=CARTESIAN_POINT('Ctrl Pts',(0.90862149268301,0.225938434751966,-7.3653328306034));
#67837=CARTESIAN_POINT('Ctrl Pts',(0.299393105433013,0.886398105959188,
-7.33355963361461));
#67838=CARTESIAN_POINT('Ctrl Pts',(-0.432276398724546,0.75723069460368,
-7.30708196945729));
#67839=CARTESIAN_POINT('Ctrl Pts',(-0.758362287164713,0.321060363203428,
-7.28589983813143));
#67840=CARTESIAN_POINT('Ctrl Pts',(-0.821309607551199,-0.0809428281197334,
-7.27001323963704));
#67841=CARTESIAN_POINT('Ctrl Pts',(-0.681572209011577,-0.462225468242849,
-7.25412664114264));
#67842=CARTESIAN_POINT('Ctrl Pts',(-0.27580762554856,-0.827662640388744,
-7.23294450981678));
#67843=CARTESIAN_POINT('Ctrl Pts',(0.316483958824071,-0.81321117149348,
-7.21176237849093));
#67844=CARTESIAN_POINT('Ctrl Pts',(0.702441255430704,-0.428258791335588,
-7.19058024716506));
#67845=CARTESIAN_POINT('Ctrl Pts',(0.867411582321966,0.0884956899559494,
-7.16939811583921));
#67846=CARTESIAN_POINT('Ctrl Pts',(0.54628116408828,0.760406524844457,-7.14292045168187));
#67847=CARTESIAN_POINT('Ctrl Pts',(-0.345617286136612,0.869417348200748,
-7.11114725469311));
#67848=CARTESIAN_POINT('Ctrl Pts',(-0.819672226101789,0.297319107192211,
-7.08466959053576));
#67849=CARTESIAN_POINT('Ctrl Pts',(-0.785855974768107,-0.24621840372986,
-7.06348745920993));
#67850=CARTESIAN_POINT('Ctrl Pts',(-0.573596104350783,-0.593370644667842,
-7.04760086071551));
#67851=CARTESIAN_POINT('Ctrl Pts',(-0.220265301577946,-0.793521427883344,
-7.03171426222114));
#67852=CARTESIAN_POINT('Ctrl Pts',(0.325571376354598,-0.809381598199867,
-7.01053213089526));
#67853=CARTESIAN_POINT('Ctrl Pts',(0.767655389158747,-0.414945429099158,
-6.98934999956942));
#67854=CARTESIAN_POINT('Ctrl Pts',(0.812628640125686,0.128312130894811,
-6.96816786824355));
#67855=CARTESIAN_POINT('Ctrl Pts',(0.603845242726765,0.628971591666356,
-6.9469857369177));
#67856=CARTESIAN_POINT('Ctrl Pts',(-0.0758805198601191,0.933211305101612,
-6.92050807276037));
#67857=CARTESIAN_POINT('Ctrl Pts',(-0.826245748361245,0.438925730783531,
-6.88873487577159));
#67858=CARTESIAN_POINT('Ctrl Pts',(-0.817216887574368,-0.304002908550855,
-6.86225721161426));
#67859=CARTESIAN_POINT('Ctrl Pts',(-0.439582126714707,-0.696391175480518,
-6.8410750802884));
#67860=CARTESIAN_POINT('Ctrl Pts',(-0.0530697585057933,-0.823580483991598,
-6.82518848179402));
#67861=CARTESIAN_POINT('Ctrl Pts',(0.345803828966025,-0.747404021571874,
-6.80930188329962));
#67862=CARTESIAN_POINT('Ctrl Pts',(0.772102651795132,-0.406143801747123,
-6.78811975197376));
#67863=CARTESIAN_POINT('Ctrl Pts',(0.853715816646702,0.180675980803334,
-6.7669376206479));
#67864=CARTESIAN_POINT('Ctrl Pts',(0.536314917779641,0.623855446924663,
-6.74575548932204));
#67865=CARTESIAN_POINT('Ctrl Pts',(0.0530790146765816,0.870297051863717,
-6.72457335799618));
#67866=CARTESIAN_POINT('Ctrl Pts',(-0.661952034834192,0.662163648080895,
-6.69809569383887));
#67867=CARTESIAN_POINT('Ctrl Pts',(-0.91389655677108,-0.200327026088165,
-6.66632249685007));
#67868=CARTESIAN_POINT('Ctrl Pts',(-0.426078187219746,-0.760735557254639,
-6.63984483269276));
#67869=CARTESIAN_POINT('Ctrl Pts',(0.115765054710094,-0.815347513367804,
-6.61866270136689));
#67870=CARTESIAN_POINT('Ctrl Pts',(0.492697539306155,-0.662080318119721,
-6.6027761028725));
#67871=CARTESIAN_POINT('Ctrl Pts',(0.747402306832701,-0.345807534904014,
-6.5868895043781));
#67872=CARTESIAN_POINT('Ctrl Pts',(0.851407724907275,0.190263446815729,
-6.56570737305224));
#67873=CARTESIAN_POINT('Ctrl Pts',(0.533733320681469,0.690364575260483,
-6.54452524172639));
#67874=CARTESIAN_POINT('Ctrl Pts',(0.00491997057463909,0.822681654372687,
-6.52334311040053));
#67875=CARTESIAN_POINT('Ctrl Pts',(-0.522932569302915,0.697693247967738,
-6.50216097907467));
#67876=CARTESIAN_POINT('Ctrl Pts',(-0.933187000294144,0.0761788004565664,
-6.47568331491735));
#67877=CARTESIAN_POINT('Ctrl Pts',(-0.566881383083514,-0.744300574444075,
-6.44391011792856));
#67878=CARTESIAN_POINT('Ctrl Pts',(0.167711135250459,-0.85564839454374,
-6.41743245377124));
#67879=CARTESIAN_POINT('Ctrl Pts',(0.616052235469796,-0.546509608852112,
-6.39625032244538));
#67880=CARTESIAN_POINT('Ctrl Pts',(0.804128869206457,-0.185682568995067,
-6.38036372395099));
#67881=CARTESIAN_POINT('Ctrl Pts',(0.793522461442759,0.220261323442116,
-6.36447712545659));
#67882=CARTESIAN_POINT('Ctrl Pts',(0.525767779146774,0.696178004642138,
-6.34329499413073));
#67883=CARTESIAN_POINT('Ctrl Pts',(-0.0401028011771158,0.871702907377351,
-6.32211286280489));
#67884=CARTESIAN_POINT('Ctrl Pts',(-0.528814706483476,0.630225578934503,
-6.30093073147902));
#67885=CARTESIAN_POINT('Ctrl Pts',(-0.850228516581944,0.193253200532271,
-6.27974860015315));
#67886=CARTESIAN_POINT('Ctrl Pts',(-0.760579602040354,-0.546036976699944,
-6.25327093599584));
#67887=CARTESIAN_POINT('Ctrl Pts',(0.0497503680220317,-0.93427305088848,
-6.22149773900705));
#67888=CARTESIAN_POINT('Ctrl Pts',(0.681738399204437,-0.543595833521218,
-6.19502007484973));
#67889=CARTESIAN_POINT('Ctrl Pts',(0.823327512862196,-0.017746274093434,
-6.17383794352387));
#67890=CARTESIAN_POINT('Ctrl Pts',(0.733115143655037,0.379039205950285,
-6.15795134502948));
#67891=CARTESIAN_POINT('Ctrl Pts',(0.462203772512288,0.68155123760968,-6.14206474653508));
#67892=CARTESIAN_POINT('Ctrl Pts',(-0.0498799697013847,0.871019985612516,
-6.12088261520922));
#67893=CARTESIAN_POINT('Ctrl Pts',(-0.594974604645952,0.638361893885933,
-6.09970048388337));
#67894=CARTESIAN_POINT('Ctrl Pts',(-0.810907624869373,0.138117835093518,
-6.0785183525575));
#67895=CARTESIAN_POINT('Ctrl Pts',(-0.77343850503288,-0.403324024697871,
-6.05733622123165));
#67896=CARTESIAN_POINT('Ctrl Pts',(-0.225596939568173,-0.908076555586584,
-6.03085855707432));
#67897=CARTESIAN_POINT('Ctrl Pts',(0.641639344974892,-0.680705173610852,
-5.99908536008554));
#67898=CARTESIAN_POINT('Ctrl Pts',(0.919468928149147,0.170110871229085,
-5.96731216309674));
#67899=CARTESIAN_POINT('Ctrl Pts',(0.35533929095156,0.864924740453239,-5.93553896610797));
#67900=CARTESIAN_POINT('Ctrl Pts',(-0.534401559546241,0.767773114634092,
-5.90376576911917));
#67901=CARTESIAN_POINT('Ctrl Pts',(-0.935052121943657,-0.0342715508429932,
-5.87199257213039));
#67902=CARTESIAN_POINT('Ctrl Pts',(-0.55358600282851,-0.674106762641006,
-5.84551490797307));
#67903=CARTESIAN_POINT('Ctrl Pts',(-0.0313842813866094,-0.821987067613631,
-5.82433277664721));
#67904=CARTESIAN_POINT('Ctrl Pts',(0.502545841796061,-0.71340617086813,
-5.80315064532135));
#67905=CARTESIAN_POINT('Ctrl Pts',(0.842203744665662,-0.227720616512817,
-5.78196851399549));
#67906=CARTESIAN_POINT('Ctrl Pts',(0.76195469850279,0.312361095915287,-5.76078638266963));
#67907=CARTESIAN_POINT('Ctrl Pts',(0.521536699949039,0.639631146919876,
-5.74489978417524));
#67908=CARTESIAN_POINT('Ctrl Pts',(0.151740387604851,0.809418296339771,
-5.72901318568084));
#67909=CARTESIAN_POINT('Ctrl Pts',(-0.391979347919493,0.778855484654289,
-5.70783105435499));
#67910=CARTESIAN_POINT('Ctrl Pts',(-0.90413480588984,0.240585713443955,
-5.68135339019766));
#67911=CARTESIAN_POINT('Ctrl Pts',(-0.690614991381718,-0.632209336092332,
-5.64958019320888));
#67912=CARTESIAN_POINT('Ctrl Pts',(0.0144991791284147,-0.871794186565672,
-5.62310252905155));
#67913=CARTESIAN_POINT('Ctrl Pts',(0.508171989488816,-0.646985705588241,
-5.60192039772569));
#67914=CARTESIAN_POINT('Ctrl Pts',(0.844880298461512,-0.218292177285309,
-5.58073826639983));
#67915=CARTESIAN_POINT('Ctrl Pts',(0.789325408565671,0.371565567738826,
-5.55955613507398));
#67916=CARTESIAN_POINT('Ctrl Pts',(0.378551563372044,0.731362879347338,
-5.53837400374811));
#67917=CARTESIAN_POINT('Ctrl Pts',(-0.0165586512023453,0.825122455027266,
-5.52248740525373));
#67918=CARTESIAN_POINT('Ctrl Pts',(-0.408322682801,0.71516829914728,-5.50660080675932));
#67919=CARTESIAN_POINT('Ctrl Pts',(-0.802957826126081,0.339882228772198,
-5.48541867543348));
#67920=CARTESIAN_POINT('Ctrl Pts',(-0.844866528645535,-0.401918395173574,
-5.45894101127615));
#67921=CARTESIAN_POINT('Ctrl Pts',(-0.117118420384341,-0.928937276011495,
-5.42716781428736));
#67922=CARTESIAN_POINT('Ctrl Pts',(0.575409343140774,-0.655086580631771,
-5.40069015013004));
#67923=CARTESIAN_POINT('Ctrl Pts',(0.806151735036186,-0.164160563625932,
-5.37950801880418));
#67924=CARTESIAN_POINT('Ctrl Pts',(0.785272019256606,0.380555331263283,
-5.35832588747833));
#67925=CARTESIAN_POINT('Ctrl Pts',(0.361082683504556,0.794175414438857,
-5.33714375615246));
#67926=CARTESIAN_POINT('Ctrl Pts',(-0.184920996590559,0.802494413983792,
-5.31596162482661));
#67927=CARTESIAN_POINT('Ctrl Pts',(-0.546765877871137,0.618181435887277,
-5.30007502633221));
#67928=CARTESIAN_POINT('Ctrl Pts',(-0.774185727665808,0.280766049453372,
-5.28418842783782));
#67929=CARTESIAN_POINT('Ctrl Pts',(-0.832030667120703,-0.260741593664439,
-5.26300629651196));
#67930=CARTESIAN_POINT('Ctrl Pts',(-0.383766661157618,-0.853264896525865,
-5.23652863235464));
#67931=CARTESIAN_POINT('Ctrl Pts',(0.512083211324558,-0.783844358237307,
-5.20475543536584));
#67932=CARTESIAN_POINT('Ctrl Pts',(0.862643602471831,-0.126808341193055,
-5.17827777120853));
#67933=CARTESIAN_POINT('Ctrl Pts',(0.720711187517118,0.396742604062407,
-5.15709563988266));
#67934=CARTESIAN_POINT('Ctrl Pts',(0.352173705763636,0.798403523665007,
-5.13591350855682));
#67935=CARTESIAN_POINT('Ctrl Pts',(-0.238897473515934,0.839060957114792,
-5.11473137723095));
#67936=CARTESIAN_POINT('Ctrl Pts',(-0.660441788609072,0.491944817482841,
-5.0935492459051));
#67937=CARTESIAN_POINT('Ctrl Pts',(-0.816921181151555,0.117221997362471,
-5.0776626474107));
#67938=CARTESIAN_POINT('Ctrl Pts',(-0.771831834158657,-0.287173702127205,
-5.0617760489163));
#67939=CARTESIAN_POINT('Ctrl Pts',(-0.465374430984834,-0.737351916475205,
-5.04059391759045));
#67940=CARTESIAN_POINT('Ctrl Pts',(0.259859673417111,-0.898782945966624,
-5.01411625343313));
#67941=CARTESIAN_POINT('Ctrl Pts',(0.897728665382349,-0.265940663710014,
-4.98234305644434));
#67942=CARTESIAN_POINT('Ctrl Pts',(0.73958871850454,0.461782273098336,-4.95586539228701));
#67943=CARTESIAN_POINT('Ctrl Pts',(0.292487162343539,0.768947702741554,
-4.93468326096116));
#67944=CARTESIAN_POINT('Ctrl Pts',(-0.248424891230033,0.836516335197404,
-4.91350112963529));
#67945=CARTESIAN_POINT('Ctrl Pts',(-0.725253603938613,0.48487369755438,
-4.89231899830945));
#67946=CARTESIAN_POINT('Ctrl Pts',(-0.821844335556061,-0.0525827700264955,
-4.87113686698358));
#67947=CARTESIAN_POINT('Ctrl Pts',(-0.698533765966645,-0.439490376099843,
-4.85525026848919));
#67948=CARTESIAN_POINT('Ctrl Pts',(-0.402380543885497,-0.718528366396501,
-4.83936366999479));
#67949=CARTESIAN_POINT('Ctrl Pts',(0.122622432224616,-0.863264124622093,
-4.81818153866894));
#67950=CARTESIAN_POINT('Ctrl Pts',(0.779891974379151,-0.516823318096077,
-4.79170387451161));
#67951=CARTESIAN_POINT('Ctrl Pts',(0.856397877334779,0.378449295097978,
-4.75993067752283));
#67952=CARTESIAN_POINT('Ctrl Pts',(0.264771855760648,0.830740756604694,
-4.7334530133655));
#67953=CARTESIAN_POINT('Ctrl Pts',(-0.274849129440295,0.775427150500415,
-4.71227088203965));
#67954=CARTESIAN_POINT('Ctrl Pts',(-0.730868047059991,0.476766613157286,
-4.69108875071378));
#67955=CARTESIAN_POINT('Ctrl Pts',(-0.866665799372539,-0.0999283983858467,
-4.66990661938793));
#67956=CARTESIAN_POINT('Ctrl Pts',(-0.592362621446505,-0.572101026307649,
-4.64872448806207));
#67957=CARTESIAN_POINT('Ctrl Pts',(-0.247910861504431,-0.787173054434702,
-4.63283788956768));
#67958=CARTESIAN_POINT('Ctrl Pts',(0.158450323706088,-0.808137742177314,
-4.61695129107328));
#67959=CARTESIAN_POINT('Ctrl Pts',(0.652297814424352,-0.578592059262353,
-4.59576915974742));
#67960=CARTESIAN_POINT('Ctrl Pts',(0.92899332781192,0.110946972512963,-4.5692914955901));
#67961=CARTESIAN_POINT('Ctrl Pts',(0.407748529104943,0.842841818063406,
-4.53751829860131));
#67962=CARTESIAN_POINT('Ctrl Pts',(-0.335975364728725,0.804583677800187,
-4.51104063444399));
#67963=CARTESIAN_POINT('Ctrl Pts',(-0.711462127024278,0.413099202973537,
-4.48985850311813));
#67964=CARTESIAN_POINT('Ctrl Pts',(-0.865696935631178,-0.109742067018724,
-4.46867637179227));
#67965=CARTESIAN_POINT('Ctrl Pts',(-0.595875822308961,-0.637202712638309,
-4.44749424046642));
#67966=CARTESIAN_POINT('Ctrl Pts',(-0.0811423644714603,-0.819517526522297,
-4.42631210914056));
#67967=CARTESIAN_POINT('Ctrl Pts',(0.320623002143957,-0.760461769832068,
-4.41042551064616));
#67968=CARTESIAN_POINT('Ctrl Pts',(0.643919307037497,-0.513381964465409,
-4.39453891215177));
#67969=CARTESIAN_POINT('Ctrl Pts',(0.871728375130321,-0.0187309833400292,
-4.37335678082591));
#67970=CARTESIAN_POINT('Ctrl Pts',(0.636248391432616,0.685948845197852,
-4.34687911666859));
#67971=CARTESIAN_POINT('Ctrl Pts',(-0.234833508809209,0.906363291624296,
-4.3151059196798));
#67972=CARTESIAN_POINT('Ctrl Pts',(-0.776926530790784,0.395751823799299,
-4.28862825552248));
#67973=CARTESIAN_POINT('Ctrl Pts',(-0.809690669352921,-0.145706313007025,
-4.26744612419662));
#67974=CARTESIAN_POINT('Ctrl Pts',(-0.588784461095656,-0.644055404454502,
-4.24626399287076));
#67975=CARTESIAN_POINT('Ctrl Pts',(-0.0416763595216752,-0.871411713062787,
-4.22508186154491));
#67976=CARTESIAN_POINT('Ctrl Pts',(0.46867069141285,-0.677156438793757,
-4.20389973021904));
#67977=CARTESIAN_POINT('Ctrl Pts',(0.736662676991888,-0.372060899863277,
-4.18801313172465));
#67978=CARTESIAN_POINT('Ctrl Pts',(0.82312844087892,0.0255477049898826,
-4.17212653323026));
#67979=CARTESIAN_POINT('Ctrl Pts',(0.676548909322497,0.550038892296514,
-4.1509444019044));
#67980=CARTESIAN_POINT('Ctrl Pts',(0.0408920339190606,0.934700848074303,
-4.12446673774708));
#67981=CARTESIAN_POINT('Ctrl Pts',(-0.765724416674785,0.538801736236745,
-4.09269354075828));
#67982=CARTESIAN_POINT('Ctrl Pts',(-0.848357168761416,-0.201306866495383,
-4.06621587660097));
#67983=CARTESIAN_POINT('Ctrl Pts',(-0.522815457501024,-0.635211230289008,
-4.04503374527511));
#67984=CARTESIAN_POINT('Ctrl Pts',(-0.0318352824786834,-0.872044161969022,
-4.02385161394925));
#67985=CARTESIAN_POINT('Ctrl Pts',(0.532345145336561,-0.691161297269021,
-4.00266948262338));
#67986=CARTESIAN_POINT('Ctrl Pts',(0.795575358243202,-0.212727311235401,
-3.98148735129753));
#67987=CARTESIAN_POINT('Ctrl Pts',(0.802332052153671,0.193298967836865,
-3.96560075280314));
#67988=CARTESIAN_POINT('Ctrl Pts',(0.6108425695864,0.552326416709447,-3.94971415430875));
#67989=CARTESIAN_POINT('Ctrl Pts',(0.159590355860081,0.857200168024185,
-3.92853202298289));
#67990=CARTESIAN_POINT('Ctrl Pts',(-0.573913326002876,0.738891959670137,
-3.90205435882556));
#67991=CARTESIAN_POINT('Ctrl Pts',(-0.932422727675164,-0.0850238212413381,
-3.87028116183678));
#67992=CARTESIAN_POINT('Ctrl Pts',(-0.516293555233426,-0.702620313620022,
-3.84380349767945));
#67993=CARTESIAN_POINT('Ctrl Pts',(0.0127203886498161,-0.8225980193265,
-3.8226213663536));
#67994=CARTESIAN_POINT('Ctrl Pts',(0.540255341213515,-0.685272698949131,
-3.80143923502774));
#67995=CARTESIAN_POINT('Ctrl Pts',(0.853173521326546,-0.182181873723091,
-3.78025710370187));
#67996=CARTESIAN_POINT('Ctrl Pts',(0.744089772117057,0.352878832774126,
-3.75907497237603));
#67997=CARTESIAN_POINT('Ctrl Pts',(0.486397566632872,0.666722296052527,
-3.74318837388162));
#67998=CARTESIAN_POINT('Ctrl Pts',(0.108028752666176,0.816408539893724,
-3.72730177538723));
#67999=CARTESIAN_POINT('Ctrl Pts',(-0.433272302094322,0.756661299381776,
-3.70611964406138));
#68000=CARTESIAN_POINT('Ctrl Pts',(-0.915754966836196,0.19165248379213,
-3.67964197990405));
#68001=CARTESIAN_POINT('Ctrl Pts',(-0.655643663299691,-0.66841048767852,
-3.64786878291526));
#68002=CARTESIAN_POINT('Ctrl Pts',(0.0613287560853172,-0.869754634344714,
-3.62139111875794));
#68003=CARTESIAN_POINT('Ctrl Pts',(0.542206184319571,-0.61874208146278,
-3.60020898743208));
#68004=CARTESIAN_POINT('Ctrl Pts',(0.855390601589418,-0.172572953695659,
-3.57902685610623));
#68005=CARTESIAN_POINT('Ctrl Pts',(0.768216900074508,0.413446595155793,
-3.55784472478036));
#68006=CARTESIAN_POINT('Ctrl Pts',(0.338701423447491,0.7506493224828,-3.53666259345451));
#68007=CARTESIAN_POINT('Ctrl Pts',(-0.060876535391473,0.823040254373167,
-3.52077599496011));
#68008=CARTESIAN_POINT('Ctrl Pts',(-0.446165523219212,0.692191766279071,
-3.50488939646573));
#68009=CARTESIAN_POINT('Ctrl Pts',(-0.820062695127696,0.296240418923788,
-3.48370726513986));
#68010=CARTESIAN_POINT('Ctrl Pts',(-0.822046725490525,-0.446740433517228,
-3.45722960098254));
#68011=CARTESIAN_POINT('Ctrl Pts',(-0.0670284302510913,-0.933888849275838,
-3.42545640399375));
#68012=CARTESIAN_POINT('Ctrl Pts',(0.609781984565828,-0.623217675925539,
-3.39897873983643));
#68013=CARTESIAN_POINT('Ctrl Pts',(0.813808759860016,-0.120601045030234,
-3.37779660851058));
#68014=CARTESIAN_POINT('Ctrl Pts',(0.763686380628467,0.422205658035691,
-3.35661447718471));
#68015=CARTESIAN_POINT('Ctrl Pts',(0.317882211072159,0.812432269478428,
-3.33543234585885));
#68016=CARTESIAN_POINT('Ctrl Pts',(-0.227779543246364,0.791397207012838,
-3.314250214533));
#68017=CARTESIAN_POINT('Ctrl Pts',(-0.57919663904568,0.587905150681739,
-3.2983636160386));
#68018=CARTESIAN_POINT('Ctrl Pts',(-0.788155281402872,0.238755874924095,
-3.28247701754421));
#68019=CARTESIAN_POINT('Ctrl Pts',(-0.816816208015877,-0.305077845912804,
-3.26129488621835));
#68020=CARTESIAN_POINT('Ctrl Pts',(-0.337357962717805,-0.872655395227547,
-3.23481722206102));
#68021=CARTESIAN_POINT('Ctrl Pts',(0.553466755356614,-0.755192521135302,
-3.20304402507224));
#68022=CARTESIAN_POINT('Ctrl Pts',(0.868211701134554,-0.0802669440064075,
-3.17656636091491));
#68023=CARTESIAN_POINT('Ctrl Pts',(0.698348941736522,0.434900063535014,
-3.15538422958906));
#68024=CARTESIAN_POINT('Ctrl Pts',(0.308758890179159,0.816175504024769,
-3.1342020982632));
#68025=CARTESIAN_POINT('Ctrl Pts',(-0.283643096155971,0.825010234245042,
-3.11301996693734));
#68026=CARTESIAN_POINT('Ctrl Pts',(-0.685924375475703,0.455742044052894,
-3.09183783561148));
#68027=CARTESIAN_POINT('Ctrl Pts',(-0.822040182887849,0.0731515590922672,
-3.07595123711709));
#68028=CARTESIAN_POINT('Ctrl Pts',(-0.755283911462092,-0.328236695846971,
-3.06006463862269));
#68029=CARTESIAN_POINT('Ctrl Pts',(-0.425076929658484,-0.761295483775094,
-3.03888250729684));
#68030=CARTESIAN_POINT('Ctrl Pts',(0.307784443480434,-0.88351942263897,
-3.01240484313951));
#68031=CARTESIAN_POINT('Ctrl Pts',(0.910722986423459,-0.217312759090691,
-2.98063164615073));
#68032=CARTESIAN_POINT('Ctrl Pts',(0.713703985933684,0.500860220769669,
-2.9541539819934));
#68033=CARTESIAN_POINT('Ctrl Pts',(0.250741540134446,0.783554713940442,
-2.93297185066755));
#68034=CARTESIAN_POINT('Ctrl Pts',(-0.293019999508349,0.821957289354433,
-2.91178971934168));
#68035=CARTESIAN_POINT('Ctrl Pts',(-0.750262537092754,0.445198178389288,
-2.89060758801583));
#68036=CARTESIAN_POINT('Ctrl Pts',(-0.817830976145884,-0.0966724058121645,
-2.86942545668997));
#68037=CARTESIAN_POINT('Ctrl Pts',(-0.673906317084987,-0.476394257598558,
-2.85353885819558));
#68038=CARTESIAN_POINT('Ctrl Pts',(-0.363185640699209,-0.739113865249405,
-2.83765225970118));
#68039=CARTESIAN_POINT('Ctrl Pts',(0.168836743962548,-0.855427006606851,
-2.81647012837533));
#68040=CARTESIAN_POINT('Ctrl Pts',(0.806538915188326,-0.474165384771702,
-2.789992464218));
#68041=CARTESIAN_POINT('Ctrl Pts',(0.834822637619531,0.423924942627393,
-2.75821926722922));
#68042=CARTESIAN_POINT('Ctrl Pts',(0.219745546203246,0.84376906509478,-2.73174160307189));
#68043=CARTESIAN_POINT('Ctrl Pts',(-0.316123143402194,0.759536350606603,
-2.71055947174603));
#68044=CARTESIAN_POINT('Ctrl Pts',(-0.75543319544171,0.436801090726061,
-2.68937734042018));
#68045=CARTESIAN_POINT('Ctrl Pts',(-0.860043335086644,-0.146358308199602,
-2.66819520909432));
#68046=CARTESIAN_POINT('Ctrl Pts',(-0.560762143209286,-0.603107683861325,
-2.64701307776846));
#68047=CARTESIAN_POINT('Ctrl Pts',(-0.205250229032953,-0.799358215296395,
-2.63112647927406));
#68048=CARTESIAN_POINT('Ctrl Pts',(0.201650391521991,-0.798454904808682,
-2.61523988077967));
#68049=CARTESIAN_POINT('Ctrl Pts',(0.682448561078831,-0.542701733206808,
-2.59405774945381));
#68050=CARTESIAN_POINT('Ctrl Pts',(0.921688664885592,0.160710419233701,
-2.56758008529649));
#68051=CARTESIAN_POINT('Ctrl Pts',(0.361865308920915,0.863536155272751,
-2.53580688830771));
#68052=CARTESIAN_POINT('Ctrl Pts',(-0.378727911435124,0.785365844296184,
-2.50932922415038));
#68053=CARTESIAN_POINT('Ctrl Pts',(-0.732633853606216,0.374268548287705,
-2.48814709282452));
#68054=CARTESIAN_POINT('Ctrl Pts',(-0.858548488350327,-0.156105729510895,
-2.46696496149866));
#68055=CARTESIAN_POINT('Ctrl Pts',(-0.560771726234211,-0.668304095200904,
-2.44578283017281));
#68056=CARTESIAN_POINT('Ctrl Pts',(-0.0369845352724926,-0.822693870002639,
-2.42460069884694));
#68057=CARTESIAN_POINT('Ctrl Pts',(0.361026637840914,-0.742132723742336,
-2.40871410035255));
#68058=CARTESIAN_POINT('Ctrl Pts',(0.67057779376091,-0.478036126175377,
-2.39282750185816));
#68059=CARTESIAN_POINT('Ctrl Pts',(0.87147530780448,0.0281424524752154,
-2.3716453705323));
#68060=CARTESIAN_POINT('Ctrl Pts',(0.598466356625525,0.71914939603411,-2.34516770637498));
#68061=CARTESIAN_POINT('Ctrl Pts',(-0.283201807191348,0.892433711637579,
-2.31339450938619));
#68062=CARTESIAN_POINT('Ctrl Pts',(-0.797071418183535,0.353428202895539,
-2.28691684522887));
#68063=CARTESIAN_POINT('Ctrl Pts',(-0.80069044652496,-0.189008249901802,
-2.26573471390301));
#68064=CARTESIAN_POINT('Ctrl Pts',(-0.553322350976712,-0.674765797550789,
-2.24455258257715));
#68065=CARTESIAN_POINT('Ctrl Pts',(0.00521321548111552,-0.872392179578859,
-2.22337045125129));
#68066=CARTESIAN_POINT('Ctrl Pts',(0.504383596946202,-0.650991740900647,
-2.20218831992543));
#68067=CARTESIAN_POINT('Ctrl Pts',(0.755592604670905,-0.331935277797579,
-2.18630172143104));
#68068=CARTESIAN_POINT('Ctrl Pts',(0.820566080579593,0.0697454143027238,
-2.17041512293665));
#68069=CARTESIAN_POINT('Ctrl Pts',(0.646012391484676,0.585601570858967,
-2.14923299161079));
#68070=CARTESIAN_POINT('Ctrl Pts',(-0.00939754306034187,0.935547711243679,
-2.12275532745346));
#68071=CARTESIAN_POINT('Ctrl Pts',(-0.793572942149156,0.496873403144509,
-2.09098213046468));
#68072=CARTESIAN_POINT('Ctrl Pts',(-0.836313118389196,-0.246606383326159,
-2.06450446630735));
#68073=CARTESIAN_POINT('Ctrl Pts',(-0.487923956549996,-0.662389252865625,
-2.0433223349815));
#68074=CARTESIAN_POINT('Ctrl Pts',(0.0150740595623384,-0.872494858645637,
-2.02214020365564));
#68075=CARTESIAN_POINT('Ctrl Pts',(0.568718656160876,-0.661554519854988,
-2.00095807232978));
#68076=CARTESIAN_POINT('Ctrl Pts',(0.805857626289395,-0.169665982861812,
-1.97977594100392));
#68077=CARTESIAN_POINT('Ctrl Pts',(0.790784850518842,0.23613668302452,-1.96388934250953));
#68078=CARTESIAN_POINT('Ctrl Pts',(0.580278067886322,0.584354754703108,
-1.94800274401513));
#68079=CARTESIAN_POINT('Ctrl Pts',(0.113294116267464,0.864537826218961,
-1.92682061268928));
#68080=CARTESIAN_POINT('Ctrl Pts',(-0.612791798659163,0.706982351494664,
-1.90034294853195));
#68081=CARTESIAN_POINT('Ctrl Pts',(-0.926506210023761,-0.135009022109928,
-1.86856975154316));
#68082=CARTESIAN_POINT('Ctrl Pts',(-0.47778893867,-0.729350444143057,-1.84209208738584));
#68083=CARTESIAN_POINT('Ctrl Pts',(0.0569081290087825,-0.820725760860472,
-1.82090995605998));
#68084=CARTESIAN_POINT('Ctrl Pts',(0.576300970503701,-0.655249339588559,
-1.79972782473412));
#68085=CARTESIAN_POINT('Ctrl Pts',(0.861731058140963,-0.136069379513772,
-1.77854569340827));
#68086=CARTESIAN_POINT('Ctrl Pts',(0.724050967135742,0.39235603293315,-1.75736356208241));
#68087=CARTESIAN_POINT('Ctrl Pts',(0.449865296872678,0.691897700205439,
-1.74147696358801));
#68088=CARTESIAN_POINT('Ctrl Pts',(0.0639991479615115,0.82103424074408,
-1.72559036509362));
#68089=CARTESIAN_POINT('Ctrl Pts',(-0.473308921554199,0.732284012198431,
-1.70440823376776));
#68090=CARTESIAN_POINT('Ctrl Pts',(-0.924731019481197,0.142163200013653,
-1.67793056961044));
#68091=CARTESIAN_POINT('Ctrl Pts',(-0.618776106988036,-0.702678676696827,
-1.64615737262165));
#68092=CARTESIAN_POINT('Ctrl Pts',(0.10798043597624,-0.865202037522717,
-1.61967970846433));
#68093=CARTESIAN_POINT('Ctrl Pts',(0.574673663161916,-0.58871002246891,
-1.59849757713847));
#68094=CARTESIAN_POINT('Ctrl Pts',(0.863428554777207,-0.12635519945809,
-1.57731544581262));
#68095=CARTESIAN_POINT('Ctrl Pts',(0.744888341191182,0.454132856952076,
-1.55613331448676));
#68096=CARTESIAN_POINT('Ctrl Pts',(0.297872369146698,0.767766312941754,
-1.5349511831609));
#68097=CARTESIAN_POINT('Ctrl Pts',(-0.105018454779645,0.818579462871879,
-1.5190645846665));
#68098=CARTESIAN_POINT('Ctrl Pts',(-0.482718942225724,0.667214761700076,
-1.50317798617211));
#68099=CARTESIAN_POINT('Ctrl Pts',(-0.83479754287494,0.251742471891821,
-1.48199585484625));
#68100=CARTESIAN_POINT('Ctrl Pts',(-0.796851182620412,-0.490271380548884,
-1.45551819068893));
#68101=CARTESIAN_POINT('Ctrl Pts',(-0.0167447222186907,-0.936141446332493,
-1.42374499370014));
#68102=CARTESIAN_POINT('Ctrl Pts',(0.642392331962497,-0.589547650426033,
-1.39726732954282));
#68103=CARTESIAN_POINT('Ctrl Pts',(0.819113847908267,-0.0766929843740207,
-1.37608519821696));
#68104=CARTESIAN_POINT('Ctrl Pts',(0.739893659542249,0.462635794339282,
-1.3549030668911));
#68105=CARTESIAN_POINT('Ctrl Pts',(0.273763047578798,0.828341165454406,
-1.33372093556524));
#68106=CARTESIAN_POINT('Ctrl Pts',(-0.269979798721475,0.778012832716501,
-1.31253880423939));
#68107=CARTESIAN_POINT('Ctrl Pts',(-0.60995350043272,0.555929797897005,
-1.29665220574499));
#68108=CARTESIAN_POINT('Ctrl Pts',(-0.799847037243918,0.196055687053803,
-1.2807656072506));
#68109=CARTESIAN_POINT('Ctrl Pts',(-0.79924111982244,-0.348532411877579,
-1.25958347592474));
#68110=CARTESIAN_POINT('Ctrl Pts',(-0.289974287295851,-0.889523887557901,
-1.23310581176742));
#68111=CARTESIAN_POINT('Ctrl Pts',(0.593250759993301,-0.724358149696021,
-1.20133261477863));
#68112=CARTESIAN_POINT('Ctrl Pts',(0.87127063585088,-0.0334935723846185,
-1.17485495062131));
#68113=CARTESIAN_POINT('Ctrl Pts',(0.673968441674755,0.471800645732692,
-1.15367281929545));
#68114=CARTESIAN_POINT('Ctrl Pts',(0.264451749975724,0.831588706975706,
-1.13249068796959));
#68115=CARTESIAN_POINT('Ctrl Pts',(-0.327568979751748,0.808575201270978,
-1.11130855664373));
#68116=CARTESIAN_POINT('Ctrl Pts',(-0.709424615516163,0.418222159251501,
-1.09012642531788));
#68117=CARTESIAN_POINT('Ctrl Pts',(-0.824783458077394,0.0288697101095931,
-1.07423982682348));
#68118=CARTESIAN_POINT('Ctrl Pts',(-0.736553190313614,-0.368351073370029,
-1.05835322832909));
#68119=CARTESIAN_POINT('Ctrl Pts',(-0.383550940276186,-0.783038878956529,
-1.03717109700323));
#68120=CARTESIAN_POINT('Ctrl Pts',(0.354819705113078,-0.865702495486934,
-1.0106934328459));
#68121=CARTESIAN_POINT('Ctrl Pts',(0.921085284334245,-0.168056812556349,
-0.978920235857119));
#68122=CARTESIAN_POINT('Ctrl Pts',(0.68575662243418,0.538490663869619,-0.952442571699793));
#68123=CARTESIAN_POINT('Ctrl Pts',(0.208271265596164,0.795897223022045,
-0.931260440373937));
#68124=CARTESIAN_POINT('Ctrl Pts',(-0.336768269145502,0.805022756530337,
-0.910078309048077));
#68125=CARTESIAN_POINT('Ctrl Pts',(-0.773103183752531,0.404236020014726,
-0.888896177722221));
#68126=CARTESIAN_POINT('Ctrl Pts',(-0.811454054952501,-0.140482654767616,
-0.86771404639636));
#68127=CARTESIAN_POINT('Ctrl Pts',(-0.647331254010008,-0.511921342065259,
-0.851827447901969));
#68128=CARTESIAN_POINT('Ctrl Pts',(-0.32294111757287,-0.757563297681273,
-0.835940849407571));
#68129=CARTESIAN_POINT('Ctrl Pts',(0.214563111264144,-0.845117672891099,
-0.814758718081718));
#68130=CARTESIAN_POINT('Ctrl Pts',(0.830854928685622,-0.430137095935519,
-0.78828105392439));
#68131=CARTESIAN_POINT('Ctrl Pts',(0.810834729594931,0.468175431378649,
-0.756507856935606));
#68132=CARTESIAN_POINT('Ctrl Pts',(0.174084163878708,0.854358849777055,
-0.730030192778281));
#68133=CARTESIAN_POINT('Ctrl Pts',(-0.356483549772279,0.741450462537814,
-0.708848061452423));
#68134=CARTESIAN_POINT('Ctrl Pts',(-0.777815113960467,0.395573197022217,
-0.687665930126566));
#68135=CARTESIAN_POINT('Ctrl Pts',(-0.850935313686701,-0.192365237173437,
-0.666483798800706));
#68136=CARTESIAN_POINT('Ctrl Pts',(-0.527541041691738,-0.632371337784837,
-0.64530166747485));
#68137=CARTESIAN_POINT('Ctrl Pts',(-0.16199641567262,-0.809233201559615,
-0.629415068980455));
#68138=CARTESIAN_POINT('Ctrl Pts',(0.244267682003785,-0.786464502814039,
-0.613528470486061));
#68139=CARTESIAN_POINT('Ctrl Pts',(0.710627006659556,-0.505242979937425,
-0.592346339160204));
#68140=CARTESIAN_POINT('Ctrl Pts',(0.911720286535661,0.210009408709779,
-0.565868675002879));
#68141=CARTESIAN_POINT('Ctrl Pts',(0.314936286484835,0.881734837871569,
-0.534095478014093));
#68142=CARTESIAN_POINT('Ctrl Pts',(-0.42038592361789,0.763878279754945,
-0.50761781385677));
#68143=CARTESIAN_POINT('Ctrl Pts',(-0.751688237041493,0.334356236573434,
-0.486435682530911));
#68144=CARTESIAN_POINT('Ctrl Pts',(-0.848918814984445,-0.202018222450293,
-0.465253551205055));
#68145=CARTESIAN_POINT('Ctrl Pts',(-0.524046957129384,-0.697474091242304,
-0.444071419879193));
#68146=CARTESIAN_POINT('Ctrl Pts',(0.00728015342758569,-0.823492551981872,
-0.422889288553338));
#68147=CARTESIAN_POINT('Ctrl Pts',(0.400386949741799,-0.72165898187089,
-0.407002690058941));
#68148=CARTESIAN_POINT('Ctrl Pts',(0.695298182707548,-0.441308572056135,
-0.39111609156455));
#68149=CARTESIAN_POINT('Ctrl Pts',(0.868703867437267,0.0749341801834311,
-0.369933960238689));
#68150=CARTESIAN_POINT('Ctrl Pts',(0.558954270913066,0.750272355031231,
-0.343456296081368));
#68151=CARTESIAN_POINT('Ctrl Pts',(-0.33075083661154,0.875923608760214,
-0.31168309909258));
#68152=CARTESIAN_POINT('Ctrl Pts',(-0.814914090257261,0.310085436417102,
-0.285205434935257));
#68153=CARTESIAN_POINT('Ctrl Pts',(-0.789374400507719,-0.23176697493687,
-0.264023303609398));
#68154=CARTESIAN_POINT('Ctrl Pts',(-0.516265749197611,-0.703518292708922,
-0.242841172283541));
#68155=CARTESIAN_POINT('Ctrl Pts',(0.0520971392298091,-0.870867259982498,
-0.221659040957681));
#68156=CARTESIAN_POINT('Ctrl Pts',(0.538627180893952,-0.622926055038332,
-0.200476909631823));
#68157=CARTESIAN_POINT('Ctrl Pts',(0.772363051366356,-0.290891130998112,
-0.184590311137431));
#68158=CARTESIAN_POINT('Ctrl Pts',(0.815588095945512,0.11381593984541,-0.168703712643035));
#68159=CARTESIAN_POINT('Ctrl Pts',(0.613704285802587,0.619311120740718,
-0.147521581317179));
#68160=CARTESIAN_POINT('Ctrl Pts',(-0.0598573691488588,0.934023329961192,
-0.121043917159855));
#68161=CARTESIAN_POINT('Ctrl Pts',(-0.81878299272184,0.452927951066564,
-0.089270720171069));
#68162=CARTESIAN_POINT('Ctrl Pts',(-0.82243198967408,-0.290216640336301,
-0.0627930560137438));
#68163=CARTESIAN_POINT('Ctrl Pts',(-0.450841104190585,-0.688967090169176,
-0.0416109246878877));
#68164=CARTESIAN_POINT('Ctrl Pts',(-0.0678909476341013,-0.822331958162865,
-0.0257243261934915));
#68165=CARTESIAN_POINT('Ctrl Pts',(0.335042445358195,-0.753606364065075,
-0.00983772769910037));
#68166=CARTESIAN_POINT('Ctrl Pts',(0.547784979994835,-0.585740710520373,
0.000753337963830978));
#68167=CARTESIAN_POINT('Ctrl Pts',(0.627854069260493,-0.481288351939915,
0.00604887079529526));
#68168=CARTESIAN_POINT('Ctrl Pts',(-0.789664670674245,0.000390155355157968,
-0.0731331508236992));
#68169=CARTESIAN_POINT('Ctrl Pts',(-0.789545021916376,-0.108669478777935,
-0.0687554338824675));
#68170=CARTESIAN_POINT('Ctrl Pts',(-0.76801952939625,-0.217821296353336,
-0.0643777169412358));
#68171=CARTESIAN_POINT('Ctrl Pts',(-0.725153241366725,-0.317623382068616,
-0.0600000000000044));
#68172=CARTESIAN_POINT('',(-0.392888236737431,-0.550964357679653,-11.9089));
#68173=CARTESIAN_POINT('Ctrl Pts',(-0.393304595585779,-0.5512599337297,
-11.9089));
#68174=CARTESIAN_POINT('Ctrl Pts',(-0.408693527352117,-0.542220167284383,
-11.9089));
#68175=CARTESIAN_POINT('Ctrl Pts',(-0.423683838010449,-0.532561211544802,
-11.9089));
#68176=CARTESIAN_POINT('Ctrl Pts',(-0.438233215603795,-0.522291678473845,
-11.9089));
#68177=CARTESIAN_POINT('Ctrl Pts',(-0.461867821271025,-0.505609427775394,
-11.9089));
#68178=CARTESIAN_POINT('Ctrl Pts',(-0.48433990880594,-0.487317637060884,
-11.9089));
#68179=CARTESIAN_POINT('Ctrl Pts',(-0.50557477026688,-0.467604008788871,
-11.9089));
#68180=CARTESIAN_POINT('Ctrl Pts',(-0.513462092846287,-0.460281722006926,
-11.9089));
#68181=CARTESIAN_POINT('Ctrl Pts',(-0.521178574541802,-0.45276297817765,
-11.9089));
#68182=CARTESIAN_POINT('Ctrl Pts',(-0.528719788537152,-0.445056426895789,
-11.9089));
#68183=CARTESIAN_POINT('Ctrl Pts',(-0.534715058150292,-0.438929714041502,
-11.9089));
#68184=CARTESIAN_POINT('Ctrl Pts',(-0.54059879777543,-0.432684821204094,
-11.9089));
#68185=CARTESIAN_POINT('Ctrl Pts',(-0.546360102250889,-0.426336159151428,
-11.9089));
#68186=CARTESIAN_POINT('Ctrl Pts',(-0.569122064476836,-0.401253644168294,
-11.9089));
#68187=CARTESIAN_POINT('Ctrl Pts',(-0.59001352525143,-0.374516741518621,
-11.9089));
#68188=CARTESIAN_POINT('Ctrl Pts',(-0.608914082959629,-0.346409536900853,
-11.9089));
#68189=CARTESIAN_POINT('Ctrl Pts',(-0.620816625689087,-0.328709148947567,
-11.9089));
#68190=CARTESIAN_POINT('Ctrl Pts',(-0.631929073242191,-0.310464307003422,
-11.9089));
#68191=CARTESIAN_POINT('Ctrl Pts',(-0.642213965653337,-0.291738016113175,
-11.9089));
#68192=CARTESIAN_POINT('Ctrl Pts',(-0.645959537905604,-0.284918238837686,
-11.9089));
#68193=CARTESIAN_POINT('Ctrl Pts',(-0.649590737078314,-0.278042814352498,
-11.9089));
#68194=CARTESIAN_POINT('Ctrl Pts',(-0.653105696058218,-0.271116451571719,
-11.9089));
#68195=CARTESIAN_POINT('Ctrl Pts',(-0.655265359288032,-0.266860751548043,
-11.9089));
#68196=CARTESIAN_POINT('Ctrl Pts',(-0.657381222064642,-0.262585667889145,
-11.9089));
#68197=CARTESIAN_POINT('Ctrl Pts',(-0.659452991369261,-0.258291988249454,
-11.9089));
#68198=CARTESIAN_POINT('Ctrl Pts',(-0.674373045108698,-0.227370625131801,
-11.9089));
#68199=CARTESIAN_POINT('Ctrl Pts',(-0.687009656395958,-0.195487698886124,
-11.9089));
#68200=CARTESIAN_POINT('Ctrl Pts',(-0.697343938616677,-0.16289685564625,
-11.9089));
#68201=CARTESIAN_POINT('Ctrl Pts',(-0.707706518654146,-0.130216770629341,
-11.9089));
#68202=CARTESIAN_POINT('Ctrl Pts',(-0.715754605809521,-0.096823788691555,
-11.9089));
#68203=CARTESIAN_POINT('Ctrl Pts',(-0.721423679591164,-0.0629478567023877,
-11.9089));
#68204=CARTESIAN_POINT('Ctrl Pts',(-0.723047928495838,-0.0532420480381235,
-11.9089));
#68205=CARTESIAN_POINT('Ctrl Pts',(-0.724476578999849,-0.0434964909242276,
-11.9089));
#68206=CARTESIAN_POINT('Ctrl Pts',(-0.725707343184254,-0.033716403000824,
-11.9089));
#68207=CARTESIAN_POINT('Ctrl Pts',(-0.7265959059525,-0.026655568676088,
-11.9089));
#68208=CARTESIAN_POINT('Ctrl Pts',(-0.727381016204586,-0.0195781656773132,
-11.9089));
#68209=CARTESIAN_POINT('Ctrl Pts',(-0.728061009551409,-0.012498405674025,
-11.9089));
#68210=CARTESIAN_POINT('Ctrl Pts',(-0.731399290066069,0.0222581474273844,
-11.9089));
#68211=CARTESIAN_POINT('Ctrl Pts',(-0.732218291976249,0.05714868313061,
-11.9089));
#68212=CARTESIAN_POINT('Ctrl Pts',(-0.730480688047011,0.0919286611337855,
-11.9089));
#68213=CARTESIAN_POINT('Ctrl Pts',(-0.728924956179102,0.123068277725504,
-11.9089));
#68214=CARTESIAN_POINT('Ctrl Pts',(-0.725319517222503,0.15412018856309,
-11.9089));
#68215=CARTESIAN_POINT('Ctrl Pts',(-0.719751379176906,0.184897223577564,
-11.9089));
#68216=CARTESIAN_POINT('Ctrl Pts',(-0.716657727201263,0.201996913706878,
-11.9089));
#68217=CARTESIAN_POINT('Ctrl Pts',(-0.712957590969093,0.219011827659849,
-11.9089));
#68218=CARTESIAN_POINT('Ctrl Pts',(-0.708661430842914,0.235909638790339,
-11.9089));
#68219=CARTESIAN_POINT('Ctrl Pts',(-0.706772031377583,0.24334109254847,
-11.9089));
#68220=CARTESIAN_POINT('Ctrl Pts',(-0.704766683530507,0.250752063241591,
-11.9089));
#68221=CARTESIAN_POINT('Ctrl Pts',(-0.702648111992644,0.258132763274611,
-11.9089));
#68222=CARTESIAN_POINT('Ctrl Pts',(-0.692735592491751,0.292666094672686,
-11.9089));
#68223=CARTESIAN_POINT('Ctrl Pts',(-0.680390309661971,0.326397320788224,
-11.9089));
#68224=CARTESIAN_POINT('Ctrl Pts',(-0.665760390044392,0.359055268523425,
-11.9089));
#68225=CARTESIAN_POINT('Ctrl Pts',(-0.65223697684172,0.38924319389273,-11.9089));
#68226=CARTESIAN_POINT('Ctrl Pts',(-0.636760651354079,0.418514986268856,
-11.9089));
#68227=CARTESIAN_POINT('Ctrl Pts',(-0.619409069747327,0.446652163200523,
-11.9089));
#68228=CARTESIAN_POINT('Ctrl Pts',(-0.610436195617874,0.461202499457351,
-11.9089));
#68229=CARTESIAN_POINT('Ctrl Pts',(-0.600961251859437,0.475449264180526,
-11.9089));
#68230=CARTESIAN_POINT('Ctrl Pts',(-0.591004529339638,0.489375201004093,
-11.9089));
#68231=CARTESIAN_POINT('Ctrl Pts',(-0.585705005712024,0.496787362092886,
-11.9089));
#68232=CARTESIAN_POINT('Ctrl Pts',(-0.580268955949018,0.504108610136061,
-11.9089));
#68233=CARTESIAN_POINT('Ctrl Pts',(-0.574699182670622,0.511336161684331,
-11.9089));
#68234=CARTESIAN_POINT('Ctrl Pts',(-0.570153054722175,0.51723539176967,
-11.9089));
#68235=CARTESIAN_POINT('Ctrl Pts',(-0.565517950353427,0.523071829695112,
-11.9089));
#68236=CARTESIAN_POINT('Ctrl Pts',(-0.560804459523544,0.528833397455703,
-11.9089));
#68237=CARTESIAN_POINT('Ctrl Pts',(-0.537795487450174,0.556958571872463,
-11.9089));
#68238=CARTESIAN_POINT('Ctrl Pts',(-0.512871815585796,0.583368342494326,
-11.9089));
#68239=CARTESIAN_POINT('Ctrl Pts',(-0.486264283896923,0.607923354592398,
-11.9089));
#68240=CARTESIAN_POINT('Ctrl Pts',(-0.459447509931059,0.632671467903429,
-11.9089));
#68241=CARTESIAN_POINT('Ctrl Pts',(-0.430919545923936,0.655536450034859,
-11.9089));
#68242=CARTESIAN_POINT('Ctrl Pts',(-0.40087273304815,0.676347523766625,
-11.9089));
#68243=CARTESIAN_POINT('Ctrl Pts',(-0.381865830138765,0.689512116613626,
-11.9089));
#68244=CARTESIAN_POINT('Ctrl Pts',(-0.362250311091213,0.701854228634629,
-11.9089));
#68245=CARTESIAN_POINT('Ctrl Pts',(-0.342067962509662,0.713322310757549,
-11.9089));
#68246=CARTESIAN_POINT('Ctrl Pts',(-0.39330459558578,-0.5512599337297,-11.9089));
#68247=CARTESIAN_POINT('Ctrl Pts',(-0.223877593268971,-0.670321260978493,
-11.8991430932763));
#68248=CARTESIAN_POINT('Ctrl Pts',(0.249389096047715,-0.750562929726869,
-11.8787951208897));
#68249=CARTESIAN_POINT('Ctrl Pts',(0.77140418662287,-0.214212144206197,
-11.8478560828401));
#68250=CARTESIAN_POINT('Ctrl Pts',(0.626282581243407,0.404955323743999,
-11.8213784186828));
#68251=CARTESIAN_POINT('Ctrl Pts',(0.238575376523109,0.662775532235479,
-11.800196287357));
#68252=CARTESIAN_POINT('Ctrl Pts',(-0.1078208916813,0.6976941672648,-11.7843096888626));
#68253=CARTESIAN_POINT('Ctrl Pts',(-0.426851047433615,0.560357959801784,
-11.7684230903682));
#68254=CARTESIAN_POINT('Ctrl Pts',(-0.634958032955366,0.302047970066774,
-11.7533805346203));
#68255=CARTESIAN_POINT('Ctrl Pts',(-0.675710582128752,0.0947324392347568,
-11.7436335117039));
#68256=CARTESIAN_POINT('Ctrl Pts',(-0.675354504231418,1.55800137812273E-5,
-11.739182021619));
#68257=CARTESIAN_POINT('Origin',(-1.87869726832665E-16,-4.25270154953079E-17,
-11.9089));
#68258=CARTESIAN_POINT('',(-0.7911,-9.68818082805471E-17,-11.9089));
#68259=CARTESIAN_POINT('Origin',(0.,0.,-11.9089));
#68260=CARTESIAN_POINT('Origin',(0.,0.,-11.9089));
#68261=CARTESIAN_POINT('',(0.392888236737201,-0.550964357679817,-11.9089));
#68262=CARTESIAN_POINT('Ctrl Pts',(0.342488254090117,0.713746195864945,
-11.9089));
#68263=CARTESIAN_POINT('Ctrl Pts',(0.360556518434521,0.703639038104608,
-11.9089));
#68264=CARTESIAN_POINT('Ctrl Pts',(0.378182479561092,0.69280655077716,-11.9089));
#68265=CARTESIAN_POINT('Ctrl Pts',(0.395317146119975,0.681247267951702,
-11.9089));
#68266=CARTESIAN_POINT('Ctrl Pts',(0.421982268203321,0.663258608138712,
-11.9089));
#68267=CARTESIAN_POINT('Ctrl Pts',(0.447458851539857,0.643510628499277,
-11.9089));
#68268=CARTESIAN_POINT('Ctrl Pts',(0.471631160417591,0.622177706263673,
-11.9089));
#68269=CARTESIAN_POINT('Ctrl Pts',(0.483299586240594,0.611879905505248,
-11.9089));
#68270=CARTESIAN_POINT('Ctrl Pts',(0.494663745687151,0.60121247873265,-11.9089));
#68271=CARTESIAN_POINT('Ctrl Pts',(0.505708478051413,0.590193655482738,
-11.9089));
#68272=CARTESIAN_POINT('Ctrl Pts',(0.512460894688372,0.583457078897764,
-11.9089));
#68273=CARTESIAN_POINT('Ctrl Pts',(0.519087121920656,0.576595844964218,
-11.9089));
#68274=CARTESIAN_POINT('Ctrl Pts',(0.525582191777545,0.569617027475966,
-11.9089));
#68275=CARTESIAN_POINT('Ctrl Pts',(0.550035144131404,0.543342838700996,
-11.9089));
#68276=CARTESIAN_POINT('Ctrl Pts',(0.572642835681347,0.515393485339714,
-11.9089));
#68277=CARTESIAN_POINT('Ctrl Pts',(0.593235951420603,0.486007583538113,
-11.9089));
#68278=CARTESIAN_POINT('Ctrl Pts',(0.60601075151929,0.467778238062261,-11.9089));
#68279=CARTESIAN_POINT('Ctrl Pts',(0.618009497356723,0.448995505770734,
-11.9089));
#68280=CARTESIAN_POINT('Ctrl Pts',(0.629182717775896,0.429713041967115,
-11.9089));
#68281=CARTESIAN_POINT('Ctrl Pts',(0.633356702732471,0.422509683327209,
-11.9089));
#68282=CARTESIAN_POINT('Ctrl Pts',(0.637411228744753,0.415243679035629,
-11.9089));
#68283=CARTESIAN_POINT('Ctrl Pts',(0.641342116321425,0.407922266341704,
-11.9089));
#68284=CARTESIAN_POINT('Ctrl Pts',(0.643851100174008,0.403249198015819,
-11.9089));
#68285=CARTESIAN_POINT('Ctrl Pts',(0.646310023336052,0.398553019144131,
-11.9089));
#68286=CARTESIAN_POINT('Ctrl Pts',(0.648718392169465,0.393834526004733,
-11.9089));
#68287=CARTESIAN_POINT('Ctrl Pts',(0.664960125725092,0.362013607509625,
-11.9089));
#68288=CARTESIAN_POINT('Ctrl Pts',(0.678906723612393,0.329179154845523,
-11.9089));
#68289=CARTESIAN_POINT('Ctrl Pts',(0.690491164722862,0.295565210178431,
-11.9089));
#68290=CARTESIAN_POINT('Ctrl Pts',(0.701944731490535,0.262331016495882,
-11.9089));
#68291=CARTESIAN_POINT('Ctrl Pts',(0.711089352408651,0.228333711694692,
-11.9089));
#68292=CARTESIAN_POINT('Ctrl Pts',(0.717810313646535,0.193793925220808,
-11.9089));
#68293=CARTESIAN_POINT('Ctrl Pts',(0.720235359810493,0.181331336354761,
-11.9089));
#68294=CARTESIAN_POINT('Ctrl Pts',(0.722344384174073,0.168798150720673,
-11.9089));
#68295=CARTESIAN_POINT('Ctrl Pts',(0.724130318202715,0.156204981080871,
-11.9089));
#68296=CARTESIAN_POINT('Ctrl Pts',(0.72520494202273,0.148627478302282,-11.9089));
#68297=CARTESIAN_POINT('Ctrl Pts',(0.726161427478842,0.141035887537196,
-11.9089));
#68298=CARTESIAN_POINT('Ctrl Pts',(0.72699834563226,0.133438337157604,-11.9089));
#68299=CARTESIAN_POINT('Ctrl Pts',(0.730622843153363,0.100535116687562,
-11.9089));
#68300=CARTESIAN_POINT('Ctrl Pts',(0.732013163304079,0.0674856197810442,
-11.9089));
#68301=CARTESIAN_POINT('Ctrl Pts',(0.731094528381772,0.0344763444030268,
-11.9089));
#68302=CARTESIAN_POINT('Ctrl Pts',(0.730263242421242,0.0046057761035988,
-11.9089));
#68303=CARTESIAN_POINT('Ctrl Pts',(0.727540491121943,-0.0252324683759116,
-11.9089));
#68304=CARTESIAN_POINT('Ctrl Pts',(0.722968144611873,-0.054854753376587,
-11.9089));
#68305=CARTESIAN_POINT('Ctrl Pts',(0.720637288536924,-0.0699553768301293,
-11.9089));
#68306=CARTESIAN_POINT('Ctrl Pts',(0.71782534797267,-0.0849997333504113,
-11.9089));
#68307=CARTESIAN_POINT('Ctrl Pts',(0.714535318964831,-0.0999621540141962,
-11.9089));
#68308=CARTESIAN_POINT('Ctrl Pts',(0.712583835435694,-0.108837126670006,
-11.9089));
#68309=CARTESIAN_POINT('Ctrl Pts',(0.710464115508743,-0.117683251491007,
-11.9089));
#68310=CARTESIAN_POINT('Ctrl Pts',(0.708176520415106,-0.126494959184421,
-11.9089));
#68311=CARTESIAN_POINT('Ctrl Pts',(0.706420038263088,-0.133260845042161,
-11.9089));
#68312=CARTESIAN_POINT('Ctrl Pts',(0.704566928605242,-0.13999735578593,
-11.9089));
#68313=CARTESIAN_POINT('Ctrl Pts',(0.702618311219262,-0.146701346994649,
-11.9089));
#68314=CARTESIAN_POINT('Ctrl Pts',(0.693128653800149,-0.17934940831711,
-11.9089));
#68315=CARTESIAN_POINT('Ctrl Pts',(0.681375773134325,-0.211235078029093,
-11.9089));
#68316=CARTESIAN_POINT('Ctrl Pts',(0.667432282574939,-0.242091271590305,
-11.9089));
#68317=CARTESIAN_POINT('Ctrl Pts',(0.657257815394937,-0.264606819426136,
-11.9089));
#68318=CARTESIAN_POINT('Ctrl Pts',(0.6459158888732,-0.286574025624279,-11.9089));
#68319=CARTESIAN_POINT('Ctrl Pts',(0.633420198244177,-0.307879193780786,
-11.9089));
#68320=CARTESIAN_POINT('Ctrl Pts',(0.625264218444548,-0.321785149543534,
-11.9089));
#68321=CARTESIAN_POINT('Ctrl Pts',(0.616616438077692,-0.335408851785583,
-11.9089));
#68322=CARTESIAN_POINT('Ctrl Pts',(0.607493621761733,-0.34872796535831,
-11.9089));
#68323=CARTESIAN_POINT('Ctrl Pts',(0.60287540554187,-0.355470460680522,
-11.9089));
#68324=CARTESIAN_POINT('Ctrl Pts',(0.598135429986056,-0.362134865865414,
-11.9089));
#68325=CARTESIAN_POINT('Ctrl Pts',(0.593275738783337,-0.368718057791076,
-11.9089));
#68326=CARTESIAN_POINT('Ctrl Pts',(0.589123720455206,-0.374342599020702,
-11.9089));
#68327=CARTESIAN_POINT('Ctrl Pts',(0.584884848339669,-0.379906916848787,
-11.9089));
#68328=CARTESIAN_POINT('Ctrl Pts',(0.580568488351745,-0.385399387785345,
-11.9089));
#68329=CARTESIAN_POINT('Ctrl Pts',(0.559975931714266,-0.411602952631009,
-11.9089));
#68330=CARTESIAN_POINT('Ctrl Pts',(0.537577275146447,-0.436236631350958,
-11.9089));
#68331=CARTESIAN_POINT('Ctrl Pts',(0.513552303528644,-0.459132736511132,
-11.9089));
#68332=CARTESIAN_POINT('Ctrl Pts',(0.489919994544589,-0.48165462916035,
-11.9089));
#68333=CARTESIAN_POINT('Ctrl Pts',(0.46471309828054,-0.502495897953426,
-11.9089));
#68334=CARTESIAN_POINT('Ctrl Pts',(0.438076047439824,-0.521455358176732,
-11.9089));
#68335=CARTESIAN_POINT('Ctrl Pts',(0.423438349467291,-0.531874036060051,
-11.9089));
#68336=CARTESIAN_POINT('Ctrl Pts',(0.408368394069875,-0.541723664274757,
-11.9089));
#68337=CARTESIAN_POINT('Ctrl Pts',(0.392888236737142,-0.550964357679859,
-11.9089));
#68338=CARTESIAN_POINT('Origin',(0.,0.,-11.9089));
#68339=CARTESIAN_POINT('Origin',(0.,0.,-12.278617978381));
#68340=CARTESIAN_POINT('Ctrl Pts',(0.392888236737129,-0.550964357679868,
-11.9089));
#68341=CARTESIAN_POINT('Ctrl Pts',(0.484548909927025,-0.485601871403322,
-11.9036044671685));
#68342=CARTESIAN_POINT('Ctrl Pts',(0.634341446219948,-0.308693578393974,
-11.8930134015056));
#68343=CARTESIAN_POINT('Ctrl Pts',(0.705002038108303,0.0337351900899797,
-11.8771268030112));
#68344=CARTESIAN_POINT('Ctrl Pts',(0.602308840879945,0.365053324407907,
-11.8612402045168));
#68345=CARTESIAN_POINT('Ctrl Pts',(0.272406965382598,0.694503928448386,
-11.840058073191));
#68346=CARTESIAN_POINT('Ctrl Pts',(-0.363000708994007,0.713347601796957,
-11.8135804090336));
#68347=CARTESIAN_POINT('Ctrl Pts',(-0.666650932811795,0.269067688681329,
-11.7913351998198));
#68348=CARTESIAN_POINT('Ctrl Pts',(-0.677875715687106,0.0226766229145017,
-11.779681056269));
#68349=CARTESIAN_POINT('Ctrl Pts',(-0.677716351375759,0.000193615723412331,
-11.778617978381));
#68350=CARTESIAN_POINT('Ctrl Pts',(0.459308237155017,-0.644108029201275,
-11.9749488707953));
#68351=CARTESIAN_POINT('Ctrl Pts',(0.566464670671375,-0.567695641299125,
-11.9696533379638));
#68352=CARTESIAN_POINT('Ctrl Pts',(0.741580490770848,-0.360879990937501,
-11.9590622723009));
#68353=CARTESIAN_POINT('Ctrl Pts',(0.824186659298766,0.0394383166547306,
-11.9431756738065));
#68354=CARTESIAN_POINT('Ctrl Pts',(0.704132590542465,0.426767673916296,
-11.9272890753121));
#68355=CARTESIAN_POINT('Ctrl Pts',(0.318458918744054,0.811913784240501,
-11.9061069439863));
#68356=CARTESIAN_POINT('Ctrl Pts',(-0.424368052143095,0.833943088194967,
-11.8796292798289));
#68357=CARTESIAN_POINT('Ctrl Pts',(-0.931397559300446,0.0920927363171967,
-11.8478560828401));
#68358=CARTESIAN_POINT('Ctrl Pts',(-0.640145236706153,-0.591940276217127,
-11.8213784186828));
#68359=CARTESIAN_POINT('Ctrl Pts',(-0.141927077663759,-0.811168734010836,
-11.800196287357));
#68360=CARTESIAN_POINT('Ctrl Pts',(0.264031815171026,-0.781952385882165,
-11.7843096888626));
#68361=CARTESIAN_POINT('Ctrl Pts',(0.60394422145073,-0.559828087380095,
-11.7684230903682));
#68362=CARTESIAN_POINT('Ctrl Pts',(0.868547317678143,-0.0821550569317134,
-11.7472409590423));
#68363=CARTESIAN_POINT('Ctrl Pts',(0.720935568709495,0.491650503650886,
-11.7260588277165));
#68364=CARTESIAN_POINT('Ctrl Pts',(0.258901989905492,0.780895405589816,
-11.7048766963906));
#68365=CARTESIAN_POINT('Ctrl Pts',(-0.281744494913556,0.82514119516826,
-11.6836945650647));
#68366=CARTESIAN_POINT('Ctrl Pts',(-0.863972983588544,0.360817083758319,
-11.6572169009074));
#68367=CARTESIAN_POINT('Ctrl Pts',(-0.769136632246591,-0.532698155274108,
-11.6254437039186));
#68368=CARTESIAN_POINT('Ctrl Pts',(-0.104903716392486,-0.865596182377949,
-11.5989660397613));
#68369=CARTESIAN_POINT('Ctrl Pts',(0.417022089888044,-0.710130547992447,
-11.5777839084354));
#68370=CARTESIAN_POINT('Ctrl Pts',(0.707394488276981,-0.425081678732232,
-11.5618973099411));
#68371=CARTESIAN_POINT('Ctrl Pts',(0.822749350428807,-0.03572800263825,
-11.5460107114466));
#68372=CARTESIAN_POINT('Ctrl Pts',(0.715163821668032,0.499635896836913,
-11.5248285801208));
#68373=CARTESIAN_POINT('Ctrl Pts',(0.231228296670995,0.841432107454425,
-11.5036464487949));
#68374=CARTESIAN_POINT('Ctrl Pts',(-0.308185297928774,0.762791662764251,
-11.4824643174691));
#68375=CARTESIAN_POINT('Ctrl Pts',(-0.74889760168553,0.446527416008366,
-11.4612821861432));
#68376=CARTESIAN_POINT('Ctrl Pts',(-0.892089647326341,-0.284283749086055,
-11.4348045219859));
#68377=CARTESIAN_POINT('Ctrl Pts',(-0.241384542900942,-0.903919982673135,
-11.4030313249971));
#68378=CARTESIAN_POINT('Ctrl Pts',(0.480388704926853,-0.727659194643114,
-11.3765536608398));
#68379=CARTESIAN_POINT('Ctrl Pts',(0.777555337808534,-0.271294694573063,
-11.3553715295139));
#68380=CARTESIAN_POINT('Ctrl Pts',(0.814347127607299,0.133940169310587,
-11.3394849310195));
#68381=CARTESIAN_POINT('Ctrl Pts',(0.650220660779249,0.505377237137551,
-11.3235983325252));
#68382=CARTESIAN_POINT('Ctrl Pts',(0.221650746048364,0.843780919035312,
-11.3024162011993));
#68383=CARTESIAN_POINT('Ctrl Pts',(-0.368463008335961,0.791018025834893,
-11.2812340698734));
#68384=CARTESIAN_POINT('Ctrl Pts',(-0.728691043035294,0.381888299710684,
-11.2600519385476));
#68385=CARTESIAN_POINT('Ctrl Pts',(-0.859863472935527,-0.144461580418369,
-11.2388698072217));
#68386=CARTESIAN_POINT('Ctrl Pts',(-0.495910766423547,-0.794174857955777,
-11.2123921430644));
#68387=CARTESIAN_POINT('Ctrl Pts',(0.401173711199402,-0.845220377927278,
-11.1806189460756));
#68388=CARTESIAN_POINT('Ctrl Pts',(0.837199800884732,-0.243634363641056,
-11.1541412819183));
#68389=CARTESIAN_POINT('Ctrl Pts',(0.76826881600657,0.29657400723058,-11.1329591505924));
#68390=CARTESIAN_POINT('Ctrl Pts',(0.533981408593767,0.629257553118175,
-11.117072552098));
#68391=CARTESIAN_POINT('Ctrl Pts',(0.168435037412188,0.806115809149882,
-11.1011859536036));
#68392=CARTESIAN_POINT('Ctrl Pts',(-0.377283459386535,0.786608214983151,
-11.0800038222778));
#68393=CARTESIAN_POINT('Ctrl Pts',(-0.792906556675638,0.364381253655753,
-11.0588216909519));
#68394=CARTESIAN_POINT('Ctrl Pts',(-0.802617937082025,-0.18064815737068,
-11.0376395596261));
#68395=CARTESIAN_POINT('Ctrl Pts',(-0.561862488264964,-0.666741992503685,
-11.0164574283002));
#68396=CARTESIAN_POINT('Ctrl Pts',(0.136132386625423,-0.926341819511223,
-10.9899797641429));
#68397=CARTESIAN_POINT('Ctrl Pts',(0.85292637800386,-0.384518435883188,
-10.9582065671541));
#68398=CARTESIAN_POINT('Ctrl Pts',(0.795823295292128,0.356267445067071,
-10.9317289029968));
#68399=CARTESIAN_POINT('Ctrl Pts',(0.393579533887635,0.723386664183689,
-10.9105467716709));
#68400=CARTESIAN_POINT('Ctrl Pts',(-0.000355675929877251,0.825288486757545,
-10.8946601731765));
#68401=CARTESIAN_POINT('Ctrl Pts',(-0.393461383550265,0.72345089622168,
-10.8787735746821));
#68402=CARTESIAN_POINT('Ctrl Pts',(-0.796774721772053,0.355310195957094,
-10.8575914433563));
#68403=CARTESIAN_POINT('Ctrl Pts',(-0.840229183144532,-0.235561935437421,
-10.8364093120304));
#68404=CARTESIAN_POINT('Ctrl Pts',(-0.494804998307184,-0.6572650327969,
-10.8152271807046));
#68405=CARTESIAN_POINT('Ctrl Pts',(0.00337061571255417,-0.871907666692289,
-10.7940450493787));
#68406=CARTESIAN_POINT('Ctrl Pts',(0.703428476217358,-0.617923597308111,
-10.7675673852214));
#68407=CARTESIAN_POINT('Ctrl Pts',(0.899011593465778,0.259067536837369,
-10.7357941882326));
#68408=CARTESIAN_POINT('Ctrl Pts',(0.375938613330605,0.786721913226838,
-10.7093165240752));
#68409=CARTESIAN_POINT('Ctrl Pts',(-0.168303403544914,0.806143336987419,
-10.6881343927494));
#68410=CARTESIAN_POINT('Ctrl Pts',(-0.534523594447955,0.628797057768532,
-10.672247794255));
#68411=CARTESIAN_POINT('Ctrl Pts',(-0.76822034367083,0.296699449206626,
-10.6563611957606));
#68412=CARTESIAN_POINT('Ctrl Pts',(-0.837305291877463,-0.244979878357376,
-10.6351790644348));
#68413=CARTESIAN_POINT('Ctrl Pts',(-0.487923377363477,-0.72346754139835,
-10.6139969331089));
#68414=CARTESIAN_POINT('Ctrl Pts',(0.0483462858974055,-0.821274586436964,
-10.5928148017831));
#68415=CARTESIAN_POINT('Ctrl Pts',(0.567000592948025,-0.662378040007112,
-10.5716326704572));
#68416=CARTESIAN_POINT('Ctrl Pts',(0.93616106243427,-0.015609562633481,
-10.5451550062999));
#68417=CARTESIAN_POINT('Ctrl Pts',(0.517510382654335,0.779436230665358,
-10.5133818093111));
#68418=CARTESIAN_POINT('Ctrl Pts',(-0.222749378110494,0.842996989493808,
-10.4869041451538));
#68419=CARTESIAN_POINT('Ctrl Pts',(-0.650138150971392,0.50548343203859,
-10.4657220138279));
#68420=CARTESIAN_POINT('Ctrl Pts',(-0.814462273688168,0.133238198796839,
-10.4498354153335));
#68421=CARTESIAN_POINT('Ctrl Pts',(-0.777599598203426,-0.271167705420671,
-10.4339488168391));
#68422=CARTESIAN_POINT('Ctrl Pts',(-0.479598086123451,-0.728753022904691,
-10.4127666855133));
#68423=CARTESIAN_POINT('Ctrl Pts',(0.0964477485296225,-0.867278696520513,
-10.3915845541874));
#68424=CARTESIAN_POINT('Ctrl Pts',(0.568503188538161,-0.594670862165976,
-10.3704024228615));
#68425=CARTESIAN_POINT('Ctrl Pts',(0.860954673904028,-0.137809251394405,
-10.3492202915357));
#68426=CARTESIAN_POINT('Ctrl Pts',(0.723638252600749,0.594128666735248,
-10.3227426273783));
#68427=CARTESIAN_POINT('Ctrl Pts',(-0.110128271419062,0.929090737045152,
-10.2909694303896));
#68428=CARTESIAN_POINT('Ctrl Pts',(-0.715493674016255,0.498327213973867,
-10.2644917662322));
#68429=CARTESIAN_POINT('Ctrl Pts',(-0.82275525250952,-0.0355936775566611,
-10.2433096349064));
#68430=CARTESIAN_POINT('Ctrl Pts',(-0.707027736084488,-0.425691194749398,
-10.227423036412));
#68431=CARTESIAN_POINT('Ctrl Pts',(-0.417138201420715,-0.710062518729677,
-10.2115364379176));
#68432=CARTESIAN_POINT('Ctrl Pts',(0.106214778315677,-0.865917844528771,
-10.1903543065917));
#68433=CARTESIAN_POINT('Ctrl Pts',(0.634946553736723,-0.598596174004323,
-10.1691721752659));
#68434=CARTESIAN_POINT('Ctrl Pts',(0.818269532838146,-0.0852307533471595,
-10.14799004394));
#68435=CARTESIAN_POINT('Ctrl Pts',(0.74542289853333,0.452304148366167,-10.1268079126142));
#68436=CARTESIAN_POINT('Ctrl Pts',(0.166939798545099,0.921288389661671,
-10.1003302484568));
#68437=CARTESIAN_POINT('Ctrl Pts',(-0.685387896845896,0.636852623992408,
-10.0685570514681));
#68438=CARTESIAN_POINT('Ctrl Pts',(-0.86793603686864,-0.0833561374404725,
-10.0420793873107));
#68439=CARTESIAN_POINT('Ctrl Pts',(-0.604054844156638,-0.559741780346003,
-10.0208972559849));
#68440=CARTESIAN_POINT('Ctrl Pts',(-0.263317821004248,-0.78215403727239,
-10.0050106574905));
#68441=CARTESIAN_POINT('Ctrl Pts',(0.141721785662681,-0.811238556195293,
-9.98912405899608));
#68442=CARTESIAN_POINT('Ctrl Pts',(0.641509943308538,-0.591236234716949,
-9.96794192767022));
#68443=CARTESIAN_POINT('Ctrl Pts',(0.871453115729,-0.0452103165325772,-9.94675979634435));
#68444=CARTESIAN_POINT('Ctrl Pts',(0.678851857913411,0.464746667222898,
-9.92557766501851));
#68445=CARTESIAN_POINT('Ctrl Pts',(0.275354301209706,0.827293387555099,
-9.90439553369265));
#68446=CARTESIAN_POINT('Ctrl Pts',(-0.469158289932969,0.810266432879237,
-9.87791786953531));
#68447=CARTESIAN_POINT('Ctrl Pts',(-0.934664449803593,0.0417157057018528,
-9.84614467254655));
#68448=CARTESIAN_POINT('Ctrl Pts',(-0.607572078939521,-0.625393778860442,
-9.8196670083892));
#68449=CARTESIAN_POINT('Ctrl Pts',(-0.0980548570626957,-0.817666411454223,
-9.79848487706337));
#68450=CARTESIAN_POINT('Ctrl Pts',(0.305630886184607,-0.766610053606093,
-9.78259827856895));
#68451=CARTESIAN_POINT('Ctrl Pts',(0.6331762884375,-0.526574636067626,-9.76671168007458));
#68452=CARTESIAN_POINT('Ctrl Pts',(0.871691196454429,-0.0353518122569055,
-9.7455295487487));
#68453=CARTESIAN_POINT('Ctrl Pts',(0.69348056963452,0.52967839787378,-9.72434741742285));
#68454=CARTESIAN_POINT('Ctrl Pts',(0.216559770685256,0.793682036717495,
-9.703165286097));
#68455=CARTESIAN_POINT('Ctrl Pts',(-0.325677859285955,0.808806696472022,
-9.68198315477113));
#68456=CARTESIAN_POINT('Ctrl Pts',(-0.882116078545032,0.313866878207942,
-9.65550549061384));
#68457=CARTESIAN_POINT('Ctrl Pts',(-0.73939742316676,-0.573261968425616,
-9.62373229362499));
#68458=CARTESIAN_POINT('Ctrl Pts',(-0.0582356808045011,-0.869982652255475,
-9.59725462946773));
#68459=CARTESIAN_POINT('Ctrl Pts',(0.45458182105381,-0.686693878945643,
-9.57607249814183));
#68460=CARTESIAN_POINT('Ctrl Pts',(0.729215930288042,-0.386452247883321,
-9.56018589964745));
#68461=CARTESIAN_POINT('Ctrl Pts',(0.823480518688803,0.00853785273125205,
-9.54429930115305));
#68462=CARTESIAN_POINT('Ctrl Pts',(0.687280105947665,0.537346581430056,
-9.52311716982721));
#68463=CARTESIAN_POINT('Ctrl Pts',(0.185675927252062,0.852642337486147,
-9.50193503850133));
#68464=CARTESIAN_POINT('Ctrl Pts',(-0.348732121100362,0.745127651748426,
-9.48075290717549));
#68465=CARTESIAN_POINT('Ctrl Pts',(-0.771811648080317,0.405636684946787,
-9.45957077584961));
#68466=CARTESIAN_POINT('Ctrl Pts',(-0.875523258105161,-0.331813528628048,
-9.43309311169231));
#68467=CARTESIAN_POINT('Ctrl Pts',(-0.19245940133309,-0.915585721091894,
-9.4013199147035));
#68468=CARTESIAN_POINT('Ctrl Pts',(0.518798676753727,-0.700791797000234,
-9.37484225054619));
#68469=CARTESIAN_POINT('Ctrl Pts',(0.791011035633738,-0.229117124893915,
-9.35366011922032));
#68470=CARTESIAN_POINT('Ctrl Pts',(0.805972484214374,0.177509345019459,
-9.33777352072595));
#68471=CARTESIAN_POINT('Ctrl Pts',(0.622122289133055,0.539589581953811,
-9.32188692223153));
#68472=CARTESIAN_POINT('Ctrl Pts',(0.175985973568179,0.85447307137982,-9.3007047909057));
#68473=CARTESIAN_POINT('Ctrl Pts',(-0.410439596498066,0.770073920647401,
-9.27952265957981));
#68474=CARTESIAN_POINT('Ctrl Pts',(-0.74816061082109,0.342176869620224,
-9.25834052825398));
#68475=CARTESIAN_POINT('Ctrl Pts',(-0.850857640946981,-0.190461584392268,
-9.2371583969281));
#68476=CARTESIAN_POINT('Ctrl Pts',(-0.452515495106881,-0.81967732672793,
-9.2106807327708));
#68477=CARTESIAN_POINT('Ctrl Pts',(0.446015846735313,-0.82244008796376,
-9.17890753578198));
#68478=CARTESIAN_POINT('Ctrl Pts',(0.849082854713835,-0.198291491434303,
-9.1524298716247));
#68479=CARTESIAN_POINT('Ctrl Pts',(0.751220872924518,0.337431942021702,
-9.13124774029881));
#68480=CARTESIAN_POINT('Ctrl Pts',(0.499393721105105,0.657044233062526,
-9.11536114180443));
#68481=CARTESIAN_POINT('Ctrl Pts',(0.124871272155171,0.814002595192172,
-9.09947454331003));
#68482=CARTESIAN_POINT('Ctrl Pts',(-0.419010320228561,0.765196474212969,
-9.07829241198418));
#68483=CARTESIAN_POINT('Ctrl Pts',(-0.811342509484049,0.321244202965407,
-9.05711028065831));
#68484=CARTESIAN_POINT('Ctrl Pts',(-0.791750172340431,-0.223519516566628,
-9.03592814933246));
#68485=CARTESIAN_POINT('Ctrl Pts',(-0.525220111816607,-0.695972825928158,
-9.01474601800659));
#68486=CARTESIAN_POINT('Ctrl Pts',(0.185716948854799,-0.917687532971727,
-8.98826835384928));
#68487=CARTESIAN_POINT('Ctrl Pts',(0.872357765986865,-0.338126842991299,
-8.95649515686048));
#68488=CARTESIAN_POINT('Ctrl Pts',(0.77552763160743,0.398519889538282,-8.93001749270316));
#68489=CARTESIAN_POINT('Ctrl Pts',(0.354136265148752,0.743492179596064,
-8.90883536137731));
#68490=CARTESIAN_POINT('Ctrl Pts',(-0.0447058682790427,0.824076815728572,
-8.89294876288291));
#68491=CARTESIAN_POINT('Ctrl Pts',(-0.431770815408578,0.701261023122384,
-8.87706216438852));
#68492=CARTESIAN_POINT('Ctrl Pts',(-0.814717609633828,0.311978379312639,
-8.85588003306266));
#68493=CARTESIAN_POINT('Ctrl Pts',(-0.826356022783278,-0.280375158037511,
-8.8346979017368));
#68494=CARTESIAN_POINT('Ctrl Pts',(-0.458768809576972,-0.682905915223033,
-8.81351577041095));
#68495=CARTESIAN_POINT('Ctrl Pts',(0.050221749372257,-0.870466608306755,
-8.79233363908508));
#68496=CARTESIAN_POINT('Ctrl Pts',(0.735619000821108,-0.579228693086441,
-8.76585597492777));
#68497=CARTESIAN_POINT('Ctrl Pts',(0.883790308873034,0.307005738987016,
-8.73408277793897));
#68498=CARTESIAN_POINT('Ctrl Pts',(0.33311722255521,0.805787891309704,-8.70760511378166));
#68499=CARTESIAN_POINT('Ctrl Pts',(-0.211382054860909,0.795933880606166,
-8.6864229824558));
#68500=CARTESIAN_POINT('Ctrl Pts',(-0.567542525583312,0.599163328763069,
-8.6705363839614));
#68501=CARTESIAN_POINT('Ctrl Pts',(-0.783054772697314,0.254986828179804,
-8.65464978546701));
#68502=CARTESIAN_POINT('Ctrl Pts',(-0.822930239729612,-0.28962236299112,
-8.63346765414114));
#68503=CARTESIAN_POINT('Ctrl Pts',(-0.448339433712863,-0.748642944141454,
-8.6122855228153));
#68504=CARTESIAN_POINT('Ctrl Pts',(0.09241142536838,-0.817489717457452,
-8.59110339148942));
#68505=CARTESIAN_POINT('Ctrl Pts',(0.601777224121419,-0.630950483648119,
-8.56992126016359));
#68506=CARTESIAN_POINT('Ctrl Pts',(0.935647144657611,0.0347219521013799,
-8.54344359600624));
#68507=CARTESIAN_POINT('Ctrl Pts',(0.474875948012168,0.806120752634742,
-8.51167039901748));
#68508=CARTESIAN_POINT('Ctrl Pts',(-0.267729856010204,0.829808371821463,
-8.48519273486012));
#68509=CARTESIAN_POINT('Ctrl Pts',(-0.676363187059825,0.469814808838856,
-8.4640106035343));
#68510=CARTESIAN_POINT('Ctrl Pts',(-0.820445533492922,0.0892767576216661,
-8.44812400503988));
#68511=CARTESIAN_POINT('Ctrl Pts',(-0.7619034974846,-0.312563785666185,
-8.4322374065455));
#68512=CARTESIAN_POINT('Ctrl Pts',(-0.439742132798475,-0.753473389873756,
-8.41105527521964));
#68513=CARTESIAN_POINT('Ctrl Pts',(0.142915624818966,-0.860842395457705,
-8.38987314389378));
#68514=CARTESIAN_POINT('Ctrl Pts',(0.599639089059623,-0.563260394985328,
-8.36869101256792));
#68515=CARTESIAN_POINT('Ctrl Pts',(0.867116398052039,-0.0913427201058315,
-8.34750888124207));
#68516=CARTESIAN_POINT('Ctrl Pts',(0.690664321177558,0.632158199121087,
-8.32103121708474));
#68517=CARTESIAN_POINT('Ctrl Pts',(-0.159898135915144,0.921829930062871,
-8.28925802009595));
#68518=CARTESIAN_POINT('Ctrl Pts',(-0.741239697580997,0.459156749350661,
-8.26278035593863));
#68519=CARTESIAN_POINT('Ctrl Pts',(-0.819653564523485,-0.0797568152445793,
-8.24159822461276));
#68520=CARTESIAN_POINT('Ctrl Pts',(-0.683129576299145,-0.46307147921814,
-8.22571162611839));
#68521=CARTESIAN_POINT('Ctrl Pts',(-0.37837692475353,-0.731453322094652,
-8.20982502762398));
#68522=CARTESIAN_POINT('Ctrl Pts',(0.152595409369933,-0.858958633256121,
-8.18864289629813));
#68523=CARTESIAN_POINT('Ctrl Pts',(0.666197387211884,-0.563609392138577,
-8.16746076497226));
#68524=CARTESIAN_POINT('Ctrl Pts',(0.82166738823947,-0.0411340830821482,
-8.14627863364641));
#68525=CARTESIAN_POINT('Ctrl Pts',(0.720039086476889,0.49170931883848,-8.12509650232054));
#68526=CARTESIAN_POINT('Ctrl Pts',(0.117188860902527,0.928928395595722,
-8.09861883816323));
#68527=CARTESIAN_POINT('Ctrl Pts',(-0.718621729503222,0.599099861220695,
-8.06684564117445));
#68528=CARTESIAN_POINT('Ctrl Pts',(-0.862202324405923,-0.129878256583835,
-8.04036797701711));
#68529=CARTESIAN_POINT('Ctrl Pts',(-0.573101651871943,-0.59139463307986,
-8.01918584569127));
#68530=CARTESIAN_POINT('Ctrl Pts',(-0.220904645367528,-0.795174415166241,
-8.00329924719686));
#68531=CARTESIAN_POINT('Ctrl Pts',(0.185112663155078,-0.802450223707911,
-7.98741264870248));
#68532=CARTESIAN_POINT('Ctrl Pts',(0.672355772075423,-0.555907373905817,
-7.9662305173766));
#68533=CARTESIAN_POINT('Ctrl Pts',(0.872623435995562,0.00168659006782953,
-7.94504838605077));
#68534=CARTESIAN_POINT('Ctrl Pts',(0.652895585756275,0.500556354257191,
-7.92386625472488));
#68535=CARTESIAN_POINT('Ctrl Pts',(0.230497960195097,0.840895374367688,
-7.90268412339905));
#68536=CARTESIAN_POINT('Ctrl Pts',(-0.512023774061414,0.783883185212936,
-7.87620645924171));
#68537=CARTESIAN_POINT('Ctrl Pts',(-0.935555629394363,-0.0085731054685198,
-7.84443326225293));
#68538=CARTESIAN_POINT('Ctrl Pts',(-0.573085689409466,-0.657140778173378,
-7.8179555980956));
#68539=CARTESIAN_POINT('Ctrl Pts',(-0.0539720672566957,-0.821754301096167,
-7.79677346676974));
#68540=CARTESIAN_POINT('Ctrl Pts',(0.346386592324105,-0.749077794049471,
-7.78088686827535));
#68541=CARTESIAN_POINT('Ctrl Pts',(0.660559268446202,-0.491787060076878,
-7.76500026978096));
#68542=CARTESIAN_POINT('Ctrl Pts',(0.872331380217636,0.0115436429949378,
-7.74381813845509));
#68543=CARTESIAN_POINT('Ctrl Pts',(0.664013750878078,0.56618039905986,-7.72263600712925));
#68544=CARTESIAN_POINT('Ctrl Pts',(0.173594650754386,0.804172995640082,
-7.70145387580338));
#68545=CARTESIAN_POINT('Ctrl Pts',(-0.36867222958205,0.790136144864968,
-7.68027174447752));
#68546=CARTESIAN_POINT('Ctrl Pts',(-0.897708497584408,0.266008734120548,
-7.65379408032021));
#68547=CARTESIAN_POINT('Ctrl Pts',(-0.70752208830902,-0.612168545732056,
-7.62202088333141));
#68548=CARTESIAN_POINT('Ctrl Pts',(-0.0113989744896448,-0.871855075757903,
-7.59554321917409));
#68549=CARTESIAN_POINT('Ctrl Pts',(0.490827623867311,-0.661272530098432,
-7.57436108784823));
#68550=CARTESIAN_POINT('Ctrl Pts',(0.748930004517856,-0.346706015541711,
-7.55847448935384));
#68551=CARTESIAN_POINT('Ctrl Pts',(0.821831752970098,0.052779062130137,
-7.54258789085944));
#68552=CARTESIAN_POINT('Ctrl Pts',(0.657410161550947,0.573504291261676,
-7.52140575953358));
#68553=CARTESIAN_POINT('Ctrl Pts',(0.13958692969923,0.861388411050381,-7.50022362820774));
#68554=CARTESIAN_POINT('Ctrl Pts',(-0.388271088612359,0.725310189805061,
-7.47904149688187));
#68555=CARTESIAN_POINT('Ctrl Pts',(-0.79249513545432,0.363573652192116,
-7.45785936555601));
#68556=CARTESIAN_POINT('Ctrl Pts',(-0.856426571169585,-0.378384356783391,
-7.43138170139869));
#68557=CARTESIAN_POINT('Ctrl Pts',(-0.142978046749217,-0.924605381758418,
-7.39960850440991));
#68558=CARTESIAN_POINT('Ctrl Pts',(0.55570930206589,-0.671899085683014,
-7.37313084025257));
#68559=CARTESIAN_POINT('Ctrl Pts',(0.802180681898857,-0.186277397990996,
-7.35194870892673));
#68560=CARTESIAN_POINT('Ctrl Pts',(0.795268550736357,0.220565512013144,
-7.33606211043232));
#68561=CARTESIAN_POINT('Ctrl Pts',(0.592225960946144,0.572242492978857,
-7.32017551193793));
#68562=CARTESIAN_POINT('Ctrl Pts',(0.129812595197046,0.862695764875549,
-7.29899338061208));
#68563=CARTESIAN_POINT('Ctrl Pts',(-0.4512299990804,0.74690427336082,-7.27781124928622));
#68564=CARTESIAN_POINT('Ctrl Pts',(-0.765467966741164,0.301476535704575,
-7.25662911796036));
#68565=CARTESIAN_POINT('Ctrl Pts',(-0.839392798903865,-0.235911147331808,
-7.2354469866345));
#68566=CARTESIAN_POINT('Ctrl Pts',(-0.40781243725763,-0.84281089769987,
-7.20896932247717));
#68567=CARTESIAN_POINT('Ctrl Pts',(0.489568979966038,-0.797282915710522,
-7.17719612548839));
#68568=CARTESIAN_POINT('Ctrl Pts',(0.858512027676108,-0.152375549481188,
-7.15071846133107));
#68569=CARTESIAN_POINT('Ctrl Pts',(0.732001873721275,0.377314686014943,
-7.1295363300052));
#68570=CARTESIAN_POINT('Ctrl Pts',(0.463362767283833,0.682932030860315,
-7.11364973151082));
#68571=CARTESIAN_POINT('Ctrl Pts',(0.0809466243007569,0.819536883613883,
-7.09776313301642));
#68572=CARTESIAN_POINT('Ctrl Pts',(-0.459526225740245,0.741573287317527,
-7.07658100169057));
#68573=CARTESIAN_POINT('Ctrl Pts',(-0.827433652417946,0.277178744641522,
-7.05539887036469));
#68574=CARTESIAN_POINT('Ctrl Pts',(-0.778594220303515,-0.265744896088806,
-7.03421673903885));
#68575=CARTESIAN_POINT('Ctrl Pts',(-0.487059829810343,-0.723192272132506,
-7.01303460771298));
#68576=CARTESIAN_POINT('Ctrl Pts',(0.234764782229873,-0.906381095504675,
-6.98655694355566));
#68577=CARTESIAN_POINT('Ctrl Pts',(0.88926800774623,-0.290758051011389,
-6.95478374656688));
#68578=CARTESIAN_POINT('Ctrl Pts',(0.752990664370407,0.439620596782193,
-6.92830608240955));
#68579=CARTESIAN_POINT('Ctrl Pts',(0.313669529499514,0.761448975097948,
-6.9071239510837));
#68580=CARTESIAN_POINT('Ctrl Pts',(-0.0889268590147663,0.820483532208579,
-6.89123735258931));
#68581=CARTESIAN_POINT('Ctrl Pts',(-0.468832413633215,0.677044479717714,
-6.8753507540949));
#68582=CARTESIAN_POINT('Ctrl Pts',(-0.830305933457297,0.267744933607144,
-6.85416862276906));
#68583=CARTESIAN_POINT('Ctrl Pts',(-0.810094662937232,-0.324378086054845,
-6.83298649144319));
#68584=CARTESIAN_POINT('Ctrl Pts',(-0.421406762012617,-0.706573174286,-6.81180436011734));
#68585=CARTESIAN_POINT('Ctrl Pts',(0.0969277403211786,-0.866509869209777,
-6.79062222879147));
#68586=CARTESIAN_POINT('Ctrl Pts',(0.765683559285303,-0.538859796515862,
-6.76414456463416));
#68587=CARTESIAN_POINT('Ctrl Pts',(0.866014837596959,0.354056683203798,
-6.73237136764536));
#68588=CARTESIAN_POINT('Ctrl Pts',(0.289333110659433,0.822525112548018,
-6.70589370348804));
#68589=CARTESIAN_POINT('Ctrl Pts',(-0.253849804187702,0.783424145888391,
-6.68471157216219));
#68590=CARTESIAN_POINT('Ctrl Pts',(-0.598921237881815,0.567797995500131,
-6.6688249736678));
#68591=CARTESIAN_POINT('Ctrl Pts',(-0.795626144337943,0.212537285908078,
-6.65293837517339));
#68592=CARTESIAN_POINT('Ctrl Pts',(-0.806176889005594,-0.333427828561512,
-6.63175624384755));
#68593=CARTESIAN_POINT('Ctrl Pts',(-0.407459771995628,-0.771654740532012,
-6.61057411252167));
#68594=CARTESIAN_POINT('Ctrl Pts',(0.13620949180056,-0.811342273578339,
-6.58939198119583));
#68595=CARTESIAN_POINT('Ctrl Pts',(0.63481469825267,-0.597699455562655,
-6.56820984986996));
#68596=CARTESIAN_POINT('Ctrl Pts',(0.932429169023787,0.0849531159557454,
-6.54173218571265));
#68597=CARTESIAN_POINT('Ctrl Pts',(0.430869109575266,0.830475561361244,
-6.50995898872384));
#68598=CARTESIAN_POINT('Ctrl Pts',(-0.31193659363892,0.814221567831034,
-6.48348132456654));
#68599=CARTESIAN_POINT('Ctrl Pts',(-0.700633496159194,0.432788416497904,
-6.46229919324067));
#68600=CARTESIAN_POINT('Ctrl Pts',(-0.824057702288797,0.045057274866246,
-6.44641259474628));
#68601=CARTESIAN_POINT('Ctrl Pts',(-0.744005417244997,-0.353056491979323,
-6.43052599625189));
#68602=CARTESIAN_POINT('Ctrl Pts',(-0.398615423024649,-0.776016311853889,
-6.40934386492602));
#68603=CARTESIAN_POINT('Ctrl Pts',(0.188970689385073,-0.851917996021742,
-6.38816173360017));
#68604=CARTESIAN_POINT('Ctrl Pts',(0.629041753542907,-0.530222355654872,
-6.36697960227431));
#68605=CARTESIAN_POINT('Ctrl Pts',(0.870772724474157,-0.0446115706622471,
-6.34579747094845));
#68606=CARTESIAN_POINT('Ctrl Pts',(0.655693065363436,0.668359420519961,
-6.31931980679113));
#68607=CARTESIAN_POINT('Ctrl Pts',(-0.209203633915283,0.911907381421729,
-6.28754660980234));
#68608=CARTESIAN_POINT('Ctrl Pts',(-0.764847329829675,0.41865527253801,
-6.26106894564502));
#68609=CARTESIAN_POINT('Ctrl Pts',(-0.814177759528614,-0.123683869477853,
-6.23988681431916));
#68610=CARTESIAN_POINT('Ctrl Pts',(-0.657268681575078,-0.499125649235067,
-6.22400021582476));
#68611=CARTESIAN_POINT('Ctrl Pts',(-0.338500623740867,-0.750707495992228,
-6.20811361733038));
#68612=CARTESIAN_POINT('Ctrl Pts',(0.198485975997741,-0.849568798889214,
-6.1869314860045));
#68613=CARTESIAN_POINT('Ctrl Pts',(0.695616949385993,-0.526894436738678,
-6.16574935467867));
#68614=CARTESIAN_POINT('Ctrl Pts',(0.822580645933705,0.00296536296201527,
-6.14456722335279));
#68615=CARTESIAN_POINT('Ctrl Pts',(0.692831037543227,0.52996466239058,-6.12338509202694));
#68616=CARTESIAN_POINT('Ctrl Pts',(0.0665577394891163,0.933309743473525,
-6.09690742786962));
#68617=CARTESIAN_POINT('Ctrl Pts',(-0.74885079779902,0.560609547756868,
-6.06513423088083));
#68618=CARTESIAN_POINT('Ctrl Pts',(-0.87668553612213,-0.325243430519842,
-6.03336103389204));
#68619=CARTESIAN_POINT('Ctrl Pts',(-0.201777547445245,-0.913042518007263,
-6.00158783690326));
#68620=CARTESIAN_POINT('Ctrl Pts',(0.658129706567036,-0.66477505348379,
-5.96981463991446));
#68621=CARTESIAN_POINT('Ctrl Pts',(0.915328905939503,0.194087619131439,
-5.93804144292568));
#68622=CARTESIAN_POINT('Ctrl Pts',(0.429806015838223,0.759041618565978,
-5.91156377876836));
#68623=CARTESIAN_POINT('Ctrl Pts',(-0.110017993077991,0.81519553092574,
-5.8903816474425));
#68624=CARTESIAN_POINT('Ctrl Pts',(-0.617424004674881,0.616675186942424,
-5.86919951611664));
#68625=CARTESIAN_POINT('Ctrl Pts',(-0.868776556752314,0.0799444879365195,
-5.84801738479078));
#68626=CARTESIAN_POINT('Ctrl Pts',(-0.697113753108197,-0.43837978060043,
-5.82683525346492));
#68627=CARTESIAN_POINT('Ctrl Pts',(-0.404142498383631,-0.719581388380777,
-5.81094865497054));
#68628=CARTESIAN_POINT('Ctrl Pts',(-0.0107108149795365,-0.823449088968177,
-5.79506205647612));
#68629=CARTESIAN_POINT('Ctrl Pts',(0.519716779792302,-0.700112950868486,
-5.77387992515028));
#68630=CARTESIAN_POINT('Ctrl Pts',(0.931996334502745,-0.0820003976102612,
-5.74740226099295));
#68631=CARTESIAN_POINT('Ctrl Pts',(0.571989477491768,0.741259568978487,
-5.71562906400416));
#68632=CARTESIAN_POINT('Ctrl Pts',(-0.163761877828015,0.856397908273568,
-5.68915139984685));
#68633=CARTESIAN_POINT('Ctrl Pts',(-0.611578414438477,0.550273674755984,
-5.66796926852098));
#68634=CARTESIAN_POINT('Ctrl Pts',(-0.869796878220926,0.0701967522717843,
-5.64678713719512));
#68635=CARTESIAN_POINT('Ctrl Pts',(-0.713927964402905,-0.501400472057978,
-5.62560500586928));
#68636=CARTESIAN_POINT('Ctrl Pts',(-0.247546526044699,-0.785438517556817,
-5.60442287454341));
#68637=CARTESIAN_POINT('Ctrl Pts',(0.157788538732795,-0.810064214593159,
-5.58853627604902));
#68638=CARTESIAN_POINT('Ctrl Pts',(0.524898314535317,-0.63456667797246,
-5.57264967755462));
#68639=CARTESIAN_POINT('Ctrl Pts',(0.849343000973622,-0.197174203863991,
-5.55146754622876));
#68640=CARTESIAN_POINT('Ctrl Pts',(0.763442303930618,0.540826863398601,
-5.52498988207145));
#68641=CARTESIAN_POINT('Ctrl Pts',(-0.0438911083957374,0.935261865875422,
-5.49321668508264));
#68642=CARTESIAN_POINT('Ctrl Pts',(-0.679209033401171,0.546726100752257,
-5.46673902092534));
#68643=CARTESIAN_POINT('Ctrl Pts',(-0.822360459076503,0.0235071457076657,
-5.44555688959947));
#68644=CARTESIAN_POINT('Ctrl Pts',(-0.708393220507744,-0.50956211546672,
-5.42437475827362));
#68645=CARTESIAN_POINT('Ctrl Pts',(-0.219566532678745,-0.844325666406878,
-5.40319262694775));
#68646=CARTESIAN_POINT('Ctrl Pts',(0.319777840880432,-0.758903941179043,
-5.38201049562191));
#68647=CARTESIAN_POINT('Ctrl Pts',(0.644662005989868,-0.515278673062417,
-5.36612389712749));
#68648=CARTESIAN_POINT('Ctrl Pts',(0.810860951904657,-0.143866716523886,
-5.35023729863312));
#68649=CARTESIAN_POINT('Ctrl Pts',(0.775002633482968,0.399539895117439,
-5.32905516730725));
#68650=CARTESIAN_POINT('Ctrl Pts',(0.231783132694296,0.906429486092428,
-5.30257750314994));
#68651=CARTESIAN_POINT('Ctrl Pts',(-0.638897434822695,0.684434994019087,
-5.27080430616114));
#68652=CARTESIAN_POINT('Ctrl Pts',(-0.871611353577846,-0.0229780024351207,
-5.24432664200383));
#68653=CARTESIAN_POINT('Ctrl Pts',(-0.642012997391936,-0.514440104259355,
-5.22314451067796));
#68654=CARTESIAN_POINT('Ctrl Pts',(-0.210064536928675,-0.846963633196215,
-5.20196237935211));
#68655=CARTESIAN_POINT('Ctrl Pts',(0.379224671095523,-0.785674195477476,
-5.18078024802624));
#68656=CARTESIAN_POINT('Ctrl Pts',(0.735010038690682,-0.371420654532431,
-5.15959811670039));
#68657=CARTESIAN_POINT('Ctrl Pts',(0.824922358102787,0.0245828391735762,
-5.14371151820599));
#68658=CARTESIAN_POINT('Ctrl Pts',(0.711163238398459,0.415258911722287,
-5.12782491971161));
#68659=CARTESIAN_POINT('Ctrl Pts',(0.332056770722144,0.806225471417083,
-5.10664278838573));
#68660=CARTESIAN_POINT('Ctrl Pts',(-0.410116348914915,0.840917602492415,
-5.08016512422843));
#68661=CARTESIAN_POINT('Ctrl Pts',(-0.930032409127722,0.108078264400297,
-5.04839192723962));
#68662=CARTESIAN_POINT('Ctrl Pts',(-0.649459303570146,-0.581753344032707,
-5.02191426308231));
#68663=CARTESIAN_POINT('Ctrl Pts',(-0.156312362641779,-0.807710192440725,
-5.00073213175645));
#68664=CARTESIAN_POINT('Ctrl Pts',(0.388174699197929,-0.781533689956709,
-4.97955000043059));
#68665=CARTESIAN_POINT('Ctrl Pts',(0.797649655718905,-0.353341646763458,
-4.95836786910473));
#68666=CARTESIAN_POINT('Ctrl Pts',(0.800657962051566,0.192717117539353,
-4.93718573777887));
#68667=CARTESIAN_POINT('Ctrl Pts',(0.612834485043679,0.552752301506898,
-4.92129913928448));
#68668=CARTESIAN_POINT('Ctrl Pts',(0.273223226583257,0.776879774398488,
-4.90541254079008));
#68669=CARTESIAN_POINT('Ctrl Pts',(-0.268821391201312,0.829455405297251,
-4.88423040946423));
#68670=CARTESIAN_POINT('Ctrl Pts',(-0.856956962236578,0.375449861770003,
-4.8577527453069));
#68671=CARTESIAN_POINT('Ctrl Pts',(-0.778826887468074,-0.519682472881723,
-4.82597954831812));
#68672=CARTESIAN_POINT('Ctrl Pts',(-0.118412479963754,-0.863836109962943,
-4.79950188416079));
#68673=CARTESIAN_POINT('Ctrl Pts',(0.403733302816536,-0.716818477638608,
-4.77831975283494));
#68674=CARTESIAN_POINT('Ctrl Pts',(0.801790918663602,-0.344391969104003,
-4.75713762150907));
#68675=CARTESIAN_POINT('Ctrl Pts',(0.836697813406502,0.247046679084701,
-4.73595549018323));
#68676=CARTESIAN_POINT('Ctrl Pts',(0.485498252731183,0.665195088815462,
-4.71477335885736));
#68677=CARTESIAN_POINT('Ctrl Pts',(0.109271274779151,0.818022616672709,
-4.69888676036297));
#68678=CARTESIAN_POINT('Ctrl Pts',(-0.294666770169491,0.769002347182303,
-4.68300016186857));
#68679=CARTESIAN_POINT('Ctrl Pts',(-0.741843161944716,0.458181113556748,
-4.66181803054272));
#68680=CARTESIAN_POINT('Ctrl Pts',(-0.896213104327743,-0.268588729212688,
-4.6353403663854));
#68681=CARTESIAN_POINT('Ctrl Pts',(-0.257196993176862,-0.900272680894212,
-4.60356716939661));
#68682=CARTESIAN_POINT('Ctrl Pts',(0.46895349403166,-0.735062555652628,
-4.57708950523928));
#68683=CARTESIAN_POINT('Ctrl Pts',(0.771755993962188,-0.284994728847248,
-4.55590737391343));
#68684=CARTESIAN_POINT('Ctrl Pts',(0.834060650473717,0.256548897807251,
-4.53472524258756));
#68685=CARTESIAN_POINT('Ctrl Pts',(0.477797123153197,0.729935066778223,
-4.51354311126171));
#68686=CARTESIAN_POINT('Ctrl Pts',(-0.0605733428831204,0.821294058009192,
-4.49236097993585));
#68687=CARTESIAN_POINT('Ctrl Pts',(-0.446263360789283,0.694226350477263,
-4.47647438144146));
#68688=CARTESIAN_POINT('Ctrl Pts',(-0.722407838794893,0.395373279144789,
-4.46058778294706));
#68689=CARTESIAN_POINT('Ctrl Pts',(-0.862030699206853,-0.131012531344061,
-4.4394056516212));
#68690=CARTESIAN_POINT('Ctrl Pts',(-0.509213832980306,-0.784881587330448,
-4.41292798746389));
#68691=CARTESIAN_POINT('Ctrl Pts',(0.386760515085133,-0.8526766662896,-4.38115479047509));
#68692=CARTESIAN_POINT('Ctrl Pts',(0.833276572853283,-0.256679748755051,
-4.35467712631777));
#68693=CARTESIAN_POINT('Ctrl Pts',(0.772717359300933,0.282377747569235,
-4.33349499499192));
#68694=CARTESIAN_POINT('Ctrl Pts',(0.469635817471363,0.735470396809251,
-4.31231286366604));
#68695=CARTESIAN_POINT('Ctrl Pts',(-0.108352654717711,0.865652929771297,
-4.29113073234021));
#68696=CARTESIAN_POINT('Ctrl Pts',(-0.57783514405307,0.586770488254485,
-4.26994860101433));
#68697=CARTESIAN_POINT('Ctrl Pts',(-0.789546945310624,0.240243280927042,
-4.25406200251995));
#68698=CARTESIAN_POINT('Ctrl Pts',(-0.806558470603616,-0.166302582395967,
-4.23817540402555));
#68699=CARTESIAN_POINT('Ctrl Pts',(-0.572220602744597,-0.657894209990364,
-4.2169932726997));
#68700=CARTESIAN_POINT('Ctrl Pts',(0.119976890218829,-0.927870346353562,
-4.19051560854236));
#68701=CARTESIAN_POINT('Ctrl Pts',(0.846767618623912,-0.399531967824429,
-4.15874241155359));
#68702=CARTESIAN_POINT('Ctrl Pts',(0.801278008580111,0.343784661165928,
-4.13226474739625));
#68703=CARTESIAN_POINT('Ctrl Pts',(0.406160155819965,0.715446180723319,
-4.1110826160704));
#68704=CARTESIAN_POINT('Ctrl Pts',(-0.118156436265154,0.864588666478961,
-4.08990048474454));
#68705=CARTESIAN_POINT('Ctrl Pts',(-0.642967919858539,0.589650359652897,
-4.06871835341868));
#68706=CARTESIAN_POINT('Ctrl Pts',(-0.820267937436497,0.0731680968928279,
-4.04753622209283));
#68707=CARTESIAN_POINT('Ctrl Pts',(-0.7573075007919,-0.328003905653948,
-4.03164962359843));
#68708=CARTESIAN_POINT('Ctrl Pts',(-0.507095079487041,-0.648881881218796,
-4.01576302510404));
#68709=CARTESIAN_POINT('Ctrl Pts',(-0.0102518774661032,-0.871869318621008,
-3.99458089377819));
#68710=CARTESIAN_POINT('Ctrl Pts',(0.692104400777655,-0.629546926172355,
-3.96810322962085));
#68711=CARTESIAN_POINT('Ctrl Pts',(0.904036489905212,0.243637472863961,
-3.93633003263208));
#68712=CARTESIAN_POINT('Ctrl Pts',(0.388176906107868,0.78073877183831,-3.90985236847474));
#68713=CARTESIAN_POINT('Ctrl Pts',(-0.153574277836826,0.80823526950646,
-3.88867023714889));
#68714=CARTESIAN_POINT('Ctrl Pts',(-0.649751318698528,0.582492686206687,
-3.86748810582302));
#68715=CARTESIAN_POINT('Ctrl Pts',(-0.871775832726098,0.033199248195006,
-3.84630597449717));
#68716=CARTESIAN_POINT('Ctrl Pts',(-0.672566233662919,-0.475234385251865,
-3.82512384317131));
#68717=CARTESIAN_POINT('Ctrl Pts',(-0.364878699197954,-0.740246410157821,
-3.80923724467692));
#68718=CARTESIAN_POINT('Ctrl Pts',(0.0335520454040853,-0.822841039121903,
-3.79335064618252));
#68719=CARTESIAN_POINT('Ctrl Pts',(0.556592829034656,-0.671167365424921,
-3.77216851485667));
#68720=CARTESIAN_POINT('Ctrl Pts',(0.935054346233315,-0.0317994248225427,
-3.74569085069934));
#68721=CARTESIAN_POINT('Ctrl Pts',(0.531329001872747,0.770928456494234,
-3.71391765371055));
#68722=CARTESIAN_POINT('Ctrl Pts',(-0.209548262673311,0.846359182556483,
-3.68743998955324));
#68723=CARTESIAN_POINT('Ctrl Pts',(-0.640265964208693,0.516612819007808,
-3.66625785822737));
#68724=CARTESIAN_POINT('Ctrl Pts',(-0.872312539777597,0.0233524855530796,
-3.64507572690152));
#68725=CARTESIAN_POINT('Ctrl Pts',(-0.685951147375653,-0.539042035485203,
-3.62389359557565));
#68726=CARTESIAN_POINT('Ctrl Pts',(-0.204979675929423,-0.797606664995417,
-3.60271146424981));
#68727=CARTESIAN_POINT('Ctrl Pts',(0.201093113573265,-0.800414125658291,
-3.5868248657554));
#68728=CARTESIAN_POINT('Ctrl Pts',(0.558241201240319,-0.605441885445481,
-3.57093826726101));
#68729=CARTESIAN_POINT('Ctrl Pts',(0.85871176293571,-0.151245885696385,
-3.54975613593516));
#68730=CARTESIAN_POINT('Ctrl Pts',(0.733275270191108,0.581072467042636,
-3.52327847177783));
#68731=CARTESIAN_POINT('Ctrl Pts',(-0.0940883185327613,0.931551706336986,
-3.49150527478904));
#68732=CARTESIAN_POINT('Ctrl Pts',(-0.707608428889974,0.509435620712697,
-3.46502761063172));
#68733=CARTESIAN_POINT('Ctrl Pts',(-0.822435398042004,-0.0207201769966671,
-3.44384547930586));
#68734=CARTESIAN_POINT('Ctrl Pts',(-0.679985894907103,-0.546894586151797,
-3.42266334798001));
#68735=CARTESIAN_POINT('Ctrl Pts',(-0.173875497258729,-0.854905026338613,
-3.40148121665414));
#68736=CARTESIAN_POINT('Ctrl Pts',(0.360098980600512,-0.740622564981457,
-3.38029908532829));
#68737=CARTESIAN_POINT('Ctrl Pts',(0.671421347990293,-0.479890181544519,
-3.36441248683389));
#68738=CARTESIAN_POINT('Ctrl Pts',(0.817420588379709,-0.100083450714793,
-3.3485258883395));
#68739=CARTESIAN_POINT('Ctrl Pts',(0.752411610162823,0.440610915248839,
-3.32734375701365));
#68740=CARTESIAN_POINT('Ctrl Pts',(0.182737007354738,0.917575620846529,
-3.30086609285632));
#68741=CARTESIAN_POINT('Ctrl Pts',(-0.674755506495149,0.649111854550621,
-3.26909289586753));
#68742=CARTESIAN_POINT('Ctrl Pts',(-0.869117029466048,-0.0697848793019947,
-3.24261523171021));
#68743=CARTESIAN_POINT('Ctrl Pts',(-0.613439450643915,-0.548198276247722,
-3.22143310038435));
#68744=CARTESIAN_POINT('Ctrl Pts',(-0.164245468909761,-0.857028547702678,
-3.2002509690585));
#68745=CARTESIAN_POINT('Ctrl Pts',(0.42089853297893,-0.764159484363172,
-3.17906883773263));
#68746=CARTESIAN_POINT('Ctrl Pts',(0.753907947908702,-0.331384769821025,
-3.15788670640678));
#68747=CARTESIAN_POINT('Ctrl Pts',(0.822409257101771,0.0688783472016456,
-3.14200010791238));
#68748=CARTESIAN_POINT('Ctrl Pts',(0.687819729871631,0.452876511439188,
-3.12611350941799));
#68749=CARTESIAN_POINT('Ctrl Pts',(0.288250675822232,0.822905072066193,
-3.10493137809213));
#68750=CARTESIAN_POINT('Ctrl Pts',(-0.454714332566075,0.817662955983605,
-3.07845371393481));
#68751=CARTESIAN_POINT('Ctrl Pts',(-0.934496582127582,0.05794248230392,
-3.04668051694602));
#68752=CARTESIAN_POINT('Ctrl Pts',(-0.61725760748963,-0.615814408960401,
-3.0202028527887));
#68753=CARTESIAN_POINT('Ctrl Pts',(-0.112680433289495,-0.814943206389853,
-2.99902072146284));
#68754=CARTESIAN_POINT('Ctrl Pts',(0.429613118847823,-0.759543990660583,
-2.97783859013698));
#68755=CARTESIAN_POINT('Ctrl Pts',(0.815485490159638,-0.309965656073528,
-2.95665645881112));
#68756=CARTESIAN_POINT('Ctrl Pts',(0.789144447933524,0.235465708511735,
-2.93547432748526));
#68757=CARTESIAN_POINT('Ctrl Pts',(0.58224421809318,0.584887068909028,-2.91958772899087));
#68758=CARTESIAN_POINT('Ctrl Pts',(0.231079174441137,0.790440086631248,
-2.90370113049647));
#68759=CARTESIAN_POINT('Ctrl Pts',(-0.313007574327803,0.813810462059596,
-2.88251899917062));
#68760=CARTESIAN_POINT('Ctrl Pts',(-0.875895184041176,0.328854770989161,
-2.85604133501329));
#68761=CARTESIAN_POINT('Ctrl Pts',(-0.749773919115458,-0.560785398773811,
-2.82426813802451));
#68762=CARTESIAN_POINT('Ctrl Pts',(-0.0718191300318257,-0.868951294865558,
-2.79779047386718));
#68763=CARTESIAN_POINT('Ctrl Pts',(0.441671467773378,-0.694086179261763,
-2.77660834254133));
#68764=CARTESIAN_POINT('Ctrl Pts',(0.81913981644577,-0.300806360883462,
-2.75542621121547));
#68765=CARTESIAN_POINT('Ctrl Pts',(0.822212569948914,0.291653531478696,
-2.73424407988961));
#68766=CARTESIAN_POINT('Ctrl Pts',(0.449049354063659,0.690324371005584,
-2.71306194856375));
#68767=CARTESIAN_POINT('Ctrl Pts',(0.0651531347017874,0.822712757843502,
-2.69717535006936));
#68768=CARTESIAN_POINT('Ctrl Pts',(-0.335566880655414,0.752055838366545,
-2.68128875157496));
#68769=CARTESIAN_POINT('Ctrl Pts',(-0.765393673021599,0.417652648791717,
-2.66010662024911));
#68770=CARTESIAN_POINT('Ctrl Pts',(-0.880484198151439,-0.316362783263885,
-2.63362895609178));
#68771=CARTESIAN_POINT('Ctrl Pts',(-0.208445008845069,-0.912793444077713,
-2.601855759103));
#68772=CARTESIAN_POINT('Ctrl Pts',(0.507777844793081,-0.708798984638362,
-2.57537809494567));
#68773=CARTESIAN_POINT('Ctrl Pts',(0.785956306448284,-0.243109016783524,
-2.55419596361982));
#68774=CARTESIAN_POINT('Ctrl Pts',(0.819068571950472,0.301000299132349,
-2.53301383229395));
#68775=CARTESIAN_POINT('Ctrl Pts',(0.437880249640628,0.754556942570053,
-2.5118317009681));
#68776=CARTESIAN_POINT('Ctrl Pts',(-0.104621860425811,0.816852083250257,
-2.49064956964224));
#68777=CARTESIAN_POINT('Ctrl Pts',(-0.482925976241363,0.669241148130661,
-2.47476297114785));
#68778=CARTESIAN_POINT('Ctrl Pts',(-0.742611163852711,0.355980020135029,
-2.45887637265345));
#68779=CARTESIAN_POINT('Ctrl Pts',(-0.853744482606572,-0.177148435395509,
-2.4376942413276));
#68780=CARTESIAN_POINT('Ctrl Pts',(-0.466298755498204,-0.811112387064631,
-2.41121657717027));
#68781=CARTESIAN_POINT('Ctrl Pts',(0.432024176205328,-0.830660161821777,
-2.37944338018149));
#68782=CARTESIAN_POINT('Ctrl Pts',(0.845866350123333,-0.21152885858932,
-2.35296571602416));
#68783=CARTESIAN_POINT('Ctrl Pts',(0.756425889876396,0.323495259334638,
-2.33178358469831));
#68784=CARTESIAN_POINT('Ctrl Pts',(0.429433270552451,0.759645688316193,
-2.31060145337244));
#68785=CARTESIAN_POINT('Ctrl Pts',(-0.154715960077263,0.858579212596816,
-2.28941932204659));
#68786=CARTESIAN_POINT('Ctrl Pts',(-0.608532996475014,0.554869941328941,
-2.26823719072073));
#68787=CARTESIAN_POINT('Ctrl Pts',(-0.801316622834949,0.19746615620993,
-2.25235059222633));
#68788=CARTESIAN_POINT('Ctrl Pts',(-0.796455937755181,-0.209406434066689,
-2.23646399373194));
#68789=CARTESIAN_POINT('Ctrl Pts',(-0.536038735277689,-0.687694469969133,
-2.21528186240609));
#68790=CARTESIAN_POINT('Ctrl Pts',(0.169666939921909,-0.920082041628023,
-2.18880419824875));
#68791=CARTESIAN_POINT('Ctrl Pts',(0.867014727932226,-0.35344964961403,
-2.15703100125997));
#68792=CARTESIAN_POINT('Ctrl Pts',(0.781645283048855,0.386348277820098,
-2.13055333710265));
#68793=CARTESIAN_POINT('Ctrl Pts',(0.367125426573497,0.73623924837685,-2.10937120577679));
#68794=CARTESIAN_POINT('Ctrl Pts',(-0.164448381852627,0.856989635492053,
-2.08818907445093));
#68795=CARTESIAN_POINT('Ctrl Pts',(-0.673726417467051,0.554245439325413,
-2.06700694312507));
#68796=CARTESIAN_POINT('Ctrl Pts',(-0.82301466228896,0.0289814638455597,
-2.04582481179922));
#68797=CARTESIAN_POINT('Ctrl Pts',(-0.738586365580606,-0.368227366525561,
-2.02993821330482));
#68798=CARTESIAN_POINT('Ctrl Pts',(-0.471491638911371,-0.675195341994213,
-2.01405161481043));
#68799=CARTESIAN_POINT('Ctrl Pts',(0.0366168801367174,-0.871160383530664,
-1.99286948348457));
#68800=CARTESIAN_POINT('Ctrl Pts',(0.724935922390556,-0.591443777764724,
-1.96639181932725));
#68801=CARTESIAN_POINT('Ctrl Pts',(0.889637150329744,0.291868007868019,
-1.93461862233846));
#68802=CARTESIAN_POINT('Ctrl Pts',(0.345659362638246,0.800471077121211,
-1.90814095818114));
#68803=CARTESIAN_POINT('Ctrl Pts',(-0.196786632712784,0.798814328159457,
-1.88695882685528));
#68804=CARTESIAN_POINT('Ctrl Pts',(-0.680115363374823,0.546733571437031,
-1.86577669552942));
#68805=CARTESIAN_POINT('Ctrl Pts',(-0.872300216170217,-0.0136976448847273,
-1.84459456420356));
#68806=CARTESIAN_POINT('Ctrl Pts',(-0.64605543815613,-0.510691130154158,
-1.82341243287771));
#68807=CARTESIAN_POINT('Ctrl Pts',(-0.324570867014354,-0.758785190396783,
-1.80752583438331));
#68808=CARTESIAN_POINT('Ctrl Pts',(0.0777227434299177,-0.819848943749846,
-1.79163923588892));
#68809=CARTESIAN_POINT('Ctrl Pts',(0.591856834804682,-0.640286417815664,
-1.77045710456306));
#68810=CARTESIAN_POINT('Ctrl Pts',(0.93541206505034,0.0184960100323257,
-1.74397944040574));
#68811=CARTESIAN_POINT('Ctrl Pts',(0.489131803792666,0.798367879979027,
-1.71220624341694));
#68812=CARTESIAN_POINT('Ctrl Pts',(-0.254728499474417,0.833875129646275,
-1.68572857925963));
#68813=CARTESIAN_POINT('Ctrl Pts',(-0.66710335504059,0.481458641402219,
-1.66454644793376));
#68814=CARTESIAN_POINT('Ctrl Pts',(-0.872306986188969,-0.0235590212162755,
-1.64336431660791));
#68815=CARTESIAN_POINT('Ctrl Pts',(-0.655992010257842,-0.575125877598879,
-1.62218218528205));
#68816=CARTESIAN_POINT('Ctrl Pts',(-0.161820381338305,-0.807469642632321,
-1.60100005395619));
#68817=CARTESIAN_POINT('Ctrl Pts',(0.243816497396363,-0.788450840875503,
-1.5851134554618));
#68818=CARTESIAN_POINT('Ctrl Pts',(0.589970761438499,-0.574567329441633,
-1.5692268569674));
#68819=CARTESIAN_POINT('Ctrl Pts',(0.865598808023936,-0.104880471450991,
-1.54804472564155));
#68820=CARTESIAN_POINT('Ctrl Pts',(0.700989048572545,0.619638755736126,
-1.52156706148422));
#68821=CARTESIAN_POINT('Ctrl Pts',(-0.144013612661718,0.925149324504857,
-1.48979386449544));
#68822=CARTESIAN_POINT('Ctrl Pts',(-0.733962808560724,0.470672854471897,
-1.46331620033811));
#68823=CARTESIAN_POINT('Ctrl Pts',(-0.82013346881962,-0.0648876183040882,
-1.44213406901226));
#68824=CARTESIAN_POINT('Ctrl Pts',(-0.649613384442308,-0.582646510663345,
-1.42095193768639));
#68825=CARTESIAN_POINT('Ctrl Pts',(-0.127681955460861,-0.863013679413998,
-1.39976980636054));
#68826=CARTESIAN_POINT('Ctrl Pts',(0.399379421048456,-0.720200762032534,
-1.37858767503468));
#68827=CARTESIAN_POINT('Ctrl Pts',(0.696240257393158,-0.443114789715985,
-1.36270107654028));
#68828=CARTESIAN_POINT('Ctrl Pts',(0.821617849133442,-0.0560109399970021,
-1.34681447804589));
#68829=CARTESIAN_POINT('Ctrl Pts',(0.72764608942882,0.48040855350751,-1.32563234672003));
#68830=CARTESIAN_POINT('Ctrl Pts',(0.133162765313291,0.926069928117188,
-1.29915468256271));
#68831=CARTESIAN_POINT('Ctrl Pts',(-0.708663509792098,0.611912757795438,
-1.26738148557392));
#68832=CARTESIAN_POINT('Ctrl Pts',(-0.864110924976073,-0.116390075281674,
-1.2409038214166));
#68833=CARTESIAN_POINT('Ctrl Pts',(-0.583093041185656,-0.580372134934255,
-1.21972169009074));
#68834=CARTESIAN_POINT('Ctrl Pts',(-0.117951725407047,-0.864616617992188,
-1.19853955876488));
#68835=CARTESIAN_POINT('Ctrl Pts',(0.461355982526874,-0.7404363240635,-1.17735742743902));
#68836=CARTESIAN_POINT('Ctrl Pts',(0.770627035260557,-0.290391170862284,
-1.15617529611317));
#68837=CARTESIAN_POINT('Ctrl Pts',(0.817519362915898,0.112974794257399,
-1.14028869761877));
#68838=CARTESIAN_POINT('Ctrl Pts',(0.66248839687407,0.48918528128025,-1.12440209912438));
#68839=CARTESIAN_POINT('Ctrl Pts',(0.243611525802989,0.837206446606919,
-1.10321996779852));
#68840=CARTESIAN_POINT('Ctrl Pts',(-0.497998174970216,0.79204523327596,
-1.0767423036412));
#68841=CARTESIAN_POINT('Ctrl Pts',(-0.936260025425832,0.00763924428965602,
-1.04496910665241));
#68842=CARTESIAN_POINT('Ctrl Pts',(-0.583272014082999,-0.648095747459154,
-1.01849144249509));
#68843=CARTESIAN_POINT('Ctrl Pts',(-0.0687228533155248,-0.819821004317041,
-0.997309311169228));
#68844=CARTESIAN_POINT('Ctrl Pts',(0.469809940687286,-0.735359181126046,
-0.976127179843371));
#68845=CARTESIAN_POINT('Ctrl Pts',(0.830964541358147,-0.265693853167689,
-0.954945048517511));
#68846=CARTESIAN_POINT('Ctrl Pts',(0.775350277160346,0.277533794873319,
-0.933762917191653));
#68847=CARTESIAN_POINT('Ctrl Pts',(0.549971243807159,0.615331491039807,
-0.917876318697261));
#68848=CARTESIAN_POINT('Ctrl Pts',(0.188267294934982,0.801715997764048,
-0.901989720202864));
#68849=CARTESIAN_POINT('Ctrl Pts',(-0.356289153983751,0.795813576474891,
-0.880807588877008));
#68850=CARTESIAN_POINT('Ctrl Pts',(-0.892302036349828,0.281309277747789,
-0.854329924719686));
#68851=CARTESIAN_POINT('Ctrl Pts',(-0.718554076398238,-0.600267634106091,
-0.822556727730897));
#68852=CARTESIAN_POINT('Ctrl Pts',(-0.0250182201471705,-0.871555178383084,
-0.796079063573576));
#68853=CARTESIAN_POINT('Ctrl Pts',(0.478333185832665,-0.669347946128884,
-0.774896932247718));
#68854=CARTESIAN_POINT('Ctrl Pts',(0.834121369879876,-0.256351411186756,
-0.75371480092186));
#68855=CARTESIAN_POINT('Ctrl Pts',(0.805351101674305,0.335417494451096,
-0.732532669596));
#68856=CARTESIAN_POINT('Ctrl Pts',(0.411302686227501,0.713458590124914,
-0.711350538270145));
#68857=CARTESIAN_POINT('Ctrl Pts',(0.0208466994859789,0.825025228897732,
-0.695463939775747));
#68858=CARTESIAN_POINT('Ctrl Pts',(-0.375497190132326,0.732935859991011,
-0.679577341281356));
#68859=CARTESIAN_POINT('Ctrl Pts',(-0.786732168724632,0.375917153191761,
-0.658395209955497));
#68860=CARTESIAN_POINT('Ctrl Pts',(-0.86221065869004,-0.363222538767329,
-0.631917545798175));
#68861=CARTESIAN_POINT('Ctrl Pts',(-0.159090613120796,-0.922676197632793,
-0.600144348809385));
#68862=CARTESIAN_POINT('Ctrl Pts',(0.545134702812622,-0.680486963024897,
-0.573666684652064));
#68863=CARTESIAN_POINT('Ctrl Pts',(0.797885170775076,-0.20052070441559,
-0.552484553326204));
#68864=CARTESIAN_POINT('Ctrl Pts',(0.801709368724974,0.344581782361119,
-0.531302422000347));
#68865=CARTESIAN_POINT('Ctrl Pts',(0.396697857986909,0.776998153601058,
-0.510120290674489));
#68866=CARTESIAN_POINT('Ctrl Pts',(-0.14836798230013,0.81004933530726,-0.48893815934863));
#68867=CARTESIAN_POINT('Ctrl Pts',(-0.518192989793109,0.642321898247082,
-0.473051560854238));
#68868=CARTESIAN_POINT('Ctrl Pts',(-0.760668183767484,0.315557812215962,
-0.457164962359843));
#68869=CARTESIAN_POINT('Ctrl Pts',(-0.842991196767877,-0.222772042303558,
-0.435982831033984));
#68870=CARTESIAN_POINT('Ctrl Pts',(-0.42203547005247,-0.834999727972205,
-0.409505166876662));
#68871=CARTESIAN_POINT('Ctrl Pts',(0.476038245560472,-0.80624182046484,
-0.377731969887874));
#68872=CARTESIAN_POINT('Ctrl Pts',(0.856013262987149,-0.165768651945676,
-0.351254305730552));
#68873=CARTESIAN_POINT('Ctrl Pts',(0.737946030751173,0.363680533637555,
-0.330072174404693));
#68874=CARTESIAN_POINT('Ctrl Pts',(0.387995544781613,0.781618685293715,
-0.308890043078836));
#68875=CARTESIAN_POINT('Ctrl Pts',(-0.200644125565596,0.849038180119929,
-0.287707911752977));
#68876=CARTESIAN_POINT('Ctrl Pts',(-0.637457343762986,0.521348487027652,
-0.266525780427118));
#68877=CARTESIAN_POINT('Ctrl Pts',(-0.810801308960607,0.154154372617482,
-0.250639181932725));
#68878=CARTESIAN_POINT('Ctrl Pts',(-0.783995360021825,-0.251970803616545,
-0.23475258343833));
#68879=CARTESIAN_POINT('Ctrl Pts',(-0.498429251676069,-0.715365288338213,
-0.213570452112473));
#68880=CARTESIAN_POINT('Ctrl Pts',(0.219118145102592,-0.909928416986752,
-0.187092787955149));
#68881=CARTESIAN_POINT('Ctrl Pts',(0.884316580820022,-0.305832475245307,
-0.155319590966362));
#68882=CARTESIAN_POINT('Ctrl Pts',(0.760492323845775,0.426932666048197,
-0.128841926809039));
#68883=CARTESIAN_POINT('Ctrl Pts',(0.32603470475945,0.756065290736446,-0.107659795483181));
#68884=CARTESIAN_POINT('Ctrl Pts',(-0.0741110827836955,0.821794729598117,
-0.0917731969887856));
#68885=CARTESIAN_POINT('Ctrl Pts',(-0.459293844256021,0.685000114437588,
-0.0758865984943949));
#68886=CARTESIAN_POINT('Ctrl Pts',(-0.640103745128917,0.483143622270636,
-0.0652955328314636));
#68887=CARTESIAN_POINT('Ctrl Pts',(-0.701077753000047,0.366509473613445,
-0.0599999999999987));
#68888=CARTESIAN_POINT('Ctrl Pts',(0.437168237015721,-0.613060138694139,
-11.9529325805302));
#68889=CARTESIAN_POINT('Ctrl Pts',(0.539159417089925,-0.540331051333857,
-11.9476370476987));
#68890=CARTESIAN_POINT('Ctrl Pts',(0.705834142587216,-0.343484520089658,
-11.9370459820358));
#68891=CARTESIAN_POINT('Ctrl Pts',(0.784458452235278,0.0375372744664799,
-11.9211593835414));
#68892=CARTESIAN_POINT('Ctrl Pts',(0.670191340654958,0.406196224080167,
-11.905272785047));
#68893=CARTESIAN_POINT('Ctrl Pts',(0.303108267623569,0.772777165643128,
-11.8840906537212));
#68894=CARTESIAN_POINT('Ctrl Pts',(-0.403912271093399,0.793744592728965,
-11.8576129895638));
#68895=CARTESIAN_POINT('Ctrl Pts',(-0.886501473350934,0.0876535971293119,
-11.8258397925751));
#68896=CARTESIAN_POINT('Ctrl Pts',(-0.609288364385278,-0.563407023952644,
-11.7993621284177));
#68897=CARTESIAN_POINT('Ctrl Pts',(-0.135085777497467,-0.772068029013216,
-11.7781799970919));
#68898=CARTESIAN_POINT('Ctrl Pts',(0.251304709598349,-0.74425999429876,
-11.7622933985975));
#68899=CARTESIAN_POINT('Ctrl Pts',(0.574832343924073,-0.532842736520013,
-11.7464068001031));
#68900=CARTESIAN_POINT('Ctrl Pts',(0.8266807971614,-0.0781949429499539,
-11.7252246687772));
#68901=CARTESIAN_POINT('Ctrl Pts',(0.686184366139097,0.467951511691284,
-11.7040425374514));
#68902=CARTESIAN_POINT('Ctrl Pts',(0.246422156911299,0.743253963547303,
-11.6828604061255));
#68903=CARTESIAN_POINT('Ctrl Pts',(-0.268163586381898,0.785366976684619,
-11.6616782747996));
#68904=CARTESIAN_POINT('Ctrl Pts',(-0.82232695935117,0.343424645220471,
-11.6352006106423));
#68905=CARTESIAN_POINT('Ctrl Pts',(-0.732061997464235,-0.507020546474788,
-11.6034274136535));
#68906=CARTESIAN_POINT('Ctrl Pts',(-0.0998470505031248,-0.823871915212379,
-11.5769497494962));
#68907=CARTESIAN_POINT('Ctrl Pts',(0.396920405700097,-0.675900179016633,
-11.5557676181703));
#68908=CARTESIAN_POINT('Ctrl Pts',(0.673296005380202,-0.404591498794211,
-11.539881019676));
#68909=CARTESIAN_POINT('Ctrl Pts',(0.783090425855826,-0.0340058084353497,
-11.5239944211816));
#68910=CARTESIAN_POINT('Ctrl Pts',(0.680690834182767,0.47555198557487,-11.5028122898557));
#68911=CARTESIAN_POINT('Ctrl Pts',(0.220082416614076,0.800872619360714,
-11.4816301585298));
#68912=CARTESIAN_POINT('Ctrl Pts',(-0.293329865373632,0.726022874064885,
-11.460448027204));
#68913=CARTESIAN_POINT('Ctrl Pts',(-0.712798547359122,0.425003488822047,
-11.4392658958781));
#68914=CARTESIAN_POINT('Ctrl Pts',(-0.849088317678126,-0.270580441077998,
-11.4127882317208));
#68915=CARTESIAN_POINT('Ctrl Pts',(-0.229749102076862,-0.860348396266937,
-11.381015034732));
#68916=CARTESIAN_POINT('Ctrl Pts',(0.457232564597481,-0.692583893641502,
-11.3545373705747));
#68917=CARTESIAN_POINT('Ctrl Pts',(0.740074896800098,-0.258217496975165,
-11.3333552392488));
#68918=CARTESIAN_POINT('Ctrl Pts',(0.775093214744087,0.127483861482161,
-11.3174686407544));
#68919=CARTESIAN_POINT('Ctrl Pts',(0.618878123555508,0.481016576484203,
-11.3015820422601));
#68920=CARTESIAN_POINT('Ctrl Pts',(0.210966531938114,0.80310821135501,-11.2803999109342));
#68921=CARTESIAN_POINT('Ctrl Pts',(-0.350702013875208,0.75288864389604,
-11.2592177796083));
#68922=CARTESIAN_POINT('Ctrl Pts',(-0.693566003923817,0.363480166947511,
-11.2380356482825));
#68923=CARTESIAN_POINT('Ctrl Pts',(-0.81841553912867,-0.137498109807854,
-11.2168535169566));
#68924=CARTESIAN_POINT('Ctrl Pts',(-0.472006417340506,-0.755893307477461,
-11.1903758527993));
#68925=CARTESIAN_POINT('Ctrl Pts',(0.381835965208045,-0.804478284119145,
-11.1586026558105));
#68926=CARTESIAN_POINT('Ctrl Pts',(0.796844322343783,-0.231890474878377,
-11.1321249916532));
#68927=CARTESIAN_POINT('Ctrl Pts',(0.731236012504642,0.282278272840807,
-11.1109428603273));
#68928=CARTESIAN_POINT('Ctrl Pts',(0.508241943232004,0.598925498983947,
-11.0950562618329));
#68929=CARTESIAN_POINT('Ctrl Pts',(0.160315976071488,0.767258669906312,
-11.0791696633385));
#68930=CARTESIAN_POINT('Ctrl Pts',(-0.359097293392396,0.748691398822516,
-11.0579875320127));
#68931=CARTESIAN_POINT('Ctrl Pts',(-0.754686142027795,0.346817011706505,
-11.0368054006868));
#68932=CARTESIAN_POINT('Ctrl Pts',(-0.763929405500613,-0.171940387934335,
-11.015623269361));
#68933=CARTESIAN_POINT('Ctrl Pts',(-0.534779073333243,-0.634603078779137,
-10.9944411380351));
#68934=CARTESIAN_POINT('Ctrl Pts',(0.129570407511939,-0.881689435003545,
-10.9679634738778));
#68935=CARTESIAN_POINT('Ctrl Pts',(0.811812832458132,-0.365983522865465,
-10.936190276889));
#68936=CARTESIAN_POINT('Ctrl Pts',(0.757462285313874,0.339094312418124,
-10.9097126127317));
#68937=CARTESIAN_POINT('Ctrl Pts',(0.374607849449645,0.688517311643914,
-10.8885304814058));
#68938=CARTESIAN_POINT('Ctrl Pts',(-0.000338531309959313,0.78550716838858,
-10.8726438829114));
#68939=CARTESIAN_POINT('Ctrl Pts',(-0.374495394303978,0.688578447509876,
-10.856757284417));
#68940=CARTESIAN_POINT('Ctrl Pts',(-0.758367850255281,0.338183205514494,
-10.8355751530912));
#68941=CARTESIAN_POINT('Ctrl Pts',(-0.799727679520165,-0.224207161319477,
-10.8143930217653));
#68942=CARTESIAN_POINT('Ctrl Pts',(-0.47095395048083,-0.62558293624273,
-10.7932108904395));
#68943=CARTESIAN_POINT('Ctrl Pts',(0.00320814217882656,-0.829879167526741,
-10.7720287591136));
#68944=CARTESIAN_POINT('Ctrl Pts',(0.669521166699254,-0.588137872986708,
-10.7455510949563));
#68945=CARTESIAN_POINT('Ctrl Pts',(0.855676605772496,0.246579723996904,
-10.7137778979675));
#68946=CARTESIAN_POINT('Ctrl Pts',(0.357817272849018,0.748799616478352,
-10.6873002338102));
#68947=CARTESIAN_POINT('Ctrl Pts',(-0.160190687341481,0.767284870821596,
-10.6661181024843));
#68948=CARTESIAN_POINT('Ctrl Pts',(-0.508757994142515,0.598487200856775,
-10.6502315039899));
#68949=CARTESIAN_POINT('Ctrl Pts',(-0.731189876677205,0.282397668146848,
-10.6343449054955));
#68950=CARTESIAN_POINT('Ctrl Pts',(-0.796944728362207,-0.233171131850758,
-10.6131627741697));
#68951=CARTESIAN_POINT('Ctrl Pts',(-0.464404043789838,-0.688594290340323,
-10.5919806428438));
#68952=CARTESIAN_POINT('Ctrl Pts',(0.0460158535429895,-0.781686749800895,
-10.5707985115179));
#68953=CARTESIAN_POINT('Ctrl Pts',(0.539669506345693,-0.630449481554002,
-10.5496163801921));
#68954=CARTESIAN_POINT('Ctrl Pts',(0.891035361704283,-0.0148571360691248,
-10.5231387160348));
#68955=CARTESIAN_POINT('Ctrl Pts',(0.492564868907406,0.741865125121111,
-10.491365519046));
#68956=CARTESIAN_POINT('Ctrl Pts',(-0.212012206722167,0.802362069509788,
-10.4648878548886));
#68957=CARTESIAN_POINT('Ctrl Pts',(-0.618799590961628,0.481117652480525,
-10.4437057235628));
#68958=CARTESIAN_POINT('Ctrl Pts',(-0.775202810447137,0.126815727999937,
-10.4278191250684));
#68959=CARTESIAN_POINT('Ctrl Pts',(-0.74011702371455,-0.258096629071203,
-10.411932526574));
#68960=CARTESIAN_POINT('Ctrl Pts',(-0.456480055932384,-0.693624996182262,
-10.3907503952481));
#68961=CARTESIAN_POINT('Ctrl Pts',(0.0917986850181122,-0.825473327253274,
-10.3695682639223));
#68962=CARTESIAN_POINT('Ctrl Pts',(0.541099672434501,-0.56600598767403,
-10.3483861325964));
#68963=CARTESIAN_POINT('Ctrl Pts',(0.81945414101959,-0.131166442495638,
-10.3272040012706));
#68964=CARTESIAN_POINT('Ctrl Pts',(0.688756772763614,0.565489927648501,
-10.3007263371132));
#68965=CARTESIAN_POINT('Ctrl Pts',(-0.104819766699716,0.884305846673958,
-10.2689531401245));
#68966=CARTESIAN_POINT('Ctrl Pts',(-0.681004786683215,0.474306385052725,
-10.2424754759671));
#68967=CARTESIAN_POINT('Ctrl Pts',(-0.783096043438991,-0.0338779582154253,
-10.2212933446413));
#68968=CARTESIAN_POINT('Ctrl Pts',(-0.672946931715876,-0.405171634356951,
-10.2054067461469));
#68969=CARTESIAN_POINT('Ctrl Pts',(-0.397030920317412,-0.675835428963228,
-10.1895201476525));
#68970=CARTESIAN_POINT('Ctrl Pts',(0.101094915407747,-0.824178072306936,
-10.1683380163266));
#68971=CARTESIAN_POINT('Ctrl Pts',(0.604340273136911,-0.569742088003379,
-10.1471558850008));
#68972=CARTESIAN_POINT('Ctrl Pts',(0.778826548572907,-0.0811223818042267,
-10.1259737536749));
#68973=CARTESIAN_POINT('Ctrl Pts',(0.709491335059612,0.430501765787835,
-10.1047916223491));
#68974=CARTESIAN_POINT('Ctrl Pts',(0.158892812090172,0.876879595249961,
-10.0783139581917));
#68975=CARTESIAN_POINT('Ctrl Pts',(-0.652350196007727,0.606154465232593,
-10.046540761203));
#68976=CARTESIAN_POINT('Ctrl Pts',(-0.826098981874427,-0.0793381278659279,
-10.0200630970456));
#68977=CARTESIAN_POINT('Ctrl Pts',(-0.574937634292116,-0.532760589737299,
-9.99888096571977));
#68978=CARTESIAN_POINT('Ctrl Pts',(-0.250625132038328,-0.744451925502288,
-9.98299436722538));
#68979=CARTESIAN_POINT('Ctrl Pts',(0.134890381171093,-0.772134485564218,
-9.96710776873098));
#68980=CARTESIAN_POINT('Ctrl Pts',(0.610587288138713,-0.56273691931158,
-9.94592563740513));
#68981=CARTESIAN_POINT('Ctrl Pts',(0.829446527249074,-0.0430310470718053,
-9.92474350607925));
#68982=CARTESIAN_POINT('Ctrl Pts',(0.646129213264504,0.442344518851281,
-9.90356137475341));
#68983=CARTESIAN_POINT('Ctrl Pts',(0.262081418700829,0.787415427104953,
-9.88237924342756));
#68984=CARTESIAN_POINT('Ctrl Pts',(-0.446543488446261,0.771209221434691,
-9.85590157927021));
#68985=CARTESIAN_POINT('Ctrl Pts',(-0.889610890178794,0.0397048867020595,
-9.82412838228145));
#68986=CARTESIAN_POINT('Ctrl Pts',(-0.578285328073375,-0.595247969943875,
-9.7976507181241));
#68987=CARTESIAN_POINT('Ctrl Pts',(-0.0933283262204505,-0.778252499403336,
-9.77646858679826));
#68988=CARTESIAN_POINT('Ctrl Pts',(0.29089858374514,-0.729657207302419,
-9.76058198830386));
#68989=CARTESIAN_POINT('Ctrl Pts',(0.60265533980172,-0.501192198800497,
-9.74469538980948));
#68990=CARTESIAN_POINT('Ctrl Pts',(0.829673131787345,-0.0336477515304431,
-9.72351325848361));
#68991=CARTESIAN_POINT('Ctrl Pts',(0.660052778303402,0.504146350211528,
-9.70233112715774));
#68992=CARTESIAN_POINT('Ctrl Pts',(0.206120956474527,0.755424241663983,
-9.6811489958319));
#68993=CARTESIAN_POINT('Ctrl Pts',(-0.309979234121676,0.769819848590857,
-9.65996686450603));
#68994=CARTESIAN_POINT('Ctrl Pts',(-0.839595504076748,0.298737576869337,
-9.63348920034872));
#68995=CARTESIAN_POINT('Ctrl Pts',(-0.703756305225402,-0.545629065215758,
-9.60171600335992));
#68996=CARTESIAN_POINT('Ctrl Pts',(-0.0554285506970736,-0.828046944414903,
-9.5752383392026));
#68997=CARTESIAN_POINT('Ctrl Pts',(0.432669647991569,-0.653593225951356,
-9.55405620787675));
#68998=CARTESIAN_POINT('Ctrl Pts',(0.694065590076106,-0.367824119472337,
-9.53816960938235));
#68999=CARTESIAN_POINT('Ctrl Pts',(0.78378634966761,0.00812630326319978,
-9.52228301088796));
#69000=CARTESIAN_POINT('Ctrl Pts',(0.65415119509764,0.511444904897103,-9.5011008795621));
#69001=CARTESIAN_POINT('Ctrl Pts',(0.176725804605299,0.811542483523972,
-9.47991874823624));
#69002=CARTESIAN_POINT('Ctrl Pts',(-0.331922213101395,0.709210320033098,
-9.45873661691039));
#69003=CARTESIAN_POINT('Ctrl Pts',(-0.734608069712466,0.386083810570246,
-9.43755448558453));
#69004=CARTESIAN_POINT('Ctrl Pts',(-0.833320476860817,-0.315819146259562,
-9.4110768214272));
#69005=CARTESIAN_POINT('Ctrl Pts',(-0.183182295399402,-0.871451811980982,
-9.37930362443841));
#69006=CARTESIAN_POINT('Ctrl Pts',(0.493791063463925,-0.667011583130608,
-9.35282596028109));
#69007=CARTESIAN_POINT('Ctrl Pts',(0.752881990642999,-0.218073009490135,
-9.33164382895524));
#69008=CARTESIAN_POINT('Ctrl Pts',(0.76712225365182,0.168952875516953,-9.31575723046083));
#69009=CARTESIAN_POINT('Ctrl Pts',(0.592134175587876,0.513579786236636,
-9.29987063196645));
#69010=CARTESIAN_POINT('Ctrl Pts',(0.167502935024326,0.81328497069054,-9.27868850064059));
#69011=CARTESIAN_POINT('Ctrl Pts',(-0.39065520774003,0.732954105823305,
-9.25750636931472));
#69012=CARTESIAN_POINT('Ctrl Pts',(-0.712097081609459,0.325682943911511,
-9.23632423798888));
#69013=CARTESIAN_POINT('Ctrl Pts',(-0.809843814576814,-0.181280779077073,
-9.21514210666301));
#69014=CARTESIAN_POINT('Ctrl Pts',(-0.430702924997686,-0.780166482680521,
-9.18866444250569));
#69015=CARTESIAN_POINT('Ctrl Pts',(0.424516578683828,-0.782796070745956,
-9.15689124551691));
#69016=CARTESIAN_POINT('Ctrl Pts',(0.808154578229917,-0.188733261703544,
-9.13041358135957));
#69017=CARTESIAN_POINT('Ctrl Pts',(0.715009830130715,0.321166735698292,
-9.10923145003374));
#69018=CARTESIAN_POINT('Ctrl Pts',(0.475321483421555,0.625372779701216,
-9.09334485153931));
#69019=CARTESIAN_POINT('Ctrl Pts',(0.118852111688952,0.77476528979884,-9.07745825304495));
#69020=CARTESIAN_POINT('Ctrl Pts',(-0.39881279752422,0.728311766569634,
-9.05627612171906));
#69021=CARTESIAN_POINT('Ctrl Pts',(-0.772233428000458,0.305759293000729,
-9.03509399039322));
#69022=CARTESIAN_POINT('Ctrl Pts',(-0.753585498799065,-0.21274522225268,
-9.01391185906737));
#69023=CARTESIAN_POINT('Ctrl Pts',(-0.499902966579275,-0.662424900555796,
-8.99272972774149));
#69024=CARTESIAN_POINT('Ctrl Pts',(0.176764848846763,-0.873452310382106,
-8.96625206358418));
#69025=CARTESIAN_POINT('Ctrl Pts',(0.830307570719126,-0.321828140409187,
-8.93447886659539));
#69026=CARTESIAN_POINT('Ctrl Pts',(0.738144931967327,0.379310065511296,
-8.90800120243806));
#69027=CARTESIAN_POINT('Ctrl Pts',(0.33706586160392,0.707653682420898,-8.88681907111222));
#69028=CARTESIAN_POINT('Ctrl Pts',(-0.0425509146991354,0.784353903446371,
-8.87093247261781));
#69029=CARTESIAN_POINT('Ctrl Pts',(-0.410958199522342,0.667458191181559,
-8.85504587412343));
#69030=CARTESIAN_POINT('Ctrl Pts',(-0.775445838453558,0.29694010914313,
-8.83386374279756));
#69031=CARTESIAN_POINT('Ctrl Pts',(-0.786523246056195,-0.26686025554749,
-8.81268161147171));
#69032=CARTESIAN_POINT('Ctrl Pts',(-0.436654811424381,-0.6499878531569,
-8.79149948014584));
#69033=CARTESIAN_POINT('Ctrl Pts',(0.047800914194124,-0.82850757236933,
-8.77031734881999));
#69034=CARTESIAN_POINT('Ctrl Pts',(0.700160013885623,-0.551308176300101,
-8.74383968466266));
#69035=CARTESIAN_POINT('Ctrl Pts',(0.841189031607181,0.292207164622127,
-8.71206648767388));
#69036=CARTESIAN_POINT('Ctrl Pts',(0.317059998327239,0.766946558664921,
-8.68558882351655));
#69037=CARTESIAN_POINT('Ctrl Pts',(-0.201192821693523,0.757567540092399,
-8.6644066921907));
#69038=CARTESIAN_POINT('Ctrl Pts',(-0.540185316243243,0.570281904244278,
-8.6485200936963));
#69039=CARTESIAN_POINT('Ctrl Pts',(-0.745309242845801,0.242695717429499,
-8.63263349520192));
#69040=CARTESIAN_POINT('Ctrl Pts',(-0.783262595763387,-0.275661718181675,
-8.61145136387603));
#69041=CARTESIAN_POINT('Ctrl Pts',(-0.426728161974488,-0.71255616505334,
-8.5902692325502));
#69042=CARTESIAN_POINT('Ctrl Pts',(0.0879569244362535,-0.778084322573904,
-8.56908710122433));
#69043=CARTESIAN_POINT('Ctrl Pts',(0.572769802202764,-0.600536825311924,
-8.54790496989848));
#69044=CARTESIAN_POINT('Ctrl Pts',(0.890546216267256,0.0330482524761829,
-8.52142730574115));
#69045=CARTESIAN_POINT('Ctrl Pts',(0.451985538686537,0.767263375100736,
-8.48965410875238));
#69046=CARTESIAN_POINT('Ctrl Pts',(-0.254824494055272,0.789809181775388,
-8.46317644459503));
#69047=CARTESIAN_POINT('Ctrl Pts',(-0.643760503623392,0.447168361221148,
-8.44199431326919));
#69048=CARTESIAN_POINT('Ctrl Pts',(-0.780897659633066,0.0849733568413833,
-8.42610771477479));
#69049=CARTESIAN_POINT('Ctrl Pts',(-0.725177520948885,-0.297497297198533,
-8.41022111628039));
#69050=CARTESIAN_POINT('Ctrl Pts',(-0.418545276104388,-0.717153769176163,
-8.38903898495455));
#69051=CARTESIAN_POINT('Ctrl Pts',(0.136026673789023,-0.819347274722716,
-8.36785685362867));
#69052=CARTESIAN_POINT('Ctrl Pts',(0.570734731503279,-0.536109596861927,
-8.34667472230283));
#69053=CARTESIAN_POINT('Ctrl Pts',(0.825318852045567,-0.0869397338925285,
-8.32549259097696));
#69054=CARTESIAN_POINT('Ctrl Pts',(0.657372281257338,0.601686325367446,
-8.29901492681965));
#69055=CARTESIAN_POINT('Ctrl Pts',(-0.15219057819013,0.877395031820266,
-8.26724172983084));
#69056=CARTESIAN_POINT('Ctrl Pts',(-0.705509776625659,0.437024051366566,
-8.24076406567354));
#69057=CARTESIAN_POINT('Ctrl Pts',(-0.780143865883835,-0.0759123035250102,
-8.21958193434766));
#69058=CARTESIAN_POINT('Ctrl Pts',(-0.650200733115148,-0.440750079806934,
-8.20369533585329));
#69059=CARTESIAN_POINT('Ctrl Pts',(-0.360138050531249,-0.696195133055061,
-8.18780873735887));
#69060=CARTESIAN_POINT('Ctrl Pts',(0.145239864419022,-0.817554315367743,
-8.16662660603304));
#69061=CARTESIAN_POINT('Ctrl Pts',(0.634084725054934,-0.536441771331854,
-8.14544447470716));
#69062=CARTESIAN_POINT('Ctrl Pts',(0.782060617407885,-0.0391512999934004,
-8.12426234338132));
#69063=CARTESIAN_POINT('Ctrl Pts',(0.685331096971596,0.468007491814848,
-8.10308021205544));
#69064=CARTESIAN_POINT('Ctrl Pts',(0.111540015123584,0.8841513305571,-8.07660254789814));
#69065=CARTESIAN_POINT('Ctrl Pts',(-0.683982060748652,0.570221496023044,
-8.04482935090934));
#69066=CARTESIAN_POINT('Ctrl Pts',(-0.820641651118927,-0.123617744826675,
-8.01835168675202));
#69067=CARTESIAN_POINT('Ctrl Pts',(-0.545476476388819,-0.562887682410165,
-7.99716955542616));
#69068=CARTESIAN_POINT('Ctrl Pts',(-0.210256395491838,-0.756844683107489,
-7.98128295693177));
#69069=CARTESIAN_POINT('Ctrl Pts',(0.176189691484825,-0.763769776401557,
-7.96539635843737));
#69070=CARTESIAN_POINT('Ctrl Pts',(0.639946257759712,-0.529111012900144,
-7.94421422711152));
#69071=CARTESIAN_POINT('Ctrl Pts',(0.830560434656543,0.00160529149460393,
-7.92303209578566));
#69072=CARTESIAN_POINT('Ctrl Pts',(0.621424109326631,0.476428074255893,
-7.90184996445979));
#69073=CARTESIAN_POINT('Ctrl Pts',(0.219387284491965,0.800361758378271,
-7.88066783313394));
#69074=CARTESIAN_POINT('Ctrl Pts',(-0.487342730892537,0.746097723455757,
-7.85419016897662));
#69075=CARTESIAN_POINT('Ctrl Pts',(-0.890459112307306,-0.00815985671544194,
-7.82241697198783));
#69076=CARTESIAN_POINT('Ctrl Pts',(-0.545461283363713,-0.625464671055404,
-7.7959393078305));
#69077=CARTESIAN_POINT('Ctrl Pts',(-0.0513704557899223,-0.78214334081074,
-7.77475717650466));
#69078=CARTESIAN_POINT('Ctrl Pts',(0.329689745670944,-0.712970053924232,
-7.75887057801024));
#69079=CARTESIAN_POINT('Ctrl Pts',(0.628718380100739,-0.468081485698276,
-7.74298397951587));
#69080=CARTESIAN_POINT('Ctrl Pts',(0.830282456821142,0.0109872056466471,
-7.72180184818998));
#69081=CARTESIAN_POINT('Ctrl Pts',(0.632006346377846,0.538888848201348,
-7.70061971686417));
#69082=CARTESIAN_POINT('Ctrl Pts',(0.165226880962859,0.765409505688858,
-7.67943758553827));
#69083=CARTESIAN_POINT('Ctrl Pts',(-0.350901150045432,0.752049272167661,
-7.65825545421243));
#69084=CARTESIAN_POINT('Ctrl Pts',(-0.854436322923102,0.253186335273663,
-7.6317777900551));
#69085=CARTESIAN_POINT('Ctrl Pts',(-0.673417454717608,-0.582660231725479,
-7.60000459306631));
#69086=CARTESIAN_POINT('Ctrl Pts',(-0.010849510586414,-0.829829111629177,
-7.573526928909));
#69087=CARTESIAN_POINT('Ctrl Pts',(0.467168297119543,-0.629397260455649,
-7.55234479758313));
#69088=CARTESIAN_POINT('Ctrl Pts',(0.712829388280181,-0.329993771755461,
-7.53645819908875));
#69089=CARTESIAN_POINT('Ctrl Pts',(0.782217059277867,0.050234956998986,
-7.52057160059434));
#69090=CARTESIAN_POINT('Ctrl Pts',(0.625721069366487,0.545859707382523,
-7.49938946926849));
#69091=CARTESIAN_POINT('Ctrl Pts',(0.132858431507887,0.819866970767157,
-7.47820733794263));
#69092=CARTESIAN_POINT('Ctrl Pts',(-0.36955528675953,0.690348117705594,
-7.45702520661678));
#69093=CARTESIAN_POINT('Ctrl Pts',(-0.754294552512423,0.346048338995004,
-7.4358430752909));
#69094=CARTESIAN_POINT('Ctrl Pts',(-0.815144306078038,-0.36014512431548,
-7.4093654111336));
#69095=CARTESIAN_POINT('Ctrl Pts',(-0.136086086799767,-0.880036698628102,
-7.3775922141448));
#69096=CARTESIAN_POINT('Ctrl Pts',(0.528922488702051,-0.6395115849869,-7.35111454998748));
#69097=CARTESIAN_POINT('Ctrl Pts',(0.763513227295881,-0.177298282695796,
-7.32993241866162));
#69098=CARTESIAN_POINT('Ctrl Pts',(0.75693428106787,0.209933609356769,-7.31404582016723));
#69099=CARTESIAN_POINT('Ctrl Pts',(0.563678937842369,0.544658731466687,
-7.29815922167283));
#69100=CARTESIAN_POINT('Ctrl Pts',(0.123555248510802,0.821111306314991,
-7.27697709034699));
#69101=CARTESIAN_POINT('Ctrl Pts',(-0.429479393638669,0.710901303288584,
-7.25579495902111));
#69102=CARTESIAN_POINT('Ctrl Pts',(-0.728570172364044,0.286944485106448,
-7.23461282769527));
#69103=CARTESIAN_POINT('Ctrl Pts',(-0.798931611445651,-0.22453954017939,
-7.2134306963694));
#69104=CARTESIAN_POINT('Ctrl Pts',(-0.388154685257379,-0.802184947884465,
-7.18695303221208));
#69105=CARTESIAN_POINT('Ctrl Pts',(0.465970323534831,-0.758851547759888,
-7.15517983522329));
#69106=CARTESIAN_POINT('Ctrl Pts',(0.817129237482638,-0.145030602419892,
-7.12870217106598));
#69107=CARTESIAN_POINT('Ctrl Pts',(0.696717242889235,0.359127014806003,
-7.1075200397401));
#69108=CARTESIAN_POINT('Ctrl Pts',(0.441027326936127,0.650012709944097,
-7.09163344124572));
#69109=CARTESIAN_POINT('Ctrl Pts',(0.0770447603055038,0.780032809335269,
-7.07574684275133));
#69110=CARTESIAN_POINT('Ctrl Pts',(-0.437375717913696,0.70582728636144,
-7.05456471142546));
#69111=CARTESIAN_POINT('Ctrl Pts',(-0.78754893079125,0.263817918624197,
-7.03338258009962));
#69112=CARTESIAN_POINT('Ctrl Pts',(-0.741063702120943,-0.252935215006503,
-7.01220044877374));
#69113=CARTESIAN_POINT('Ctrl Pts',(-0.46358212175395,-0.688332289858035,
-6.99101831744789));
#69114=CARTESIAN_POINT('Ctrl Pts',(0.223448433227565,-0.862690876263233,
-6.96454065329057));
#69115=CARTESIAN_POINT('Ctrl Pts',(0.846402689376789,-0.276742662718453,
-6.93276745630178));
#69116=CARTESIAN_POINT('Ctrl Pts',(0.716694312453694,0.418429598479429,
-6.90628979214446));
#69117=CARTESIAN_POINT('Ctrl Pts',(0.298549740945737,0.724744907870361,
-6.88510766081859));
#69118=CARTESIAN_POINT('Ctrl Pts',(-0.0846403243704471,0.780933826699518,
-6.86922106232421));
#69119=CARTESIAN_POINT('Ctrl Pts',(-0.446233320337088,0.644408955982971,
-6.85333446382981));
#69120=CARTESIAN_POINT('Ctrl Pts',(-0.790282759485384,0.254838844868011,
-6.83215233250395));
#69121=CARTESIAN_POINT('Ctrl Pts',(-0.771045731306174,-0.308742113761099,
-6.8109702011781));
#69122=CARTESIAN_POINT('Ctrl Pts',(-0.401093723806668,-0.672514281125272,
-6.78978806985224));
#69123=CARTESIAN_POINT('Ctrl Pts',(0.0922555398017252,-0.824741559667119,
-6.76860593852637));
#69124=CARTESIAN_POINT('Ctrl Pts',(0.728775372717111,-0.512885178590886,
-6.74212827436905));
#69125=CARTESIAN_POINT('Ctrl Pts',(0.82427039002562,0.336990115741366,-6.71035507738027));
#69126=CARTESIAN_POINT('Ctrl Pts',(0.275386408658267,0.782876996896595,
-6.68387741322294));
#69127=CARTESIAN_POINT('Ctrl Pts',(-0.241613501318641,0.745660811168969,
-6.66269528189708));
#69128=CARTESIAN_POINT('Ctrl Pts',(-0.57005148285138,0.540428471763071,
-6.6468086834027));
#69129=CARTESIAN_POINT('Ctrl Pts',(-0.75727463761217,0.202292367226153,
-6.63092208490829));
#69130=CARTESIAN_POINT('Ctrl Pts',(-0.767316805534387,-0.317355632215704,
-6.60973995358245));
#69131=CARTESIAN_POINT('Ctrl Pts',(-0.387819019492267,-0.734458725566816,
-6.58855782225657));
#69132=CARTESIAN_POINT('Ctrl Pts',(0.129643795992169,-0.772233203466112,
-6.56737569093074));
#69133=CARTESIAN_POINT('Ctrl Pts',(0.60421477347276,-0.568888594012783,
-6.54619355960485));
#69134=CARTESIAN_POINT('Ctrl Pts',(0.887483356468985,0.0808581273468804,
-6.51971589544755));
#69135=CARTESIAN_POINT('Ctrl Pts',(0.410099958547019,0.79044421082833,-6.48794269845874));
#69136=CARTESIAN_POINT('Ctrl Pts',(-0.296900337661013,0.774973707316207,
-6.46146503430144));
#69137=CARTESIAN_POINT('Ctrl Pts',(-0.666860912852976,0.411926749263547,
-6.44028290297557));
#69138=CARTESIAN_POINT('Ctrl Pts',(-0.784335711330281,0.0428853824613141,
-6.42439630448119));
#69139=CARTESIAN_POINT('Ctrl Pts',(-0.708142180514372,-0.336038136658672,
-6.40850970598678));
#69140=CARTESIAN_POINT('Ctrl Pts',(-0.379400994004317,-0.73861005639688,
-6.38732757466094));
#69141=CARTESIAN_POINT('Ctrl Pts',(0.179861749568897,-0.810853057436283,
-6.36614544333507));
#69142=CARTESIAN_POINT('Ctrl Pts',(0.598720101579247,-0.504664087636979,
-6.34496331200921));
#69143=CARTESIAN_POINT('Ctrl Pts',(0.828798932842316,-0.0424611625032776,
-6.32378118068336));
#69144=CARTESIAN_POINT('Ctrl Pts',(0.624086742236349,0.636142542035344,
-6.29730351652602));
#69145=CARTESIAN_POINT('Ctrl Pts',(-0.199119407007607,0.867950779039128,
-6.26553031953726));
#69146=CARTESIAN_POINT('Ctrl Pts',(-0.72797945196655,0.39847486417064,-6.23905265537991));
#69147=CARTESIAN_POINT('Ctrl Pts',(-0.774932010702059,-0.117721945292821,
-6.21787052405407));
#69148=CARTESIAN_POINT('Ctrl Pts',(-0.625586409139169,-0.4750663333995,
-6.20198392555967));
#69149=CARTESIAN_POINT('Ctrl Pts',(-0.322183903833611,-0.714521199467751,
-6.18609732706528));
#69150=CARTESIAN_POINT('Ctrl Pts',(0.18891837154225,-0.808617098475062,
-6.16491519573941));
#69151=CARTESIAN_POINT('Ctrl Pts',(0.662086178303616,-0.501496584144044,
-6.14373306441357));
#69152=CARTESIAN_POINT('Ctrl Pts',(0.782929853410714,0.00282242379590618,
-6.12255093308769));
#69153=CARTESIAN_POINT('Ctrl Pts',(0.65943455555827,0.504418815941523,-6.10136880176185));
#69154=CARTESIAN_POINT('Ctrl Pts',(0.0633494618177429,0.888321484655266,
-6.07489113760451));
#69155=CARTESIAN_POINT('Ctrl Pts',(-0.712753999556802,0.533586528221487,
-6.04311794061574));
#69156=CARTESIAN_POINT('Ctrl Pts',(-0.834426729678636,-0.309565746092443,
-6.01134474362693));
#69157=CARTESIAN_POINT('Ctrl Pts',(-0.192051279620842,-0.869031198721859,
-5.97957154663817));
#69158=CARTESIAN_POINT('Ctrl Pts',(0.626405930208662,-0.632730951971766,
-5.94779834964936));
#69159=CARTESIAN_POINT('Ctrl Pts',(0.871207376069929,0.18473202833857,-5.91602515266059));
#69160=CARTESIAN_POINT('Ctrl Pts',(0.409088109036795,0.722453592962815,
-5.88954748850325));
#69161=CARTESIAN_POINT('Ctrl Pts',(-0.104714804097165,0.775900722541678,
-5.86836535717741));
#69162=CARTESIAN_POINT('Ctrl Pts',(-0.587662362179258,0.586949639651242,
-5.84718322585153));
#69163=CARTESIAN_POINT('Ctrl Pts',(-0.826898986241856,0.076090929844471,
-5.82600109452569));
#69164=CARTESIAN_POINT('Ctrl Pts',(-0.663510831709495,-0.417248593266023,
-5.80481896319982));
#69165=CARTESIAN_POINT('Ctrl Pts',(-0.38466164816873,-0.684895461262083,
-5.78893236470544));
#69166=CARTESIAN_POINT('Ctrl Pts',(-0.0101945223770054,-0.783756434951424,
-5.77304576621103));
#69167=CARTESIAN_POINT('Ctrl Pts',(0.494664911251325,-0.666365459367492,
-5.75186363488519));
#69168=CARTESIAN_POINT('Ctrl Pts',(0.887071385837545,-0.078047738660052,
-5.72538597072785));
#69169=CARTESIAN_POINT('Ctrl Pts',(0.544417912065992,0.705528690163676,
-5.69361277373907));
#69170=CARTESIAN_POINT('Ctrl Pts',(-0.155868076444456,0.815117024817418,
-5.66713510958174));
#69171=CARTESIAN_POINT('Ctrl Pts',(-0.582098546485917,0.523748874523383,
-5.64595297825589));
#69172=CARTESIAN_POINT('Ctrl Pts',(-0.827870125232059,0.0668130635430879,
-5.62477084693002));
#69173=CARTESIAN_POINT('Ctrl Pts',(-0.679514548851711,-0.477231503110312,
-5.60358871560419));
#69174=CARTESIAN_POINT('Ctrl Pts',(-0.235614059614225,-0.747578084232534,
-5.58240658427831));
#69175=CARTESIAN_POINT('Ctrl Pts',(0.150182669760855,-0.771016750661316,
-5.56651998578392));
#69176=CARTESIAN_POINT('Ctrl Pts',(0.499596680867893,-0.60397870849536,
-5.55063338728952));
#69177=CARTESIAN_POINT('Ctrl Pts',(0.808402184679265,-0.187669830661293,
-5.52945125596367));
#69178=CARTESIAN_POINT('Ctrl Pts',(0.726642152424438,0.514757427097727,
-5.50297359180634));
#69179=CARTESIAN_POINT('Ctrl Pts',(-0.0417754286247196,0.890179509049,-5.47120039481756));
#69180=CARTESIAN_POINT('Ctrl Pts',(-0.646469171849264,0.52037230396045,
-5.44472273066023));
#69181=CARTESIAN_POINT('Ctrl Pts',(-0.782720280203898,0.022374032545029,
-5.42354059933438));
#69182=CARTESIAN_POINT('Ctrl Pts',(-0.674246595796987,-0.484999731440488,
-5.40235846800852));
#69183=CARTESIAN_POINT('Ctrl Pts',(-0.208982783747563,-0.803626700310318,
-5.38117633668266));
#69184=CARTESIAN_POINT('Ctrl Pts',(0.304363613856124,-0.722322552028555,
-5.35999420535681));
#69185=CARTESIAN_POINT('Ctrl Pts',(0.613587412181548,-0.490440734243774,
-5.3441076068624));
#69186=CARTESIAN_POINT('Ctrl Pts',(0.771775082904571,-0.136931920092647,
-5.32822100836802));
#69187=CARTESIAN_POINT('Ctrl Pts',(0.737645240287663,0.380280903838839,
-5.30703887704216));
#69188=CARTESIAN_POINT('Ctrl Pts',(0.220610507918605,0.862736934283135,
-5.28056121288483));
#69189=CARTESIAN_POINT('Ctrl Pts',(-0.608100710201375,0.651443225883695,
-5.24878801589605));
#69190=CARTESIAN_POINT('Ctrl Pts',(-0.829597137570893,-0.0218703955254784,
-5.22231035173872));
#69191=CARTESIAN_POINT('Ctrl Pts',(-0.611066093544301,-0.489642586909114,
-5.20112822041286));
#69192=CARTESIAN_POINT('Ctrl Pts',(-0.199938811978368,-0.80613750938647,
-5.17994608908701));
#69193=CARTESIAN_POINT('Ctrl Pts',(0.360944933020524,-0.74780240178827,
-5.15876395776115));
#69194=CARTESIAN_POINT('Ctrl Pts',(0.699580405510616,-0.353517092876322,
-5.13758182643528));
#69195=CARTESIAN_POINT('Ctrl Pts',(0.785158688205617,0.0233978744402808,
-5.12169522794091));
#69196=CARTESIAN_POINT('Ctrl Pts',(0.676883090725284,0.395242217877812,
-5.10580862944649));
#69197=CARTESIAN_POINT('Ctrl Pts',(0.316050663373499,0.767363046131555,
-5.08462649812065));
#69198=CARTESIAN_POINT('Ctrl Pts',(-0.390347541635626,0.800382915042411,
-5.05814883396331));
#69199=CARTESIAN_POINT('Ctrl Pts',(-0.885202127408502,0.102868576013952,
-5.02637563697454));
#69200=CARTESIAN_POINT('Ctrl Pts',(-0.618153465990248,-0.553711131688124,
-4.9998979728172));
#69201=CARTESIAN_POINT('Ctrl Pts',(-0.148777649674118,-0.768776199260246,
-4.97871584149136));
#69202=CARTESIAN_POINT('Ctrl Pts',(0.369463543596736,-0.743861480741264,
-4.95753371016549));
#69203=CARTESIAN_POINT('Ctrl Pts',(0.759200609827415,-0.336309546148421,
-4.93635157883964));
#69204=CARTESIAN_POINT('Ctrl Pts',(0.762063906997977,0.183427588930845,
-4.91516944751377));
#69205=CARTESIAN_POINT('Ctrl Pts',(0.58329407081499,0.526108024216862,-4.89928284901939));
#69206=CARTESIAN_POINT('Ctrl Pts',(0.260053068103058,0.739431897521899,
-4.88339625052499));
#69207=CARTESIAN_POINT('Ctrl Pts',(-0.255863414058302,0.789473229269786,
-4.86221411919913));
#69208=CARTESIAN_POINT('Ctrl Pts',(-0.815649130744606,0.357352080542846,
-4.83573645504181));
#69209=CARTESIAN_POINT('Ctrl Pts',(-0.741285154047814,-0.494632258034153,
-4.80396325805302));
#69210=CARTESIAN_POINT('Ctrl Pts',(-0.112704652167952,-0.822196683434577,
-4.7774855938957));
#69211=CARTESIAN_POINT('Ctrl Pts',(0.384272177024485,-0.682265730897016,
-4.75630346256984));
#69212=CARTESIAN_POINT('Ctrl Pts',(0.763142251788303,-0.327791269122783,
-4.73512133124398));
#69213=CARTESIAN_POINT('Ctrl Pts',(0.796366532129932,0.23513830673929,-4.71393919991812));
#69214=CARTESIAN_POINT('Ctrl Pts',(0.462095817256364,0.633130740372142,
-4.69275706859227));
#69215=CARTESIAN_POINT('Ctrl Pts',(0.104004079803942,0.778591534488675,
-4.67687047009787));
#69216=CARTESIAN_POINT('Ctrl Pts',(-0.280462970183203,0.731934185332714,
-4.66098387160347));
#69217=CARTESIAN_POINT('Ctrl Pts',(-0.706084152242396,0.436095444070873,
-4.63980174027762));
#69218=CARTESIAN_POINT('Ctrl Pts',(-0.853013011994254,-0.255641967057878,
-4.61332407612029));
#69219=CARTESIAN_POINT('Ctrl Pts',(-0.244799346010742,-0.856876905099193,
-4.58155087913152));
#69220=CARTESIAN_POINT('Ctrl Pts',(0.446348564306262,-0.69963039100146,
-4.55507321497417));
#69221=CARTESIAN_POINT('Ctrl Pts',(0.734555098285578,-0.271257149535717,
-4.53389108364833));
#69222=CARTESIAN_POINT('Ctrl Pts',(0.793856488162095,0.24418249073304,-4.51270895232246));
#69223=CARTESIAN_POINT('Ctrl Pts',(0.454765904643669,0.694750062084561,
-4.49152682099662));
#69224=CARTESIAN_POINT('Ctrl Pts',(-0.0576535306276524,0.781705282786401,
-4.47034468967075));
#69225=CARTESIAN_POINT('Ctrl Pts',(-0.42475216183662,0.660762610328711,
-4.45445809117636));
#69226=CARTESIAN_POINT('Ctrl Pts',(-0.687585668501137,0.376315130940137,
-4.43857149268196));
#69227=CARTESIAN_POINT('Ctrl Pts',(-0.820478298756319,-0.124697344226614,
-4.41738936135611));
#69228=CARTESIAN_POINT('Ctrl Pts',(-0.484668237188422,-0.74704799967164,
-4.39091169719878));
#69229=CARTESIAN_POINT('Ctrl Pts',(0.368117527293529,-0.811575157578735,
-4.35913850020999));
#69230=CARTESIAN_POINT('Ctrl Pts',(0.793110205375747,-0.244307034282585,
-4.33266083605267));
#69231=CARTESIAN_POINT('Ctrl Pts',(0.735470123003793,0.268766314407819,
-4.31147870472682));
#69232=CARTESIAN_POINT('Ctrl Pts',(0.446997997760977,0.700018573021691,
-4.29029657340095));
#69233=CARTESIAN_POINT('Ctrl Pts',(-0.103129739915628,0.823925927215433,
-4.2691144420751));
#69234=CARTESIAN_POINT('Ctrl Pts',(-0.549981800405103,0.558486434887335,
-4.24793231074924));
#69235=CARTESIAN_POINT('Ctrl Pts',(-0.751488473754749,0.228662852267375,
-4.23204571225485));
#69236=CARTESIAN_POINT('Ctrl Pts',(-0.76767999378356,-0.158286311622709,
-4.21615911376045));
#69237=CARTESIAN_POINT('Ctrl Pts',(-0.544637896405776,-0.626181785255629,
-4.19497698243459));
#69238=CARTESIAN_POINT('Ctrl Pts',(0.114193653274018,-0.883144282382366,
-4.16849931827727));
#69239=CARTESIAN_POINT('Ctrl Pts',(0.805950943289732,-0.380273358664594,
-4.13672612128849));
#69240=CARTESIAN_POINT('Ctrl Pts',(0.762654065470712,0.327213235203154,
-4.11024845713116));
#69241=CARTESIAN_POINT('Ctrl Pts',(0.386582048616603,0.680959582705881,
-4.0890663258053));
#69242=CARTESIAN_POINT('Ctrl Pts',(-0.112460950524283,0.822912964525908,
-4.06788419447944));
#69243=CARTESIAN_POINT('Ctrl Pts',(-0.611974985955589,0.561227488063028,
-4.04670206315359));
#69244=CARTESIAN_POINT('Ctrl Pts',(-0.780728624225886,0.0696411806645941,
-4.02551993182773));
#69245=CARTESIAN_POINT('Ctrl Pts',(-0.720803064736381,-0.312193158252911,
-4.00963333333333));
#69246=CARTESIAN_POINT('Ctrl Pts',(-0.482651613809183,-0.61760387708469,
-3.99374673483894));
#69247=CARTESIAN_POINT('Ctrl Pts',(-0.00975770699374649,-0.829842667944631,
-3.97256460351309));
#69248=CARTESIAN_POINT('Ctrl Pts',(0.658742944809585,-0.599200923410776,
-3.94608693935576));
#69249=CARTESIAN_POINT('Ctrl Pts',(0.860459287509756,0.231893434227583,
-3.91431374236698));
#69250=CARTESIAN_POINT('Ctrl Pts',(0.369465644127221,0.743104880000642,
-3.88783607820964));
#69251=CARTESIAN_POINT('Ctrl Pts',(-0.146171548563407,0.769275966075993,
-3.8666539468838));
#69252=CARTESIAN_POINT('Ctrl Pts',(-0.618431405135488,0.554414835407384,
-3.84547181555793));
#69253=CARTESIAN_POINT('Ctrl Pts',(-0.829753688343227,0.0315989473508514,
-3.82428968423208));
#69254=CARTESIAN_POINT('Ctrl Pts',(-0.640146574483296,-0.452326698203083,
-3.80310755290621));
#69255=CARTESIAN_POINT('Ctrl Pts',(-0.347290478918943,-0.704564368560852,
-3.78722095441182));
#69256=CARTESIAN_POINT('Ctrl Pts',(0.0319347387027416,-0.7831776948858,
-3.77133435591742));
#69257=CARTESIAN_POINT('Ctrl Pts',(0.529763427087315,-0.638815135784943,
-3.75015222459158));
#69258=CARTESIAN_POINT('Ctrl Pts',(0.88998199246047,-0.0302665995583043,
-3.72367456043424));
#69259=CARTESIAN_POINT('Ctrl Pts',(0.505717390271106,0.733767450543454,
-3.69190136344546));
#69260=CARTESIAN_POINT('Ctrl Pts',(-0.199447423651738,0.805562195035123,
-3.66542369928813));
#69261=CARTESIAN_POINT('Ctrl Pts',(-0.609403272469123,0.491710570453291,
-3.64424156796228));
#69262=CARTESIAN_POINT('Ctrl Pts',(-0.830264524545408,0.0222268274621526,
-3.62305943663642));
#69263=CARTESIAN_POINT('Ctrl Pts',(-0.652886296214935,-0.513058633108947,
-3.60187730531056));
#69264=CARTESIAN_POINT('Ctrl Pts',(-0.19509905614842,-0.759159691382518,
-3.58069517398471));
#69265=CARTESIAN_POINT('Ctrl Pts',(0.191399837462849,-0.761831824231885,
-3.5648085754903));
#69266=CARTESIAN_POINT('Ctrl Pts',(0.5313323429325,-0.576257816134853,-3.54892197699592));
#69267=CARTESIAN_POINT('Ctrl Pts',(0.817319344918664,-0.143955391732878,
-3.52773984567005));
#69268=CARTESIAN_POINT('Ctrl Pts',(0.697929257925564,0.553063074959991,
-3.50126218151273));
#69269=CARTESIAN_POINT('Ctrl Pts',(-0.0895529864465379,0.886648190049562,
-3.46948898452395));
#69270=CARTESIAN_POINT('Ctrl Pts',(-0.673499633430044,0.484879334103558,
-3.44301132036662));
#69271=CARTESIAN_POINT('Ctrl Pts',(-0.782791606892125,-0.0197214038754891,
-3.42182918904077));
#69272=CARTESIAN_POINT('Ctrl Pts',(-0.647208586358955,-0.520532667870995,
-3.4006470577149));
#69273=CARTESIAN_POINT('Ctrl Pts',(-0.165494189844444,-0.813696104157199,
-3.37946492638905));
#69274=CARTESIAN_POINT('Ctrl Pts',(0.342741156734687,-0.704922391622064,
-3.35828279506319));
#69275=CARTESIAN_POINT('Ctrl Pts',(0.639056875647929,-0.45675807150001,
-3.3423961965688));
#69276=CARTESIAN_POINT('Ctrl Pts',(0.778018525719848,-0.0952591357265069,
-3.3265095980744));
#69277=CARTESIAN_POINT('Ctrl Pts',(0.716143170352185,0.419372180700096,
-3.30532746674855));
#69278=CARTESIAN_POINT('Ctrl Pts',(0.173928549241014,0.873345792748581,
-3.27884980259121));
#69279=CARTESIAN_POINT('Ctrl Pts',(-0.642230317963104,0.617822765029477,
-3.24707660560244));
#69280=CARTESIAN_POINT('Ctrl Pts',(-0.827223047175183,-0.0664210440547759,
-3.22059894144511));
#69281=CARTESIAN_POINT('Ctrl Pts',(-0.583869875304254,-0.521773516292051,
-3.19941681011925));
#69282=CARTESIAN_POINT('Ctrl Pts',(-0.15632835702201,-0.815717265581917,
-3.17823467879339));
#69283=CARTESIAN_POINT('Ctrl Pts',(0.400609992898513,-0.727324762662962,
-3.15705254746754));
#69284=CARTESIAN_POINT('Ctrl Pts',(0.717567380243094,-0.315411054880874,
-3.13587041614168));
#69285=CARTESIAN_POINT('Ctrl Pts',(0.782766726021657,0.0655582094525445,
-3.11998381764728));
#69286=CARTESIAN_POINT('Ctrl Pts',(0.6546648075705,0.431046539287036,-3.10409721915289));
#69287=CARTESIAN_POINT('Ctrl Pts',(0.274356150345474,0.783238641254918,
-3.08291508782703));
#69288=CARTESIAN_POINT('Ctrl Pts',(-0.432795772061448,0.778249210496526,
-3.05643742366971));
#69289=CARTESIAN_POINT('Ctrl Pts',(-0.889451114215646,0.055149485221593,
-3.02466422668093));
#69290=CARTESIAN_POINT('Ctrl Pts',(-0.58750398582496,-0.586130353684993,
-2.99818656252359));
#69291=CARTESIAN_POINT('Ctrl Pts',(-0.107248906905033,-0.775660560786259,
-2.97700443119775));
#69292=CARTESIAN_POINT('Ctrl Pts',(0.408904510245349,-0.722931749253457,
-2.95582229987188));
#69293=CARTESIAN_POINT('Ctrl Pts',(0.776176704892586,-0.295024405049747,
-2.93464016854603));
#69294=CARTESIAN_POINT('Ctrl Pts',(0.751105377928227,0.224115572812998,
-2.91345803722016));
#69295=CARTESIAN_POINT('Ctrl Pts',(0.554178344183514,0.556693801861776,
-2.89757143872578));
#69296=CARTESIAN_POINT('Ctrl Pts',(0.219940482511759,0.752338563051997,
-2.88168484023137));
#69297=CARTESIAN_POINT('Ctrl Pts',(-0.297919693948934,0.774582418045106,
-2.86050270890553));
#69298=CARTESIAN_POINT('Ctrl Pts',(-0.833674474879105,0.313003009390929,
-2.83402504474819));
#69299=CARTESIAN_POINT('Ctrl Pts',(-0.71363262372644,-0.533753902705133,
-2.80225184775942));
#69300=CARTESIAN_POINT('Ctrl Pts',(-0.0683572379509413,-0.827065301467073,
-2.77577418360209));
#69301=CARTESIAN_POINT('Ctrl Pts',(0.420381611491688,-0.660629195775685,
-2.75459205227623));
#69302=CARTESIAN_POINT('Ctrl Pts',(0.779654881965752,-0.286306614671439,
-2.73340992095037));
#69303=CARTESIAN_POINT('Ctrl Pts',(0.78257951976473,0.27759497840861,-2.71222778962451));
#69304=CARTESIAN_POINT('Ctrl Pts',(0.427403862088424,0.657048717677694,
-2.69104565829866));
#69305=CARTESIAN_POINT('Ctrl Pts',(0.0620125630885026,0.783055597140136,
-2.67515905980426));
#69306=CARTESIAN_POINT('Ctrl Pts',(-0.319391575743669,0.71580454779683,
-2.65927246130987));
#69307=CARTESIAN_POINT('Ctrl Pts',(-0.728499459819008,0.397520569820789,
-2.63809032998401));
#69308=CARTESIAN_POINT('Ctrl Pts',(-0.838042285090092,-0.301113172002998,
-2.61161266582668));
#69309=CARTESIAN_POINT('Ctrl Pts',(-0.198397349884215,-0.868794130884054,
-2.5798394688379));
#69310=CARTESIAN_POINT('Ctrl Pts',(0.483301467830881,-0.674632800909974,
-2.55336180468057));
#69311=CARTESIAN_POINT('Ctrl Pts',(0.748070914185315,-0.231390451275595,
-2.53217967335472));
#69312=CARTESIAN_POINT('Ctrl Pts',(0.779587071663486,0.286491204529554,
-2.51099754202886));
#69313=CARTESIAN_POINT('Ctrl Pts',(0.416773141159263,0.718185091463975,
-2.48981541070299));
#69314=CARTESIAN_POINT('Ctrl Pts',(-0.0995787808181823,0.777477424200066,
-2.46863327937715));
#69315=CARTESIAN_POINT('Ctrl Pts',(-0.45964753201515,0.636981767796903,
-2.45274668088275));
#69316=CARTESIAN_POINT('Ctrl Pts',(-0.706815134212639,0.338820742208353,
-2.43686008238836));
#69317=CARTESIAN_POINT('Ctrl Pts',(-0.812591502026715,-0.168609362792247,
-2.4156779510625));
#69318=CARTESIAN_POINT('Ctrl Pts',(-0.443821791933158,-0.772014398154575,
-2.38920028690517));
#69319=CARTESIAN_POINT('Ctrl Pts',(0.411199347587806,-0.790619913006889,
-2.35742708991639));
#69320=CARTESIAN_POINT('Ctrl Pts',(0.805093118566376,-0.201332549053002,
-2.33094942575906));
#69321=CARTESIAN_POINT('Ctrl Pts',(0.719963950045008,0.307901841870368,
-2.3097672944332));
#69322=CARTESIAN_POINT('Ctrl Pts',(0.408733331163781,0.723028544784651,
-2.28858516310735));
#69323=CARTESIAN_POINT('Ctrl Pts',(-0.147258198381348,0.817193183893717,
-2.26740303178149));
#69324=CARTESIAN_POINT('Ctrl Pts',(-0.579199926573699,0.528123587607129,
-2.24622090045563));
#69325=CARTESIAN_POINT('Ctrl Pts',(-0.762690818405532,0.187947710050428,
-2.23033430196123));
#69326=CARTESIAN_POINT('Ctrl Pts',(-0.758064432560231,-0.199312431598691,
-2.21444770346684));
#69327=CARTESIAN_POINT('Ctrl Pts',(-0.510200100753733,-0.654545585561551,
-2.19326557214098));
#69328=CARTESIAN_POINT('Ctrl Pts',(0.161488497277849,-0.875731396719148,
-2.16678790798366));
#69329=CARTESIAN_POINT('Ctrl Pts',(0.825222082722822,-0.336412342945777,
-2.13501471099487));
#69330=CARTESIAN_POINT('Ctrl Pts',(0.743967694720049,0.367725161070136,
-2.10853704683755));
#69331=CARTESIAN_POINT('Ctrl Pts',(0.349428907465107,0.700750363695459,
-2.08735491551169));
#69332=CARTESIAN_POINT('Ctrl Pts',(-0.156521488967608,0.815680229053644,
-2.06617278418584));
#69333=CARTESIAN_POINT('Ctrl Pts',(-0.641250834035424,0.52752918842634,
-2.04499065285997));
#69334=CARTESIAN_POINT('Ctrl Pts',(-0.783342948908494,0.0275844725406853,
-2.02380852153412));
#69335=CARTESIAN_POINT('Ctrl Pts',(-0.702984342986585,-0.350477730689136,
-2.00792192303972));
#69336=CARTESIAN_POINT('Ctrl Pts',(-0.448764363180785,-0.642648952104954,
-1.99203532454533));
#69337=CARTESIAN_POINT('Ctrl Pts',(0.0348518394390736,-0.82916790559871,
-1.97085319321947));
#69338=CARTESIAN_POINT('Ctrl Pts',(0.689991891074865,-0.562934458177559,
-1.94437552906215));
#69339=CARTESIAN_POINT('Ctrl Pts',(0.846754038208352,0.277799116408794,
-1.91260233207336));
#69340=CARTESIAN_POINT('Ctrl Pts',(0.328997570582567,0.761886030467734,
-1.88612466791604));
#69341=CARTESIAN_POINT('Ctrl Pts',(-0.187300941572847,0.76030914165062,
-1.86494253659018));
#69342=CARTESIAN_POINT('Ctrl Pts',(-0.647331814067898,0.520379414536371,
-1.84376040526432));
#69343=CARTESIAN_POINT('Ctrl Pts',(-0.830252794971939,-0.0130373783466202,
-1.82257827393846));
#69344=CARTESIAN_POINT('Ctrl Pts',(-0.614913676842763,-0.486074324318531,
-1.80139614261261));
#69345=CARTESIAN_POINT('Ctrl Pts',(-0.308925602114689,-0.722209525381228,
-1.78550954411821));
#69346=CARTESIAN_POINT('Ctrl Pts',(0.073976279919845,-0.780329827260158,
-1.76962294562382));
#69347=CARTESIAN_POINT('Ctrl Pts',(0.563327604660279,-0.609422740152469,
-1.74844081429796));
#69348=CARTESIAN_POINT('Ctrl Pts',(0.890322468184475,0.0176044482627306,
-1.72196315014064));
#69349=CARTESIAN_POINT('Ctrl Pts',(0.465554220531463,0.759884213577963,
-1.69018995315185));
#69350=CARTESIAN_POINT('Ctrl Pts',(-0.242449840923054,0.793679909981037,
-1.66371228899453));
#69351=CARTESIAN_POINT('Ctrl Pts',(-0.63494702258507,0.45825092700608,-1.64253015766867));
#69352=CARTESIAN_POINT('Ctrl Pts',(-0.83025923865599,-0.0224234075023661,
-1.62134802634281));
#69353=CARTESIAN_POINT('Ctrl Pts',(-0.624371277112666,-0.547403128516433,
-1.60016589501695));
#69354=CARTESIAN_POINT('Ctrl Pts',(-0.154020165762932,-0.768547244656021,
-1.57898376369109));
#69355=CARTESIAN_POINT('Ctrl Pts',(0.232063829254024,-0.750445204758646,
-1.5630971651967));
#69356=CARTESIAN_POINT('Ctrl Pts',(0.561532445545602,-0.546871504013718,
-1.54721056670231));
#69357=CARTESIAN_POINT('Ctrl Pts',(0.823874414294551,-0.0998249260357819,
-1.52602843537644));
#69358=CARTESIAN_POINT('Ctrl Pts',(0.667199326600337,0.589770355762977,
-1.49955077121913));
#69359=CARTESIAN_POINT('Ctrl Pts',(-0.137071735407018,0.880554421743578,
-1.46777757423034));
#69360=CARTESIAN_POINT('Ctrl Pts',(-0.698583654935227,0.447985046545584,
-1.44129991007301));
#69361=CARTESIAN_POINT('Ctrl Pts',(-0.780600637389563,-0.0617598453575331,
-1.42011777874716));
#69362=CARTESIAN_POINT('Ctrl Pts',(-0.618300119713807,-0.554561245075368,
-1.3989356474213));
#69363=CARTESIAN_POINT('Ctrl Pts',(-0.121527311840313,-0.821413896443042,
-1.37775351609544));
#69364=CARTESIAN_POINT('Ctrl Pts',(0.38012816508924,-0.685484979292683,
-1.35657138476958));
#69365=CARTESIAN_POINT('Ctrl Pts',(0.662679441042163,-0.421755361096154,
-1.34068478627519));
#69366=CARTESIAN_POINT('Ctrl Pts',(0.78201346623163,-0.053311048902077,
-1.32479818778079));
#69367=CARTESIAN_POINT('Ctrl Pts',(0.692571420136857,0.457251456418509,
-1.30361605645493));
#69368=CARTESIAN_POINT('Ctrl Pts',(0.126743930630883,0.881430649569758,
-1.27713839229761));
#69369=CARTESIAN_POINT('Ctrl Pts',(-0.674503856347413,0.582416773515433,
-1.24536519530882));
#69370=CARTESIAN_POINT('Ctrl Pts',(-0.82245825156047,-0.110779733305397,
-1.2188875311515));
#69371=CARTESIAN_POINT('Ctrl Pts',(-0.554986251520806,-0.552396500907149,
-1.19770539982564));
#69372=CARTESIAN_POINT('Ctrl Pts',(-0.112266107328216,-0.822939568694453,
-1.17652326849979));
#69373=CARTESIAN_POINT('Ctrl Pts',(0.439117275072637,-0.704745128060961,
-1.15534113717392));
#69374=CARTESIAN_POINT('Ctrl Pts',(0.733480558694665,-0.276393467265362,
-1.13415900584807));
#69375=CARTESIAN_POINT('Ctrl Pts',(0.778112539034564,0.107529078813453,
-1.11827240735367));
#69376=CARTESIAN_POINT('Ctrl Pts',(0.630554518897266,0.465605120247713,
-1.10238580885928));
#69377=CARTESIAN_POINT('Ctrl Pts',(0.231868737890888,0.796850647722728,
-1.08120367753342));
#69378=CARTESIAN_POINT('Ctrl Pts',(-0.473993206691168,0.753866336934694,
-1.0547260133761));
#69379=CARTESIAN_POINT('Ctrl Pts',(-0.891129554390263,0.00727101037626396,
-1.02295281638731));
#69380=CARTESIAN_POINT('Ctrl Pts',(-0.555156597401148,-0.616855637271071,
-0.996475152229989));
#69381=CARTESIAN_POINT('Ctrl Pts',(-0.0654102108264915,-0.78030323458971,
-0.97529302090413));
#69382=CARTESIAN_POINT('Ctrl Pts',(0.447163727728668,-0.699912718259666,
-0.954110889578273));
#69383=CARTESIAN_POINT('Ctrl Pts',(0.790909620559512,-0.252886632503504,
-0.932928758252414));
#69384=CARTESIAN_POINT('Ctrl Pts',(0.737976126523209,0.264155854396524,
-0.911746626926556));
#69385=CARTESIAN_POINT('Ctrl Pts',(0.523461021630659,0.585670713820323,
-0.895860028432162));
#69386=CARTESIAN_POINT('Ctrl Pts',(0.179192260788228,0.763070942295198,
-0.879973429937767));
#69387=CARTESIAN_POINT('Ctrl Pts',(-0.339114974901541,0.757453034972048,
-0.858791298611909));
#69388=CARTESIAN_POINT('Ctrl Pts',(-0.849290468929591,0.267749347956247,
-0.832313634454588));
#69389=CARTESIAN_POINT('Ctrl Pts',(-0.683917668721205,-0.571332978840512,
-0.800540437465799));
#69390=CARTESIAN_POINT('Ctrl Pts',(-0.0238122687778703,-0.829543670184782,
-0.774062773308478));
#69391=CARTESIAN_POINT('Ctrl Pts',(0.455276127534381,-0.637083417819315,
-0.752880641982621));
#69392=CARTESIAN_POINT('Ctrl Pts',(0.793914280715303,-0.243994523545205,
-0.731698510656761));
#69393=CARTESIAN_POINT('Ctrl Pts',(0.766530823567235,0.319249390391231,
-0.710516379330903));
#69394=CARTESIAN_POINT('Ctrl Pts',(0.391476694020716,0.67906779978643,-0.689334248005045));
#69395=CARTESIAN_POINT('Ctrl Pts',(0.0198418276109007,0.785256600327428,
-0.673447649510651));
#69396=CARTESIAN_POINT('Ctrl Pts',(-0.357397127539648,0.697606208289608,
-0.657561051016257));
#69397=CARTESIAN_POINT('Ctrl Pts',(-0.748809377631163,0.357796847151619,
-0.6363789196904));
#69398=CARTESIAN_POINT('Ctrl Pts',(-0.820649583666188,-0.345714150263954,
-0.609901255533077));
#69399=CARTESIAN_POINT('Ctrl Pts',(-0.151421980355895,-0.87820050681865,
-0.578128058544288));
#69400=CARTESIAN_POINT('Ctrl Pts',(0.518857616055017,-0.647685501528246,
-0.551650394386966));
#69401=CARTESIAN_POINT('Ctrl Pts',(0.759424772369192,-0.190855020100471,
-0.530468263061107));
#69402=CARTESIAN_POINT('Ctrl Pts',(0.76306463279521,0.327971932825795,-0.509286131735249));
#69403=CARTESIAN_POINT('Ctrl Pts',(0.377575861208738,0.739544570500736,
-0.488104000409392));
#69404=CARTESIAN_POINT('Ctrl Pts',(-0.141216211695821,0.771002588600507,
-0.466921869083532));
#69405=CARTESIAN_POINT('Ctrl Pts',(-0.493214572385959,0.611360104474943,
-0.451035270589139));
#69406=CARTESIAN_POINT('Ctrl Pts',(-0.724001752965214,0.300347002913539,
-0.435148672094745));
#69407=CARTESIAN_POINT('Ctrl Pts',(-0.802356556010187,-0.212033778434851,
-0.413966540768886));
#69408=CARTESIAN_POINT('Ctrl Pts',(-0.401692126280537,-0.794750299379084,
-0.387488876611564));
#69409=CARTESIAN_POINT('Ctrl Pts',(0.453091810094164,-0.767378607107432,
-0.355715679622776));
#69410=CARTESIAN_POINT('Ctrl Pts',(0.814750920558571,-0.157778118181504,
-0.329238015465453));
#69411=CARTESIAN_POINT('Ctrl Pts',(0.702374874168397,0.346150068442172,
-0.308055884139595));
#69412=CARTESIAN_POINT('Ctrl Pts',(0.369293024947228,0.743942379054456,
-0.286873752813738));
#69413=CARTESIAN_POINT('Ctrl Pts',(-0.190972491990077,0.80811205708209,
-0.265691621487879));
#69414=CARTESIAN_POINT('Ctrl Pts',(-0.606730035741863,0.496217965426545,
-0.24450949016202));
#69415=CARTESIAN_POINT('Ctrl Pts',(-0.771718314924831,0.146723681079384,
-0.228622891667627));
#69416=CARTESIAN_POINT('Ctrl Pts',(-0.746204491110825,-0.239825074069584,
-0.212736293173232));
#69417=CARTESIAN_POINT('Ctrl Pts',(-0.474403504239302,-0.68088258957028,
-0.191554161847375));
#69418=CARTESIAN_POINT('Ctrl Pts',(0.208556009763689,-0.866067206476802,
-0.165076497690051));
#69419=CARTESIAN_POINT('Ctrl Pts',(0.841689935707378,-0.29109045562369,
-0.133303300701264));
#69420=CARTESIAN_POINT('Ctrl Pts',(0.723834370006008,0.406353263108837,
-0.106825636543941));
#69421=CARTESIAN_POINT('Ctrl Pts',(0.310318878599919,0.719620732838044,
-0.0856435052180828));
#69422=CARTESIAN_POINT('Ctrl Pts',(-0.0705387118779829,0.782181820540678,
-0.0697569067236875));
#69423=CARTESIAN_POINT('Ctrl Pts',(-0.437154537896543,0.651981105845494,
-0.0538703082292969));
#69424=CARTESIAN_POINT('Ctrl Pts',(-0.609248872823355,0.459854686869421,
-0.0432792425663656));
#69425=CARTESIAN_POINT('Ctrl Pts',(-0.667283755215006,0.348842645238897,
-0.0379837097349007));
#69426=CARTESIAN_POINT('Ctrl Pts',(0.415028236876425,-0.582012248187004,
-11.9309162902651));
#69427=CARTESIAN_POINT('Ctrl Pts',(0.511854163508475,-0.51296646136859,
-11.9256207574336));
#69428=CARTESIAN_POINT('Ctrl Pts',(0.670087794403581,-0.326089049241816,
-11.9150296917707));
#69429=CARTESIAN_POINT('Ctrl Pts',(0.744730245171791,0.0356362322782299,
-11.8991430932763));
#69430=CARTESIAN_POINT('Ctrl Pts',(0.636250090767451,0.385624774244037,
-11.8832564947819));
#69431=CARTESIAN_POINT('Ctrl Pts',(0.287757616503084,0.733640547045757,
-11.8620743634561));
#69432=CARTESIAN_POINT('Ctrl Pts',(-0.383456490043703,0.75354609726296,
-11.8355966992987));
#69433=CARTESIAN_POINT('Ctrl Pts',(-0.84160538740142,0.0832144579414285,
-11.80382350231));
#69434=CARTESIAN_POINT('Ctrl Pts',(-0.578431492064404,-0.534873771688162,
-11.7773458381526));
#69435=CARTESIAN_POINT('Ctrl Pts',(-0.128244477331174,-0.732967324015595,
-11.7561637068268));
#69436=CARTESIAN_POINT('Ctrl Pts',(0.238577604025672,-0.706567602715354,
-11.7402771083324));
#69437=CARTESIAN_POINT('Ctrl Pts',(0.545720466397418,-0.505857385659933,
-11.724390509838));
#69438=CARTESIAN_POINT('Ctrl Pts',(0.784814276644656,-0.0742348289681934,
-11.7032083785121));
#69439=CARTESIAN_POINT('Ctrl Pts',(0.651433163568701,0.44425251973168,-11.6820262471863));
#69440=CARTESIAN_POINT('Ctrl Pts',(0.233942323917106,0.705612521504789,
-11.6608441158604));
#69441=CARTESIAN_POINT('Ctrl Pts',(-0.25458267785024,0.745592758200979,
-11.6396619845345));
#69442=CARTESIAN_POINT('Ctrl Pts',(-0.780680935113796,0.326032206682622,
-11.6131843203772));
#69443=CARTESIAN_POINT('Ctrl Pts',(-0.69498736268188,-0.481342937675468,
-11.5814111233884));
#69444=CARTESIAN_POINT('Ctrl Pts',(-0.0947903846137628,-0.782147648046809,
-11.5549334592311));
#69445=CARTESIAN_POINT('Ctrl Pts',(0.37681872151215,-0.641669810040819,
-11.5337513279052));
#69446=CARTESIAN_POINT('Ctrl Pts',(0.639197522483424,-0.384101318856191,
-11.5178647294109));
#69447=CARTESIAN_POINT('Ctrl Pts',(0.743431501282844,-0.0322836142324497,
-11.5019781309165));
#69448=CARTESIAN_POINT('Ctrl Pts',(0.646217846697502,0.451468074312828,
-11.4807959995906));
#69449=CARTESIAN_POINT('Ctrl Pts',(0.208936536557157,0.760313131267001,
-11.4596138682647));
#69450=CARTESIAN_POINT('Ctrl Pts',(-0.27847443281849,0.68925408536552,-11.4384317369389));
#69451=CARTESIAN_POINT('Ctrl Pts',(-0.676699493032713,0.403479561635729,
-11.417249605613));
#69452=CARTESIAN_POINT('Ctrl Pts',(-0.806086988029912,-0.25687713306994,
-11.3907719414558));
#69453=CARTESIAN_POINT('Ctrl Pts',(-0.218113661252782,-0.81677680986074,
-11.3589987444669));
#69454=CARTESIAN_POINT('Ctrl Pts',(0.43407642426811,-0.657508592639888,
-11.3325210803096));
#69455=CARTESIAN_POINT('Ctrl Pts',(0.702594455791664,-0.245140299377268,
-11.3113389489837));
#69456=CARTESIAN_POINT('Ctrl Pts',(0.735839301880873,0.121027553653736,
-11.2954523504894));
#69457=CARTESIAN_POINT('Ctrl Pts',(0.58753558633177,0.456655915830853,-11.279565751995));
#69458=CARTESIAN_POINT('Ctrl Pts',(0.200282317827862,0.762435503674711,
-11.2583836206691));
#69459=CARTESIAN_POINT('Ctrl Pts',(-0.332941019414456,0.714759261957186,
-11.2372014893433));
#69460=CARTESIAN_POINT('Ctrl Pts',(-0.658440964812338,0.345072034184339,
-11.2160193580174));
#69461=CARTESIAN_POINT('Ctrl Pts',(-0.776967605321815,-0.130534639197338,
-11.1948372266915));
#69462=CARTESIAN_POINT('Ctrl Pts',(-0.448102068257463,-0.717611756999146,
-11.1683595625342));
#69463=CARTESIAN_POINT('Ctrl Pts',(0.362498219216689,-0.763736190311011,
-11.1365863655454));
#69464=CARTESIAN_POINT('Ctrl Pts',(0.756488843802834,-0.2201465861157,-11.1101087013881));
#69465=CARTESIAN_POINT('Ctrl Pts',(0.694203209002715,0.267982538451035,
-11.0889265700622));
#69466=CARTESIAN_POINT('Ctrl Pts',(0.482502477870242,0.568593444849717,
-11.0730399715678));
#69467=CARTESIAN_POINT('Ctrl Pts',(0.152196914730789,0.728401530662744,
-11.0571533730735));
#69468=CARTESIAN_POINT('Ctrl Pts',(-0.340911127398258,0.710774582661878,
-11.0359712417476));
#69469=CARTESIAN_POINT('Ctrl Pts',(-0.716465727379952,0.329252769757259,
-11.0147891104217));
#69470=CARTESIAN_POINT('Ctrl Pts',(-0.7252408739192,-0.163232618497991,
-10.9936069790959));
#69471=CARTESIAN_POINT('Ctrl Pts',(-0.507695658401522,-0.602464165054588,
-10.97242484777));
#69472=CARTESIAN_POINT('Ctrl Pts',(0.123008428398455,-0.837037050495868,
-10.9459471836127));
#69473=CARTESIAN_POINT('Ctrl Pts',(0.770699286912404,-0.347448609847742,
-10.9141739866239));
#69474=CARTESIAN_POINT('Ctrl Pts',(0.719101275335622,0.321921179769178,
-10.8876963224665));
#69475=CARTESIAN_POINT('Ctrl Pts',(0.355636165011655,0.653647959104139,
-10.8665141911407));
#69476=CARTESIAN_POINT('Ctrl Pts',(-0.000321386690041276,0.745725850019615,
-10.8506275926463));
#69477=CARTESIAN_POINT('Ctrl Pts',(-0.35552940505769,0.653705998798072,
-10.8347409941519));
#69478=CARTESIAN_POINT('Ctrl Pts',(-0.719960978738509,0.321056215071895,
-10.8135588628261));
#69479=CARTESIAN_POINT('Ctrl Pts',(-0.759226175895796,-0.212852387201534,
-10.7923767315002));
#69480=CARTESIAN_POINT('Ctrl Pts',(-0.447102902654478,-0.593900839688561,
-10.7711946001744));
#69481=CARTESIAN_POINT('Ctrl Pts',(0.00304566864510004,-0.787850668361192,
-10.7500124688485));
#69482=CARTESIAN_POINT('Ctrl Pts',(0.635613857181148,-0.558352148665305,
-10.7235348046912));
#69483=CARTESIAN_POINT('Ctrl Pts',(0.812341618079216,0.23409191115644,-10.6917616077024));
#69484=CARTESIAN_POINT('Ctrl Pts',(0.339695932367431,0.710877319729864,
-10.6652839435451));
#69485=CARTESIAN_POINT('Ctrl Pts',(-0.152077971138047,0.728426404655775,
-10.6441018122192));
#69486=CARTESIAN_POINT('Ctrl Pts',(-0.482992393837075,0.568177343945017,
-10.6282152137248));
#69487=CARTESIAN_POINT('Ctrl Pts',(-0.69415940968358,0.268095887087071,
-10.6123286152304));
#69488=CARTESIAN_POINT('Ctrl Pts',(-0.75658416484695,-0.22136238534414,
-10.5911464839045));
#69489=CARTESIAN_POINT('Ctrl Pts',(-0.440884710216198,-0.653721039282296,
-10.5699643525787));
#69490=CARTESIAN_POINT('Ctrl Pts',(0.043685421188573,-0.742098913164826,
-10.5487822212529));
#69491=CARTESIAN_POINT('Ctrl Pts',(0.512338419743362,-0.598520923100893,
-10.527600089927));
#69492=CARTESIAN_POINT('Ctrl Pts',(0.845909660974294,-0.014104709504769,
-10.5011224257697));
#69493=CARTESIAN_POINT('Ctrl Pts',(0.467619355160476,0.704294019576864,
-10.4693492287809));
#69494=CARTESIAN_POINT('Ctrl Pts',(-0.20127503533384,0.761727149525769,
-10.4428715646235));
#69495=CARTESIAN_POINT('Ctrl Pts',(-0.587461030951866,0.45675187292246,
-10.4216894332977));
#69496=CARTESIAN_POINT('Ctrl Pts',(-0.735943347206106,0.120393257203035,
-10.4058028348033));
#69497=CARTESIAN_POINT('Ctrl Pts',(-0.702634449225675,-0.245025552721734,
-10.3899162363089));
#69498=CARTESIAN_POINT('Ctrl Pts',(-0.433362025741317,-0.658496969459834,
-10.368734104983));
#69499=CARTESIAN_POINT('Ctrl Pts',(0.0871496215066032,-0.783667957986035,
-10.3475519736572));
#69500=CARTESIAN_POINT('Ctrl Pts',(0.513696156330839,-0.537341113182083,
-10.3263698423313));
#69501=CARTESIAN_POINT('Ctrl Pts',(0.777953608135155,-0.12452363359687,
-10.3051877110055));
#69502=CARTESIAN_POINT('Ctrl Pts',(0.653875292926478,0.536851188561754,
-10.2787100468481));
#69503=CARTESIAN_POINT('Ctrl Pts',(-0.0995112619803705,0.839520956302764,
-10.2469368498594));
#69504=CARTESIAN_POINT('Ctrl Pts',(-0.646515899350175,0.450285556131582,
-10.220459185702));
#69505=CARTESIAN_POINT('Ctrl Pts',(-0.743436834368463,-0.0321622388741894,
-10.1992770543762));
#69506=CARTESIAN_POINT('Ctrl Pts',(-0.638866127347263,-0.384652073964505,
-10.1833904558818));
#69507=CARTESIAN_POINT('Ctrl Pts',(-0.376923639214111,-0.641608339196779,
-10.1675038573874));
#69508=CARTESIAN_POINT('Ctrl Pts',(0.0959750524998173,-0.782438300085102,
-10.1463217260615));
#69509=CARTESIAN_POINT('Ctrl Pts',(0.573733992537099,-0.540888002002435,
-10.1251395947357));
#69510=CARTESIAN_POINT('Ctrl Pts',(0.739383564307667,-0.0770140102612942,
-10.1039574634098));
#69511=CARTESIAN_POINT('Ctrl Pts',(0.673559771585897,0.408699383209504,
-10.082775332084));
#69512=CARTESIAN_POINT('Ctrl Pts',(0.150845825635244,0.832470800838251,
-10.0562976679266));
#69513=CARTESIAN_POINT('Ctrl Pts',(-0.619312495169557,0.575456306472777,
-10.0245244709379));
#69514=CARTESIAN_POINT('Ctrl Pts',(-0.784261926880214,-0.0753201182913833,
-9.99804680678051));
#69515=CARTESIAN_POINT('Ctrl Pts',(-0.545820424427594,-0.505779399128595,
-9.97686467545469));
#69516=CARTESIAN_POINT('Ctrl Pts',(-0.237932443072409,-0.706749813732185,
-9.96097807696027));
#69517=CARTESIAN_POINT('Ctrl Pts',(0.128058976679507,-0.733030414933145,
-9.94509147846588));
#69518=CARTESIAN_POINT('Ctrl Pts',(0.579664632968886,-0.534237603906211,
-9.92390934714004));
#69519=CARTESIAN_POINT('Ctrl Pts',(0.787439938769152,-0.0408517776110334,
-9.90272721581415));
#69520=CARTESIAN_POINT('Ctrl Pts',(0.613406568615596,0.419942370479663,
-9.88154508448832));
#69521=CARTESIAN_POINT('Ctrl Pts',(0.248808536191952,0.74753746665481,-9.86036295316244));
#69522=CARTESIAN_POINT('Ctrl Pts',(-0.423928686959554,0.732152009990144,
-9.83388528900514));
#69523=CARTESIAN_POINT('Ctrl Pts',(-0.844557330553996,0.0376940677022658,
-9.80211209201634));
#69524=CARTESIAN_POINT('Ctrl Pts',(-0.548998577207228,-0.565102161027307,
-9.775634427859));
#69525=CARTESIAN_POINT('Ctrl Pts',(-0.0886017953782055,-0.738838587352449,
-9.75445229653318));
#69526=CARTESIAN_POINT('Ctrl Pts',(0.276166281305673,-0.692704360998744,
-9.73856569803876));
#69527=CARTESIAN_POINT('Ctrl Pts',(0.57213439116594,-0.475809761533366,
-9.72267909954437));
#69528=CARTESIAN_POINT('Ctrl Pts',(0.787655067120261,-0.0319436908039809,
-9.70149696821853));
#69529=CARTESIAN_POINT('Ctrl Pts',(0.626624986972285,0.478614302549277,
-9.68031483689264));
#69530=CARTESIAN_POINT('Ctrl Pts',(0.195682142263798,0.717166446610471,
-9.65913270556681));
#69531=CARTESIAN_POINT('Ctrl Pts',(-0.294280608957396,0.73083300070969,
-9.63795057424093));
#69532=CARTESIAN_POINT('Ctrl Pts',(-0.797074929608463,0.283608275530733,
-9.61147291008363));
#69533=CARTESIAN_POINT('Ctrl Pts',(-0.668115187284044,-0.5179961620059,
-9.57969971309482));
#69534=CARTESIAN_POINT('Ctrl Pts',(-0.0526214205896454,-0.78611123657433,
-9.5532220489375));
#69535=CARTESIAN_POINT('Ctrl Pts',(0.410757474929328,-0.62049257295707,
-9.53203991761165));
#69536=CARTESIAN_POINT('Ctrl Pts',(0.658915249864171,-0.349195991061354,
-9.51615331911726));
#69537=CARTESIAN_POINT('Ctrl Pts',(0.744092180646416,0.00771475379514762,
-9.50026672062285));
#69538=CARTESIAN_POINT('Ctrl Pts',(0.621022284247614,0.485543228364149,
-9.47908458929701));
#69539=CARTESIAN_POINT('Ctrl Pts',(0.167775681958537,0.770442629561796,
-9.45790245797112));
#69540=CARTESIAN_POINT('Ctrl Pts',(-0.315112305102429,0.67329298831777,
-9.4367203266453));
#69541=CARTESIAN_POINT('Ctrl Pts',(-0.697404491344613,0.366530936193706,
-9.4155381953194));
#69542=CARTESIAN_POINT('Ctrl Pts',(-0.791117695616473,-0.299824763891077,
-9.38906053116213));
#69543=CARTESIAN_POINT('Ctrl Pts',(-0.173905189465712,-0.827317902870068,
-9.35728733417329));
#69544=CARTESIAN_POINT('Ctrl Pts',(0.468783450174122,-0.633231369260984,
-9.33080967001601));
#69545=CARTESIAN_POINT('Ctrl Pts',(0.714752945652261,-0.207028894086353,
-9.30962753869013));
#69546=CARTESIAN_POINT('Ctrl Pts',(0.728272023089266,0.160396406014447,
-9.29374094019575));
#69547=CARTESIAN_POINT('Ctrl Pts',(0.562146062042697,0.487569990519461,
-9.27785434170134));
#69548=CARTESIAN_POINT('Ctrl Pts',(0.159019896480474,0.772096870001262,
-9.2566722103755));
#69549=CARTESIAN_POINT('Ctrl Pts',(-0.370870818981993,0.695834290999209,
-9.23549007904961));
#69550=CARTESIAN_POINT('Ctrl Pts',(-0.676033552397828,0.309189018202799,
-9.21430794772379));
#69551=CARTESIAN_POINT('Ctrl Pts',(-0.768829988206647,-0.172099973761879,
-9.1931258163979));
#69552=CARTESIAN_POINT('Ctrl Pts',(-0.40889035488849,-0.740655638633112,
-9.1666481522406));
#69553=CARTESIAN_POINT('Ctrl Pts',(0.403017310632342,-0.743152053528152,
-9.1348749552518));
#69554=CARTESIAN_POINT('Ctrl Pts',(0.767226301746,-0.179175031972786,-9.10839729109448));
#69555=CARTESIAN_POINT('Ctrl Pts',(0.678798787336911,0.304901529374881,
-9.08721515976862));
#69556=CARTESIAN_POINT('Ctrl Pts',(0.451249245738007,0.593701326339906,
-9.07132856127423));
#69557=CARTESIAN_POINT('Ctrl Pts',(0.112832951222732,0.735527984405508,
-9.05544196277983));
#69558=CARTESIAN_POINT('Ctrl Pts',(-0.378615274819878,0.691427058926299,
-9.03425983145398));
#69559=CARTESIAN_POINT('Ctrl Pts',(-0.733124346516869,0.290274383036051,
-9.01307770012811));
#69560=CARTESIAN_POINT('Ctrl Pts',(-0.715420825257699,-0.201970927938732,
-8.99189556880227));
#69561=CARTESIAN_POINT('Ctrl Pts',(-0.474585821341943,-0.628876975183433,
-8.97071343747639));
#69562=CARTESIAN_POINT('Ctrl Pts',(0.167812748838726,-0.829217087792485,
-8.94423577331909));
#69563=CARTESIAN_POINT('Ctrl Pts',(0.788257375451387,-0.305529437827074,
-8.91246257633028));
#69564=CARTESIAN_POINT('Ctrl Pts',(0.700762232327224,0.360100241484309,
-8.88598491217298));
#69565=CARTESIAN_POINT('Ctrl Pts',(0.319995458059088,0.671815185245732,
-8.8648027808471));
#69566=CARTESIAN_POINT('Ctrl Pts',(-0.040395961119228,0.744630991164172,
-8.84891618235272));
#69567=CARTESIAN_POINT('Ctrl Pts',(-0.390145583636105,0.633655359240732,
-8.83302958385832));
#69568=CARTESIAN_POINT('Ctrl Pts',(-0.736174067273288,0.281901838973623,
-8.81184745253247));
#69569=CARTESIAN_POINT('Ctrl Pts',(-0.746690469329113,-0.253345353057471,
-8.7906653212066));
#69570=CARTESIAN_POINT('Ctrl Pts',(-0.414540813271791,-0.617069791090766,
-8.76948318988076));
#69571=CARTESIAN_POINT('Ctrl Pts',(0.0453800790159918,-0.786548536431907,
-8.74830105855488));
#69572=CARTESIAN_POINT('Ctrl Pts',(0.664701026950137,-0.523387659513758,
-8.72182339439757));
#69573=CARTESIAN_POINT('Ctrl Pts',(0.798587754341329,0.277408590257236,
-8.69005019740877));
#69574=CARTESIAN_POINT('Ctrl Pts',(0.301002774099267,0.728105226020141,
-8.66357253325146));
#69575=CARTESIAN_POINT('Ctrl Pts',(-0.191003588526136,0.719201199578629,
-8.6423904019256));
#69576=CARTESIAN_POINT('Ctrl Pts',(-0.512828106903175,0.541400479725488,
-8.62650380343121));
#69577=CARTESIAN_POINT('Ctrl Pts',(-0.707563712994288,0.230404606679193,
-8.61061720493682));
#69578=CARTESIAN_POINT('Ctrl Pts',(-0.743594951797162,-0.261701073372229,
-8.58943507361094));
#69579=CARTESIAN_POINT('Ctrl Pts',(-0.405116890236114,-0.676469385965225,
-8.5682529422851));
#69580=CARTESIAN_POINT('Ctrl Pts',(0.0835024235041277,-0.738678927690356,
-8.54707081095923));
#69581=CARTESIAN_POINT('Ctrl Pts',(0.543762380284107,-0.570123166975729,
-8.52588867963338));
#69582=CARTESIAN_POINT('Ctrl Pts',(0.845445287876903,0.0313745528509859,
-8.49941101547605));
#69583=CARTESIAN_POINT('Ctrl Pts',(0.429095129360905,0.728405997566729,
-8.46763781848728));
#69584=CARTESIAN_POINT('Ctrl Pts',(-0.24191913210034,0.749809991729314,
-8.44116015432992));
#69585=CARTESIAN_POINT('Ctrl Pts',(-0.611157820186959,0.42452191360344,
-8.4199780230041));
#69586=CARTESIAN_POINT('Ctrl Pts',(-0.74134978577321,0.080669956061101,
-8.40409142450968));
#69587=CARTESIAN_POINT('Ctrl Pts',(-0.688451544413171,-0.282430808730881,
-8.38820482601531));
#69588=CARTESIAN_POINT('Ctrl Pts',(-0.3973484194103,-0.68083414847857,-8.36702269468943));
#69589=CARTESIAN_POINT('Ctrl Pts',(0.129137722759079,-0.777852153987728,
-8.34584056336358));
#69590=CARTESIAN_POINT('Ctrl Pts',(0.541830373946935,-0.508958798738525,
-8.32465843203773));
#69591=CARTESIAN_POINT('Ctrl Pts',(0.783521306039094,-0.0825367476792268,
-8.30347630071186));
#69592=CARTESIAN_POINT('Ctrl Pts',(0.624080241337119,0.571214451613806,
-8.27699863655454));
#69593=CARTESIAN_POINT('Ctrl Pts',(-0.144483020465117,0.832960133577659,
-8.24522543956576));
#69594=CARTESIAN_POINT('Ctrl Pts',(-0.66977985567032,0.414891353382473,
-8.21874777540842));
#69595=CARTESIAN_POINT('Ctrl Pts',(-0.740634167244186,-0.0720677918054417,
-8.19756564408258));
#69596=CARTESIAN_POINT('Ctrl Pts',(-0.617271889931151,-0.418428680395727,
-8.18167904558817));
#69597=CARTESIAN_POINT('Ctrl Pts',(-0.341899176308968,-0.66093694401547,
-8.1657924470938));
#69598=CARTESIAN_POINT('Ctrl Pts',(0.137884319468111,-0.776149997479365,
-8.14461031576791));
#69599=CARTESIAN_POINT('Ctrl Pts',(0.601972062897985,-0.509274150525132,
-8.12342818444209));
#69600=CARTESIAN_POINT('Ctrl Pts',(0.742453846576301,-0.0371685169046532,
-8.1022460531162));
#69601=CARTESIAN_POINT('Ctrl Pts',(0.650623107466303,0.444305664791217,
-8.08106392179036));
#69602=CARTESIAN_POINT('Ctrl Pts',(0.105891169344639,0.839374265518477,
-8.05458625763302));
#69603=CARTESIAN_POINT('Ctrl Pts',(-0.649342391994081,0.541343130825394,
-8.02281306064425));
#69604=CARTESIAN_POINT('Ctrl Pts',(-0.779080977831934,-0.117357233069515,
-7.99633539648691));
#69605=CARTESIAN_POINT('Ctrl Pts',(-0.517851300905695,-0.534380731740471,
-7.97515326516107));
#69606=CARTESIAN_POINT('Ctrl Pts',(-0.199608145616148,-0.718514951048735,
-7.95926666666666));
#69607=CARTESIAN_POINT('Ctrl Pts',(0.167266719814572,-0.725089329095204,
-7.94338006817229));
#69608=CARTESIAN_POINT('Ctrl Pts',(0.607536743444001,-0.502314651894469,
-7.92219793684639));
#69609=CARTESIAN_POINT('Ctrl Pts',(0.788497433317525,0.00152399292137779,
-7.90101580552058));
#69610=CARTESIAN_POINT('Ctrl Pts',(0.589952632896988,0.452299794254596,
-7.87983367419468));
#69611=CARTESIAN_POINT('Ctrl Pts',(0.208276608788832,0.759828142388853,
-7.85865154286886));
#69612=CARTESIAN_POINT('Ctrl Pts',(-0.462661687723661,0.708312261698578,
-7.8321738787115));
#69613=CARTESIAN_POINT('Ctrl Pts',(-0.845362595220247,-0.00774660796236431,
-7.80040068172274));
#69614=CARTESIAN_POINT('Ctrl Pts',(-0.517836877317961,-0.59378856393743,
-7.7739230175654));
#69615=CARTESIAN_POINT('Ctrl Pts',(-0.0487688443231488,-0.742532380525313,
-7.75274088623955));
#69616=CARTESIAN_POINT('Ctrl Pts',(0.312992899017785,-0.676862313798992,
-7.73685428774516));
#69617=CARTESIAN_POINT('Ctrl Pts',(0.596877491755274,-0.444375911319675,
-7.72096768925076));
#69618=CARTESIAN_POINT('Ctrl Pts',(0.788233533424651,0.0104307682983569,
-7.69978555792491));
#69619=CARTESIAN_POINT('Ctrl Pts',(0.599998941877613,0.511597297342836,
-7.67860342659904));
#69620=CARTESIAN_POINT('Ctrl Pts',(0.156859111171333,0.726646015737633,
-7.65742129527319));
#69621=CARTESIAN_POINT('Ctrl Pts',(-0.333130070508813,0.713962399470354,
-7.63623916394732));
#69622=CARTESIAN_POINT('Ctrl Pts',(-0.811164148261794,0.240363936426778,
-7.60976149979001));
#69623=CARTESIAN_POINT('Ctrl Pts',(-0.639312821126197,-0.553151917718901,
-7.57798830280121));
#69624=CARTESIAN_POINT('Ctrl Pts',(-0.010300046683182,-0.787803147500451,
-7.55151063864389));
#69625=CARTESIAN_POINT('Ctrl Pts',(0.443508970371773,-0.597521990812866,
-7.53032850731804));
#69626=CARTESIAN_POINT('Ctrl Pts',(0.676728772042507,-0.313281527969212,
-7.51444190882364));
#69627=CARTESIAN_POINT('Ctrl Pts',(0.742602365585634,0.0476908518678349,
-7.49855531032925));
#69628=CARTESIAN_POINT('Ctrl Pts',(0.594031977182028,0.518215123503371,
-7.47737317900339));
#69629=CARTESIAN_POINT('Ctrl Pts',(0.126129933316543,0.778345530483932,
-7.45619104767754));
#69630=CARTESIAN_POINT('Ctrl Pts',(-0.350839484906702,0.655386045606128,
-7.43500891635167));
#69631=CARTESIAN_POINT('Ctrl Pts',(-0.716093969570523,0.32852302579789,
-7.41382678502582));
#69632=CARTESIAN_POINT('Ctrl Pts',(-0.773862040986492,-0.341905891847567,
-7.3873491208685));
#69633=CARTESIAN_POINT('Ctrl Pts',(-0.129194126850317,-0.835468015497788,
-7.3555759238797));
#69634=CARTESIAN_POINT('Ctrl Pts',(0.502135675338213,-0.607124084290786,
-7.32909825972239));
#69635=CARTESIAN_POINT('Ctrl Pts',(0.724845772692903,-0.168319167400595,
-7.30791612839653));
#69636=CARTESIAN_POINT('Ctrl Pts',(0.718600011399384,0.199301706700394,
-7.29202952990213));
#69637=CARTESIAN_POINT('Ctrl Pts',(0.535131914738594,0.517074969954517,
-7.27614293140774));
#69638=CARTESIAN_POINT('Ctrl Pts',(0.117297901824557,0.779526847754431,
-7.25496080008188));
#69639=CARTESIAN_POINT('Ctrl Pts',(-0.407728788196936,0.674898333216349,
-7.23377866875603));
#69640=CARTESIAN_POINT('Ctrl Pts',(-0.691672377986925,0.27241243450832,
-7.21259653743016));
#69641=CARTESIAN_POINT('Ctrl Pts',(-0.758470423987435,-0.213167933026972,
-7.19141440610431));
#69642=CARTESIAN_POINT('Ctrl Pts',(-0.368496933257126,-0.761558998069061,
-7.16493674194697));
#69643=CARTESIAN_POINT('Ctrl Pts',(0.442371667103622,-0.720420179809253,
-7.1331635449582));
#69644=CARTESIAN_POINT('Ctrl Pts',(0.77574644728917,-0.137685655358597,
-7.10668588080086));
#69645=CARTESIAN_POINT('Ctrl Pts',(0.661432612057195,0.340939343597065,
-7.08550374947501));
#69646=CARTESIAN_POINT('Ctrl Pts',(0.418691886588421,0.617093389027879,
-7.06961715098062));
#69647=CARTESIAN_POINT('Ctrl Pts',(0.0731428963102508,0.740528735056654,
-7.05373055248622));
#69648=CARTESIAN_POINT('Ctrl Pts',(-0.415225210087146,0.670081285405351,
-7.03254842116036));
#69649=CARTESIAN_POINT('Ctrl Pts',(-0.747664209164554,0.250457092606872,
-7.01136628983452));
#69650=CARTESIAN_POINT('Ctrl Pts',(-0.70353318393837,-0.240125533924201,
-6.99018415850864));
#69651=CARTESIAN_POINT('Ctrl Pts',(-0.440104413697557,-0.653472307583564,
-6.9690020271828));
#69652=CARTESIAN_POINT('Ctrl Pts',(0.212132084225257,-0.819000657021791,
-6.94252436302547));
#69653=CARTESIAN_POINT('Ctrl Pts',(0.803537371007348,-0.262727274425518,
-6.91075116603669));
#69654=CARTESIAN_POINT('Ctrl Pts',(0.68039796053698,0.397238600176665,-6.88427350187936));
#69655=CARTESIAN_POINT('Ctrl Pts',(0.283429952391962,0.688040840642773,
-6.8630913705535));
#69656=CARTESIAN_POINT('Ctrl Pts',(-0.0803537897261284,0.741384121190458,
-6.8472047720591));
#69657=CARTESIAN_POINT('Ctrl Pts',(-0.42363422704096,0.611773432248228,
-6.83131817356472));
#69658=CARTESIAN_POINT('Ctrl Pts',(-0.750259585513473,0.241932756128878,
-6.81013604223885));
#69659=CARTESIAN_POINT('Ctrl Pts',(-0.731996799675116,-0.293106141467353,
-6.788953910913));
#69660=CARTESIAN_POINT('Ctrl Pts',(-0.380780685600718,-0.638455387964545,
-6.76777177958714));
#69661=CARTESIAN_POINT('Ctrl Pts',(0.0875833392822713,-0.782973250124461,
-6.74658964826127));
#69662=CARTESIAN_POINT('Ctrl Pts',(0.691867186148921,-0.48691056066591,
-6.72011198410396));
#69663=CARTESIAN_POINT('Ctrl Pts',(0.78252594245428,0.319923548278934,-6.68833878711517));
#69664=CARTESIAN_POINT('Ctrl Pts',(0.261439706657101,0.743228881245174,
-6.66186112295785));
#69665=CARTESIAN_POINT('Ctrl Pts',(-0.22937719844958,0.707897476449544,
-6.64067899163199));
#69666=CARTESIAN_POINT('Ctrl Pts',(-0.541181727820946,0.513058948026012,
-6.62479239313759));
#69667=CARTESIAN_POINT('Ctrl Pts',(-0.718923130886396,0.192047448544228,
-6.60890579464321));
#69668=CARTESIAN_POINT('Ctrl Pts',(-0.728456722063183,-0.301283435869895,
-6.58772366331733));
#69669=CARTESIAN_POINT('Ctrl Pts',(-0.368178266988903,-0.69726271060162,
-6.56654153199149));
#69670=CARTESIAN_POINT('Ctrl Pts',(0.123078100183777,-0.733124133353885,
-6.54535940066562));
#69671=CARTESIAN_POINT('Ctrl Pts',(0.573614848692852,-0.54007773246291,
-6.52417726933977));
#69672=CARTESIAN_POINT('Ctrl Pts',(0.842537543914182,0.0767631387380145,
-6.49769960518244));
#69673=CARTESIAN_POINT('Ctrl Pts',(0.389330807518773,0.750412860295417,
-6.46592640819366));
#69674=CARTESIAN_POINT('Ctrl Pts',(-0.281864081683107,0.735725846801378,
-6.43944874403633));
#69675=CARTESIAN_POINT('Ctrl Pts',(-0.633088329546757,0.391065082029191,
-6.41826661271048));
#69676=CARTESIAN_POINT('Ctrl Pts',(-0.744613720371767,0.0407134900563816,
-6.40238001421609));
#69677=CARTESIAN_POINT('Ctrl Pts',(-0.672278943783744,-0.319019781338021,
-6.38649341572168));
#69678=CARTESIAN_POINT('Ctrl Pts',(-0.360186564983986,-0.701203800939871,
-6.36531128439583));
#69679=CARTESIAN_POINT('Ctrl Pts',(0.170752809752722,-0.769788118850823,
-6.34412915306997));
#69680=CARTESIAN_POINT('Ctrl Pts',(0.568398449615586,-0.479105819619089,
-6.32294702174411));
#69681=CARTESIAN_POINT('Ctrl Pts',(0.786825141210475,-0.0403107543443066,
-6.30176489041825));
#69682=CARTESIAN_POINT('Ctrl Pts',(0.592480419109261,0.603925663550727,
-6.27528722626093));
#69683=CARTESIAN_POINT('Ctrl Pts',(-0.18903518009993,0.823994176656527,
-6.24351402927215));
#69684=CARTESIAN_POINT('Ctrl Pts',(-0.691111574103426,0.378294455803269,
-6.21703636511482));
#69685=CARTESIAN_POINT('Ctrl Pts',(-0.735686261875505,-0.111760021107787,
-6.19585423378896));
#69686=CARTESIAN_POINT('Ctrl Pts',(-0.593904136703258,-0.451007017563935,
-6.17996763529457));
#69687=CARTESIAN_POINT('Ctrl Pts',(-0.305867183926357,-0.678334902943274,
-6.16408103680018));
#69688=CARTESIAN_POINT('Ctrl Pts',(0.17935076708676,-0.767665398060909,
-6.14289890547431));
#69689=CARTESIAN_POINT('Ctrl Pts',(0.628555407221239,-0.476098731549411,
-6.12171677414847));
#69690=CARTESIAN_POINT('Ctrl Pts',(0.743279060887722,0.00267948462979709,
-6.1005346428226));
#69691=CARTESIAN_POINT('Ctrl Pts',(0.626038073573313,0.478872969492467,
-6.07935251149674));
#69692=CARTESIAN_POINT('Ctrl Pts',(0.0601411841463684,0.843333225837006,
-6.05287484733942));
#69693=CARTESIAN_POINT('Ctrl Pts',(-0.676657201314584,0.506563508686106,
-6.02110165035063));
#69694=CARTESIAN_POINT('Ctrl Pts',(-0.792167923235142,-0.293888061665043,
-5.98932845336184));
#69695=CARTESIAN_POINT('Ctrl Pts',(-0.18232501179644,-0.825019879436455,
-5.95755525637306));
#69696=CARTESIAN_POINT('Ctrl Pts',(0.594682153850289,-0.600686850459742,
-5.92578205938427));
#69697=CARTESIAN_POINT('Ctrl Pts',(0.827085846200354,0.1753764375457,-5.89400886239548));
#69698=CARTESIAN_POINT('Ctrl Pts',(0.38837020223537,0.685865567359653,-5.86753119823816));
#69699=CARTESIAN_POINT('Ctrl Pts',(-0.0994116151163395,0.736605914157616,
-5.84634906691231));
#69700=CARTESIAN_POINT('Ctrl Pts',(-0.557900719683635,0.557224092360063,
-5.82516693558644));
#69701=CARTESIAN_POINT('Ctrl Pts',(-0.785021415731397,0.0722373717524209,
-5.80398480426059));
#69702=CARTESIAN_POINT('Ctrl Pts',(-0.629907910310793,-0.396117405931614,
-5.78280267293472));
#69703=CARTESIAN_POINT('Ctrl Pts',(-0.36518079795383,-0.650209534143389,
-5.76691607444034));
#69704=CARTESIAN_POINT('Ctrl Pts',(-0.00967822977447486,-0.744063780934671,
-5.75102947594593));
#69705=CARTESIAN_POINT('Ctrl Pts',(0.469613042710347,-0.632617967866498,
-5.72984734462008));
#69706=CARTESIAN_POINT('Ctrl Pts',(0.842146437172344,-0.0740950797098429,
-5.70336968046277));
#69707=CARTESIAN_POINT('Ctrl Pts',(0.516846346640217,0.669797811348866,
-5.67159648347396));
#69708=CARTESIAN_POINT('Ctrl Pts',(-0.147974275060897,0.773836141361268,
-5.64511881931665));
#69709=CARTESIAN_POINT('Ctrl Pts',(-0.552618678533357,0.497224074290783,
-5.62393668799079));
#69710=CARTESIAN_POINT('Ctrl Pts',(-0.785943372243192,0.0634293748143924,
-5.60275455666493));
#69711=CARTESIAN_POINT('Ctrl Pts',(-0.645101133300516,-0.453062534162647,
-5.58157242533907));
#69712=CARTESIAN_POINT('Ctrl Pts',(-0.223681593183752,-0.709717650908249,
-5.56039029401322));
#69713=CARTESIAN_POINT('Ctrl Pts',(0.142576800788917,-0.731969286729474,
-5.54450369551882));
#69714=CARTESIAN_POINT('Ctrl Pts',(0.474295047200469,-0.573390739018259,
-5.52861709702442));
#69715=CARTESIAN_POINT('Ctrl Pts',(0.767461368384907,-0.178165457458594,
-5.50743496569857));
#69716=CARTESIAN_POINT('Ctrl Pts',(0.689842000918259,0.488687990796851,
-5.48095730154124));
#69717=CARTESIAN_POINT('Ctrl Pts',(-0.0396597488537021,0.84509715222258,
-5.44918410455246));
#69718=CARTESIAN_POINT('Ctrl Pts',(-0.613729310297357,0.494018507168641,
-5.42270644039513));
#69719=CARTESIAN_POINT('Ctrl Pts',(-0.743080101331292,0.0212409193823935,
-5.40152430906928));
#69720=CARTESIAN_POINT('Ctrl Pts',(-0.64009997108623,-0.460437347414257,
-5.38034217774342));
#69721=CARTESIAN_POINT('Ctrl Pts',(-0.19839903481638,-0.762927734213757,
-5.35916004641756));
#69722=CARTESIAN_POINT('Ctrl Pts',(0.288949386831816,-0.685741162878066,
-5.33797791509171));
#69723=CARTESIAN_POINT('Ctrl Pts',(0.582512818373229,-0.465602795425132,
-5.3220913165973));
#69724=CARTESIAN_POINT('Ctrl Pts',(0.732689213904483,-0.129997123661407,
-5.30620471810292));
#69725=CARTESIAN_POINT('Ctrl Pts',(0.70028784709236,0.361021912560238,-5.28502258677706));
#69726=CARTESIAN_POINT('Ctrl Pts',(0.209437883142914,0.819044382473843,
-5.25854492261973));
#69727=CARTESIAN_POINT('Ctrl Pts',(-0.577303985580056,0.618451457748302,
-5.22677172563096));
#69728=CARTESIAN_POINT('Ctrl Pts',(-0.787582921563938,-0.0207627886158348,
-5.20029406147361));
#69729=CARTESIAN_POINT('Ctrl Pts',(-0.580119189696666,-0.464845069558873,
-5.17911193014777));
#69730=CARTESIAN_POINT('Ctrl Pts',(-0.18981308702806,-0.765311385576726,
-5.1579297988219));
#69731=CARTESIAN_POINT('Ctrl Pts',(0.342665194945523,-0.709930608099066,
-5.13674766749606));
#69732=CARTESIAN_POINT('Ctrl Pts',(0.664150772330552,-0.335613531220212,
-5.11556553617018));
#69733=CARTESIAN_POINT('Ctrl Pts',(0.745395018308445,0.0222129097069853,
-5.0996789376758));
#69734=CARTESIAN_POINT('Ctrl Pts',(0.642602943052109,0.375225524033337,
-5.0837923391814));
#69735=CARTESIAN_POINT('Ctrl Pts',(0.300044556024852,0.728500620846027,
-5.06261020785554));
#69736=CARTESIAN_POINT('Ctrl Pts',(-0.370578734356334,0.759848227592405,
-5.03613254369823));
#69737=CARTESIAN_POINT('Ctrl Pts',(-0.840371845689285,0.0976588876276082,
-5.00435934670943));
#69738=CARTESIAN_POINT('Ctrl Pts',(-0.58684762841035,-0.525668919343541,
-4.97788168255212));
#69739=CARTESIAN_POINT('Ctrl Pts',(-0.141242936706458,-0.729842206079766,
-4.95669955122626));
#69740=CARTESIAN_POINT('Ctrl Pts',(0.350752387995542,-0.70618927152582,
-4.93551741990039));
#69741=CARTESIAN_POINT('Ctrl Pts',(0.720751563935925,-0.319277445533383,
-4.91433528857454));
#69742=CARTESIAN_POINT('Ctrl Pts',(0.723469851944388,0.174138060322337,
-4.89315315724868));
#69743=CARTESIAN_POINT('Ctrl Pts',(0.553753656586301,0.499463746926826,
-4.87726655875429));
#69744=CARTESIAN_POINT('Ctrl Pts',(0.246882909622859,0.701984020645308,
-4.86137996025989));
#69745=CARTESIAN_POINT('Ctrl Pts',(-0.242905436915294,0.749491053242322,
-4.84019782893404));
#69746=CARTESIAN_POINT('Ctrl Pts',(-0.774341299252633,0.339254299315688,
-4.81372016477671));
#69747=CARTESIAN_POINT('Ctrl Pts',(-0.703743420627555,-0.469582043186583,
-4.78194696778792));
#69748=CARTESIAN_POINT('Ctrl Pts',(-0.10699682437215,-0.780557256906211,
-4.75546930363059));
#69749=CARTESIAN_POINT('Ctrl Pts',(0.364811051232433,-0.647712984155424,
-4.73428717230475));
#69750=CARTESIAN_POINT('Ctrl Pts',(0.724493584913005,-0.311190569141564,
-4.71310504097887));
#69751=CARTESIAN_POINT('Ctrl Pts',(0.756035250853362,0.223229934393878,
-4.69192290965303));
#69752=CARTESIAN_POINT('Ctrl Pts',(0.438693381781545,0.601066391928822,
-4.67074077832716));
#69753=CARTESIAN_POINT('Ctrl Pts',(0.0987368848287337,0.739160452304642,
-4.65485417983278));
#69754=CARTESIAN_POINT('Ctrl Pts',(-0.266259170196915,0.694866023483125,
-4.63896758133838));
#69755=CARTESIAN_POINT('Ctrl Pts',(-0.670325142540075,0.414009774584999,
-4.61778545001252));
#69756=CARTESIAN_POINT('Ctrl Pts',(-0.809812919660765,-0.242695204903068,
-4.5913077858552));
#69757=CARTESIAN_POINT('Ctrl Pts',(-0.232401698844621,-0.813481129304173,
-4.55953458886641));
#69758=CARTESIAN_POINT('Ctrl Pts',(0.423743634580864,-0.66419822635029,
-4.53305692470909));
#69759=CARTESIAN_POINT('Ctrl Pts',(0.697354202608967,-0.257519570224186,
-4.51187479338323));
#69760=CARTESIAN_POINT('Ctrl Pts',(0.753652325850476,0.23181608365883,-4.49069266205737));
#69761=CARTESIAN_POINT('Ctrl Pts',(0.431734686134142,0.659565057390897,
-4.46951053073151));
#69762=CARTESIAN_POINT('Ctrl Pts',(-0.0547337183721843,0.742116507563613,
-4.44832839940566));
#69763=CARTESIAN_POINT('Ctrl Pts',(-0.403240962883958,0.627298870180159,
-4.43244180091126));
#69764=CARTESIAN_POINT('Ctrl Pts',(-0.652763498207381,0.357256982735486,
-4.41655520241687));
#69765=CARTESIAN_POINT('Ctrl Pts',(-0.778925898305787,-0.118382157109167,
-4.395373071091));
#69766=CARTESIAN_POINT('Ctrl Pts',(-0.460122641396538,-0.709214412012832,
-4.36889540693369));
#69767=CARTESIAN_POINT('Ctrl Pts',(0.349474539501924,-0.77047364886787,
-4.33712220994489));
#69768=CARTESIAN_POINT('Ctrl Pts',(0.75294383789821,-0.231934319810118,
-4.31064454578758));
#69769=CARTESIAN_POINT('Ctrl Pts',(0.698222886706653,0.255154881246402,
-4.28946241446172));
#69770=CARTESIAN_POINT('Ctrl Pts',(0.424360178050591,0.66456674923413,-4.26828028313586));
#69771=CARTESIAN_POINT('Ctrl Pts',(-0.0979068251135458,0.782198924659571,
-4.24709815181));
#69772=CARTESIAN_POINT('Ctrl Pts',(-0.522128456757134,0.530202381520183,
-4.22591602048414));
#69773=CARTESIAN_POINT('Ctrl Pts',(-0.713430002198875,0.217082423607711,
-4.21002942198974));
#69774=CARTESIAN_POINT('Ctrl Pts',(-0.728801516963504,-0.150270040849453,
-4.19414282349536));
#69775=CARTESIAN_POINT('Ctrl Pts',(-0.517055190066955,-0.594469360520892,
-4.17296069216949));
#69776=CARTESIAN_POINT('Ctrl Pts',(0.108410416329209,-0.838418218411172,
-4.14648302801217));
#69777=CARTESIAN_POINT('Ctrl Pts',(0.765134267955551,-0.361014749504757,
-4.11470983102339));
#69778=CARTESIAN_POINT('Ctrl Pts',(0.724030122361315,0.310641809240379,
-4.08823216686606));
#69779=CARTESIAN_POINT('Ctrl Pts',(0.36700394141324,0.646472984688444,-4.06705003554021));
#69780=CARTESIAN_POINT('Ctrl Pts',(-0.106765464783411,0.781237262572854,
-4.04586790421435));
#69781=CARTESIAN_POINT('Ctrl Pts',(-0.580982052052641,0.53280461647316,
-4.02468577288849));
#69782=CARTESIAN_POINT('Ctrl Pts',(-0.741189311015275,0.0661142644363603,
-4.00350364156263));
#69783=CARTESIAN_POINT('Ctrl Pts',(-0.684298628680863,-0.296382410851875,
-3.98761704306823));
#69784=CARTESIAN_POINT('Ctrl Pts',(-0.458208148131325,-0.586325872950584,
-3.97173044457385));
#69785=CARTESIAN_POINT('Ctrl Pts',(-0.0092635365213895,-0.787816017268254,
-3.95054831324798));
#69786=CARTESIAN_POINT('Ctrl Pts',(0.625381488841516,-0.568854920649197,
-3.92407064909066));
#69787=CARTESIAN_POINT('Ctrl Pts',(0.8168820851143,0.220149395591204,-3.89229745210187));
#69788=CARTESIAN_POINT('Ctrl Pts',(0.350754382146573,0.705470988162975,
-3.86581978794455));
#69789=CARTESIAN_POINT('Ctrl Pts',(-0.138768819289989,0.730316662645527,
-3.84463765661869));
#69790=CARTESIAN_POINT('Ctrl Pts',(-0.587111491572448,0.526336984608081,
-3.82345552529284));
#69791=CARTESIAN_POINT('Ctrl Pts',(-0.787731543960356,0.0299986465066971,
-3.80227339396697));
#69792=CARTESIAN_POINT('Ctrl Pts',(-0.607726915303675,-0.429419011154302,
-3.78109126264112));
#69793=CARTESIAN_POINT('Ctrl Pts',(-0.32970225863993,-0.668882326963883,
-3.76520466414672));
#69794=CARTESIAN_POINT('Ctrl Pts',(0.0303174320013971,-0.743514350649698,
-3.74931806565233));
#69795=CARTESIAN_POINT('Ctrl Pts',(0.502934025139974,-0.606462906144964,
-3.72813593432647));
#69796=CARTESIAN_POINT('Ctrl Pts',(0.844909638687625,-0.0287337742940667,
-3.70165827016915));
#69797=CARTESIAN_POINT('Ctrl Pts',(0.480105778669465,0.696606444592673,
-3.66988507318036));
#69798=CARTESIAN_POINT('Ctrl Pts',(-0.189346584630163,0.764765207513764,
-3.64340740902304));
#69799=CARTESIAN_POINT('Ctrl Pts',(-0.578540580729554,0.466808321898773,
-3.62222527769718));
#69800=CARTESIAN_POINT('Ctrl Pts',(-0.788216509313215,0.0211011693712273,
-3.60104314637132));
#69801=CARTESIAN_POINT('Ctrl Pts',(-0.619821445054221,-0.487075230732692,
-3.57986101504546));
#69802=CARTESIAN_POINT('Ctrl Pts',(-0.185218436367416,-0.720712717769618,
-3.55867888371961));
#69803=CARTESIAN_POINT('Ctrl Pts',(0.181706561352431,-0.723249522805478,
-3.54279228522521));
#69804=CARTESIAN_POINT('Ctrl Pts',(0.504423484624682,-0.547073746824225,
-3.52690568673082));
#69805=CARTESIAN_POINT('Ctrl Pts',(0.775926926901616,-0.136664897769372,
-3.50572355540496));
#69806=CARTESIAN_POINT('Ctrl Pts',(0.662583245660023,0.525053682877346,
-3.47924589124763));
#69807=CARTESIAN_POINT('Ctrl Pts',(-0.0850176543603167,0.841744673762138,
-3.44747269425885));
#69808=CARTESIAN_POINT('Ctrl Pts',(-0.63939083797011,0.460323047494419,
-3.42099503010152));
#69809=CARTESIAN_POINT('Ctrl Pts',(-0.743147815742249,-0.0187226307543114,
-3.39981289877567));
#69810=CARTESIAN_POINT('Ctrl Pts',(-0.614431277810804,-0.494170749590194,
-3.37863076744981));
#69811=CARTESIAN_POINT('Ctrl Pts',(-0.157112882430159,-0.772487181975783,
-3.35744863612394));
#69812=CARTESIAN_POINT('Ctrl Pts',(0.325383332868861,-0.669222218262672,
-3.3362665047981));
#69813=CARTESIAN_POINT('Ctrl Pts',(0.606692403305564,-0.433625961455501,
-3.32037990630369));
#69814=CARTESIAN_POINT('Ctrl Pts',(0.738616463059989,-0.0904348207382206,
-3.30449330780931));
#69815=CARTESIAN_POINT('Ctrl Pts',(0.679874730541545,0.398133446151352,
-3.28331117648344));
#69816=CARTESIAN_POINT('Ctrl Pts',(0.165120091127291,0.829115964650634,
-3.25683351232612));
#69817=CARTESIAN_POINT('Ctrl Pts',(-0.609705129431059,0.586533675508332,
-3.22506031533734));
#69818=CARTESIAN_POINT('Ctrl Pts',(-0.785329064884318,-0.0630572088075564,
-3.19858265118001));
#69819=CARTESIAN_POINT('Ctrl Pts',(-0.554300299964595,-0.49534875633638,
-3.17740051985415));
#69820=CARTESIAN_POINT('Ctrl Pts',(-0.148411245134259,-0.774405983461156,
-3.1562183885283));
#69821=CARTESIAN_POINT('Ctrl Pts',(0.380321452818095,-0.690490040962752,
-3.13503625720243));
#69822=CARTESIAN_POINT('Ctrl Pts',(0.681226812577487,-0.299437339940724,
-3.11385412587658));
#69823=CARTESIAN_POINT('Ctrl Pts',(0.743124194941543,0.0622380717034434,
-3.09796752738218));
#69824=CARTESIAN_POINT('Ctrl Pts',(0.621509885269368,0.409216567134883,
-3.0820809288878));
#69825=CARTESIAN_POINT('Ctrl Pts',(0.260461624868717,0.743572210443643,
-3.06089879756193));
#69826=CARTESIAN_POINT('Ctrl Pts',(-0.410877211556822,0.738835465009447,
-3.03442113340462));
#69827=CARTESIAN_POINT('Ctrl Pts',(-0.844405646303706,0.0523564881392667,
-3.00264793641582));
#69828=CARTESIAN_POINT('Ctrl Pts',(-0.557750364160292,-0.556446298409586,
-2.9761702722585));
#69829=CARTESIAN_POINT('Ctrl Pts',(-0.101817380520569,-0.736377915182664,
-2.95498814093264));
#69830=CARTESIAN_POINT('Ctrl Pts',(0.38819590164287,-0.686319507846331,
-2.93380600960679));
#69831=CARTESIAN_POINT('Ctrl Pts',(0.736867919625537,-0.280083154025966,
-2.91262387828092));
#69832=CARTESIAN_POINT('Ctrl Pts',(0.713066307922928,0.212765437114261,
-2.89144174695507));
#69833=CARTESIAN_POINT('Ctrl Pts',(0.526112470273849,0.528500534814524,
-2.87555514846067));
#69834=CARTESIAN_POINT('Ctrl Pts',(0.208801790582379,0.714237039472746,
-2.85966854996628));
#69835=CARTESIAN_POINT('Ctrl Pts',(-0.282831813570063,0.735354374030618,
-2.83848641864042));
#69836=CARTESIAN_POINT('Ctrl Pts',(-0.791453765717036,0.297151247792696,
-2.8120087544831));
#69837=CARTESIAN_POINT('Ctrl Pts',(-0.677491328337421,-0.506722406636456,
-2.78023555749431));
#69838=CARTESIAN_POINT('Ctrl Pts',(-0.064895345870056,-0.785179308068587,
-2.753757893337));
#69839=CARTESIAN_POINT('Ctrl Pts',(0.399091755209997,-0.627172212289608,
-2.73257576201113));
#69840=CARTESIAN_POINT('Ctrl Pts',(0.740169947485737,-0.271806868459416,
-2.71139363068528));
#69841=CARTESIAN_POINT('Ctrl Pts',(0.742946469580542,0.263536425338524,
-2.69021149935941));
#69842=CARTESIAN_POINT('Ctrl Pts',(0.405758370113191,0.623773064349805,
-2.66902936803356));
#69843=CARTESIAN_POINT('Ctrl Pts',(0.0588719914752158,0.743398436436768,
-2.65314276953916));
#69844=CARTESIAN_POINT('Ctrl Pts',(-0.303216270831923,0.679553257227116,
-2.63725617104477));
#69845=CARTESIAN_POINT('Ctrl Pts',(-0.691605246616418,0.377388490849861,
-2.61607403971891));
#69846=CARTESIAN_POINT('Ctrl Pts',(-0.795600372028744,-0.285863560742109,
-2.58959637556159));
#69847=CARTESIAN_POINT('Ctrl Pts',(-0.188349690923361,-0.824794817690396,
-2.5578231785728));
#69848=CARTESIAN_POINT('Ctrl Pts',(0.45882509086868,-0.640466617181587,
-2.53134551441548));
#69849=CARTESIAN_POINT('Ctrl Pts',(0.710185521922345,-0.219671885767667,
-2.51016338308962));
#69850=CARTESIAN_POINT('Ctrl Pts',(0.740105571376498,0.271982109926758,
-2.48898125176376));
#69851=CARTESIAN_POINT('Ctrl Pts',(0.395666032677899,0.6818132403579,-2.4677991204379));
#69852=CARTESIAN_POINT('Ctrl Pts',(-0.0945357012105535,0.738102765149872,
-2.44661698911204));
#69853=CARTESIAN_POINT('Ctrl Pts',(-0.436369087788938,0.604722387463148,
-2.43073039061765));
#69854=CARTESIAN_POINT('Ctrl Pts',(-0.671019104572567,0.321661464281676,
-2.41484379212326));
#69855=CARTESIAN_POINT('Ctrl Pts',(-0.771438521446857,-0.160070290188984,
-2.3936616607974));
#69856=CARTESIAN_POINT('Ctrl Pts',(-0.421344828368112,-0.73291640924452,
-2.36718399664008));
#69857=CARTESIAN_POINT('Ctrl Pts',(0.390374518970285,-0.750579664192001,
-2.33541079965129));
#69858=CARTESIAN_POINT('Ctrl Pts',(0.764319887009418,-0.191136239516684,
-2.30893313549396));
#69859=CARTESIAN_POINT('Ctrl Pts',(0.683502010213621,0.292308424406099,
-2.28775100416811));
#69860=CARTESIAN_POINT('Ctrl Pts',(0.38803339177511,0.686411401253109,-2.26656887284225));
#69861=CARTESIAN_POINT('Ctrl Pts',(-0.139800436685434,0.77580715519062,
-2.24538674151639));
#69862=CARTESIAN_POINT('Ctrl Pts',(-0.549866856672383,0.501377233885317,
-2.22420461019053));
#69863=CARTESIAN_POINT('Ctrl Pts',(-0.724065013976115,0.178429263890927,
-2.20831801169614));
#69864=CARTESIAN_POINT('Ctrl Pts',(-0.719672927365281,-0.189218429130693,
-2.19243141320174));
#69865=CARTESIAN_POINT('Ctrl Pts',(-0.484361466229776,-0.621396701153967,
-2.17124928187589));
#69866=CARTESIAN_POINT('Ctrl Pts',(0.153310054633789,-0.831380751810275,
-2.14477161771856));
#69867=CARTESIAN_POINT('Ctrl Pts',(0.783429437513418,-0.319375036277522,
-2.11299842072978));
#69868=CARTESIAN_POINT('Ctrl Pts',(0.706290106391243,0.349102044320172,
-2.08652075657245));
#69869=CARTESIAN_POINT('Ctrl Pts',(0.331732388356717,0.665261479014068,
-2.06533862524659));
#69870=CARTESIAN_POINT('Ctrl Pts',(-0.148594596082589,0.774370822615237,
-2.04415649392074));
#69871=CARTESIAN_POINT('Ctrl Pts',(-0.608775250603796,0.500812937527267,
-2.02297436259487));
#69872=CARTESIAN_POINT('Ctrl Pts',(-0.743671235528029,0.026187481235811,
-2.00179223126902));
#69873=CARTESIAN_POINT('Ctrl Pts',(-0.667382320392564,-0.33272809485271,
-1.98590563277462));
#69874=CARTESIAN_POINT('Ctrl Pts',(-0.426037087450199,-0.610102562215694,
-1.97001903428023));
#69875=CARTESIAN_POINT('Ctrl Pts',(0.0330867987414303,-0.787175427666758,
-1.94883690295438));
#69876=CARTESIAN_POINT('Ctrl Pts',(0.655047859759172,-0.534425138590393,
-1.92235923879705));
#69877=CARTESIAN_POINT('Ctrl Pts',(0.803870926086962,0.263730224949567,
-1.89058604180827));
#69878=CARTESIAN_POINT('Ctrl Pts',(0.312335778526887,0.723300983814258,
-1.86410837765094));
#69879=CARTESIAN_POINT('Ctrl Pts',(-0.17781525043291,0.721803955141782,
-1.84292624632508));
#69880=CARTESIAN_POINT('Ctrl Pts',(-0.614548264760971,0.494025257635711,
-1.82174411499922));
#69881=CARTESIAN_POINT('Ctrl Pts',(-0.788205373773664,-0.0123771118085124,
-1.80056198367336));
#69882=CARTESIAN_POINT('Ctrl Pts',(-0.583771915529394,-0.461457518482905,
-1.77937985234751));
#69883=CARTESIAN_POINT('Ctrl Pts',(-0.293280337215025,-0.68563386036567,
-1.76349325385311));
#69884=CARTESIAN_POINT('Ctrl Pts',(0.070229816409773,-0.740810710770472,
-1.74760665535872));
#69885=CARTESIAN_POINT('Ctrl Pts',(0.534798374515875,-0.578559062489274,
-1.72642452403286));
#69886=CARTESIAN_POINT('Ctrl Pts',(0.845232871318611,0.0167128864931346,
-1.69994685987554));
#69887=CARTESIAN_POINT('Ctrl Pts',(0.441976637270261,0.7214005471769,-1.66817366288675));
#69888=CARTESIAN_POINT('Ctrl Pts',(-0.230171182371692,0.753484690315798,
-1.64169599872943));
#69889=CARTESIAN_POINT('Ctrl Pts',(-0.602790690129551,0.435043212609942,
-1.62051386740357));
#69890=CARTESIAN_POINT('Ctrl Pts',(-0.788211491123012,-0.0212877937884581,
-1.59933173607771));
#69891=CARTESIAN_POINT('Ctrl Pts',(-0.592750543967491,-0.519680379433986,
-1.57814960475185));
#69892=CARTESIAN_POINT('Ctrl Pts',(-0.14621995018756,-0.729624846679722,
-1.55696747342599));
#69893=CARTESIAN_POINT('Ctrl Pts',(0.220311161111685,-0.712439568641789,
-1.5410808749316));
#69894=CARTESIAN_POINT('Ctrl Pts',(0.533094129652703,-0.519175678585803,
-1.52519427643721));
#69895=CARTESIAN_POINT('Ctrl Pts',(0.782150020565167,-0.0947693806205724,
-1.50401214511135));
#69896=CARTESIAN_POINT('Ctrl Pts',(0.633409604628127,0.559901955789828,
-1.47753448095402));
#69897=CARTESIAN_POINT('Ctrl Pts',(-0.130129858152316,0.835959518982299,
-1.44576128396524));
#69898=CARTESIAN_POINT('Ctrl Pts',(-0.663204501309733,0.425297238619271,
-1.41928361980792));
#69899=CARTESIAN_POINT('Ctrl Pts',(-0.741067805959503,-0.0586320724109774,
-1.39810148848206));
#69900=CARTESIAN_POINT('Ctrl Pts',(-0.586986854985309,-0.526475979487392,
-1.3769193571562));
#69901=CARTESIAN_POINT('Ctrl Pts',(-0.115372668219765,-0.779814113472083,
-1.35573722583034));
#69902=CARTESIAN_POINT('Ctrl Pts',(0.360876909130024,-0.650769196552833,
-1.33455509450448));
#69903=CARTESIAN_POINT('Ctrl Pts',(0.629118624691168,-0.400395932476321,
-1.31866849601009));
#69904=CARTESIAN_POINT('Ctrl Pts',(0.742409083329817,-0.0506111578071527,
-1.30278189751569));
#69905=CARTESIAN_POINT('Ctrl Pts',(0.657496750844895,0.434094359329509,
-1.28159976618984));
#69906=CARTESIAN_POINT('Ctrl Pts',(0.120325095948475,0.836791371022327,
-1.25512210203251));
#69907=CARTESIAN_POINT('Ctrl Pts',(-0.640344202902728,0.552920789235428,
-1.22334890504373));
#69908=CARTESIAN_POINT('Ctrl Pts',(-0.780805578144866,-0.105169391329118,
-1.1968712408864));
#69909=CARTESIAN_POINT('Ctrl Pts',(-0.526879461855956,-0.524420866880043,
-1.17568910956055));
#69910=CARTESIAN_POINT('Ctrl Pts',(-0.106580489249386,-0.781262519396717,
-1.15450697823469));
#69911=CARTESIAN_POINT('Ctrl Pts',(0.416878567618402,-0.669053932058423,
-1.13332484690883));
#69912=CARTESIAN_POINT('Ctrl Pts',(0.696334082128771,-0.262395763668439,
-1.11214271558297));
#69913=CARTESIAN_POINT('Ctrl Pts',(0.738705715153232,0.102083363369506,
-1.09625611708858));
#69914=CARTESIAN_POINT('Ctrl Pts',(0.598620640920461,0.442024959215177,
-1.08036951859418));
#69915=CARTESIAN_POINT('Ctrl Pts',(0.220125949978788,0.756494848838535,
-1.05918738726833));
#69916=CARTESIAN_POINT('Ctrl Pts',(-0.449988238412121,0.715687440593429,
-1.032709723111));
#69917=CARTESIAN_POINT('Ctrl Pts',(-0.845999083354694,0.00690277646287119,
-1.00093652612222));
#69918=CARTESIAN_POINT('Ctrl Pts',(-0.527041180719297,-0.585615527082987,
-0.97445886196489));
#69919=CARTESIAN_POINT('Ctrl Pts',(-0.0620975683374578,-0.740785464862379,
-0.953276730639033));
#69920=CARTESIAN_POINT('Ctrl Pts',(0.424517514770048,-0.664466255393287,
-0.932094599313175));
#69921=CARTESIAN_POINT('Ctrl Pts',(0.75085469976088,-0.240079411839319,
-0.910912467987315));
#69922=CARTESIAN_POINT('Ctrl Pts',(0.700601975886072,0.25077791391973,-0.889730336661459));
#69923=CARTESIAN_POINT('Ctrl Pts',(0.496950799454161,0.556009936600838,
-0.873843738167064));
#69924=CARTESIAN_POINT('Ctrl Pts',(0.170117226641474,0.724425886826345,
-0.857957139672669));
#69925=CARTESIAN_POINT('Ctrl Pts',(-0.321940795819329,0.719092493469208,
-0.836775008346812));
#69926=CARTESIAN_POINT('Ctrl Pts',(-0.806278901509358,0.254189418164704,
-0.810297344189489));
#69927=CARTESIAN_POINT('Ctrl Pts',(-0.64928126104417,-0.542398323574931,
-0.778524147200702));
#69928=CARTESIAN_POINT('Ctrl Pts',(-0.0226063174085712,-0.787532161986483,
-0.752046483043379));
#69929=CARTESIAN_POINT('Ctrl Pts',(0.432219069236098,-0.604818889509744,
-0.730864351717523));
#69930=CARTESIAN_POINT('Ctrl Pts',(0.753707191550731,-0.231637635903656,
-0.709682220391664));
#69931=CARTESIAN_POINT('Ctrl Pts',(0.727710545460163,0.303081286331367,
-0.688500089065805));
#69932=CARTESIAN_POINT('Ctrl Pts',(0.371650701813931,0.644677009447944,
-0.667317957739948));
#69933=CARTESIAN_POINT('Ctrl Pts',(0.0188369557358222,0.745487971757124,
-0.651431359245553));
#69934=CARTESIAN_POINT('Ctrl Pts',(-0.339297064946969,0.662276556588206,
-0.635544760751158));
#69935=CARTESIAN_POINT('Ctrl Pts',(-0.710886586537695,0.339676541111478,
-0.614362629425303));
#69936=CARTESIAN_POINT('Ctrl Pts',(-0.779088508642335,-0.32820576176058,
-0.587884965267977));
#69937=CARTESIAN_POINT('Ctrl Pts',(-0.143753347590996,-0.833724816004507,
-0.556111768279191));
#69938=CARTESIAN_POINT('Ctrl Pts',(0.492580529297411,-0.614884040031596,
-0.529634104121868));
#69939=CARTESIAN_POINT('Ctrl Pts',(0.720964373963307,-0.181189335785351,
-0.508451972796009));
#69940=CARTESIAN_POINT('Ctrl Pts',(0.724419896865446,0.311362083290472,
-0.48726984147015));
#69941=CARTESIAN_POINT('Ctrl Pts',(0.358453864430568,0.702090987400412,
-0.466087710144294));
#69942=CARTESIAN_POINT('Ctrl Pts',(-0.134064441091513,0.731955841893754,
-0.444905578818434));
#69943=CARTESIAN_POINT('Ctrl Pts',(-0.468236154978809,0.580398310702801,
-0.429018980324041));
#69944=CARTESIAN_POINT('Ctrl Pts',(-0.687335322162944,0.285136193611118,
-0.413132381829648));
#69945=CARTESIAN_POINT('Ctrl Pts',(-0.761721915252497,-0.201295514566145,
-0.391950250503788));
#69946=CARTESIAN_POINT('Ctrl Pts',(-0.381348782508604,-0.754500870785961,
-0.365472586346466));
#69947=CARTESIAN_POINT('Ctrl Pts',(0.430145374627856,-0.728515393750025,
-0.333699389357679));
#69948=CARTESIAN_POINT('Ctrl Pts',(0.773488578129993,-0.149787584417332,
-0.307221725200355));
#69949=CARTESIAN_POINT('Ctrl Pts',(0.666803717585622,0.32861960324679,-0.286039593874498));
#69950=CARTESIAN_POINT('Ctrl Pts',(0.350590505112842,0.706266072815195,
-0.264857462548639));
#69951=CARTESIAN_POINT('Ctrl Pts',(-0.181300858414558,0.767185934044253,
-0.243675331222782));
#69952=CARTESIAN_POINT('Ctrl Pts',(-0.57600272772074,0.471087443825438,
-0.222493199896921));
#69953=CARTESIAN_POINT('Ctrl Pts',(-0.732635320889055,0.139292989541286,
-0.206606601402529));
#69954=CARTESIAN_POINT('Ctrl Pts',(-0.708413622199826,-0.227679344522623,
-0.190720002908134));
#69955=CARTESIAN_POINT('Ctrl Pts',(-0.450377756802535,-0.646399890802347,
-0.169537871582277));
#69956=CARTESIAN_POINT('Ctrl Pts',(0.197993874424786,-0.822205995966851,
-0.143060207424953));
#69957=CARTESIAN_POINT('Ctrl Pts',(0.799063290594735,-0.276348436002072,
-0.111287010436166));
#69958=CARTESIAN_POINT('Ctrl Pts',(0.687176416166241,0.385773860169478,
-0.0848093462788429));
#69959=CARTESIAN_POINT('Ctrl Pts',(0.294603052440389,0.683176174939641,
-0.0636272149529848));
#69960=CARTESIAN_POINT('Ctrl Pts',(-0.0669663409722705,0.742568911483241,
-0.0477406164585896));
#69961=CARTESIAN_POINT('Ctrl Pts',(-0.415015231537065,0.618962097253398,
-0.0318540179641988));
#69962=CARTESIAN_POINT('Ctrl Pts',(-0.578394000517792,0.436565751468206,
-0.0212629523012676));
#69963=CARTESIAN_POINT('Ctrl Pts',(-0.633489757429965,0.331175816864348,
-0.0159674194698027));
#69964=CARTESIAN_POINT('Ctrl Pts',(0.392888236737129,-0.550964357679868,
-11.9089));
#69965=CARTESIAN_POINT('Ctrl Pts',(0.484548909927025,-0.485601871403322,
-11.9036044671685));
#69966=CARTESIAN_POINT('Ctrl Pts',(0.634341446219948,-0.308693578393974,
-11.8930134015056));
#69967=CARTESIAN_POINT('Ctrl Pts',(0.705002038108303,0.0337351900899797,
-11.8771268030112));
#69968=CARTESIAN_POINT('Ctrl Pts',(0.602308840879945,0.365053324407907,
-11.8612402045168));
#69969=CARTESIAN_POINT('Ctrl Pts',(0.272406965382598,0.694503928448386,
-11.840058073191));
#69970=CARTESIAN_POINT('Ctrl Pts',(-0.363000708994007,0.713347601796957,
-11.8135804090336));
#69971=CARTESIAN_POINT('Ctrl Pts',(-0.796709301451907,0.0787753187535436,
-11.7818072120449));
#69972=CARTESIAN_POINT('Ctrl Pts',(-0.54757461974353,-0.506340519423678,
-11.7553295478875));
#69973=CARTESIAN_POINT('Ctrl Pts',(-0.121403177164881,-0.693866619017976,
-11.7341474165617));
#69974=CARTESIAN_POINT('Ctrl Pts',(0.225850498452994,-0.668875211131948,
-11.7182608180673));
#69975=CARTESIAN_POINT('Ctrl Pts',(0.516608588870761,-0.478872034799853,
-11.7023742195729));
#69976=CARTESIAN_POINT('Ctrl Pts',(0.742947756127913,-0.0702747149864332,
-11.681192088247));
#69977=CARTESIAN_POINT('Ctrl Pts',(0.616681960998304,0.420553527772077,
-11.6600099569212));
#69978=CARTESIAN_POINT('Ctrl Pts',(0.221462490922912,0.667971079462276,
-11.6388278255953));
#69979=CARTESIAN_POINT('Ctrl Pts',(-0.241001769318581,0.705818539717338,
-11.6176456942695));
#69980=CARTESIAN_POINT('Ctrl Pts',(-0.739034910876422,0.308639768144774,
-11.5911680301121));
#69981=CARTESIAN_POINT('Ctrl Pts',(-0.657912727899525,-0.455665328876149,
-11.5593948331233));
#69982=CARTESIAN_POINT('Ctrl Pts',(-0.0897337187244002,-0.740423380881239,
-11.532917168966));
#69983=CARTESIAN_POINT('Ctrl Pts',(0.356717037324203,-0.607439441065005,
-11.5117350376402));
#69984=CARTESIAN_POINT('Ctrl Pts',(0.605099039586646,-0.36361113891817,
-11.4958484391458));
#69985=CARTESIAN_POINT('Ctrl Pts',(0.703772576709861,-0.0305614200295496,
-11.4799618406514));
#69986=CARTESIAN_POINT('Ctrl Pts',(0.611744859212238,0.427384163050785,
-11.4587797093255));
#69987=CARTESIAN_POINT('Ctrl Pts',(0.197790656500237,0.719753643173289,
-11.4375975779997));
#69988=CARTESIAN_POINT('Ctrl Pts',(-0.263619000263347,0.652485296666156,
-11.4164154466738));
#69989=CARTESIAN_POINT('Ctrl Pts',(-0.640600438706306,0.381955634449409,
-11.395233315348));
#69990=CARTESIAN_POINT('Ctrl Pts',(-0.763085658381697,-0.243173825061882,
-11.3687556511906));
#69991=CARTESIAN_POINT('Ctrl Pts',(-0.206478220428704,-0.773205223454543,
-11.3369824542018));
#69992=CARTESIAN_POINT('Ctrl Pts',(0.410920283938739,-0.622433291638274,
-11.3105047900445));
#69993=CARTESIAN_POINT('Ctrl Pts',(0.665114014783227,-0.232063101779371,
-11.2893226587187));
#69994=CARTESIAN_POINT('Ctrl Pts',(0.696585389017661,0.11457124582531,-11.2734360602242));
#69995=CARTESIAN_POINT('Ctrl Pts',(0.55619304910803,0.432295255177504,-11.2575494617299));
#69996=CARTESIAN_POINT('Ctrl Pts',(0.189598103717612,0.721762795994409,
-11.236367330404));
#69997=CARTESIAN_POINT('Ctrl Pts',(-0.315180024953703,0.676629880018334,
-11.2151851990782));
#69998=CARTESIAN_POINT('Ctrl Pts',(-0.623315925700859,0.326663901421167,
-11.1940030677523));
#69999=CARTESIAN_POINT('Ctrl Pts',(-0.735519671514959,-0.123571168586822,
-11.1728209364264));
#70000=CARTESIAN_POINT('Ctrl Pts',(-0.424197719174421,-0.679330206520831,
-11.1463432722691));
#70001=CARTESIAN_POINT('Ctrl Pts',(0.343160473225332,-0.722994096502876,
-11.1145700752803));
#70002=CARTESIAN_POINT('Ctrl Pts',(0.716133365261885,-0.208402697353022,
-11.088092411123));
#70003=CARTESIAN_POINT('Ctrl Pts',(0.657170405500786,0.253686804061263,
-11.0669102797971));
#70004=CARTESIAN_POINT('Ctrl Pts',(0.456763012508479,0.538261390715488,
-11.0510236813027));
#70005=CARTESIAN_POINT('Ctrl Pts',(0.144077853390088,0.689544391419175,
-11.0351370828084));
#70006=CARTESIAN_POINT('Ctrl Pts',(-0.322724961404119,0.672857766501242,
-11.0139549514825));
#70007=CARTESIAN_POINT('Ctrl Pts',(-0.67824531273211,0.311688527808011,
-10.9927728201566));
#70008=CARTESIAN_POINT('Ctrl Pts',(-0.686552342337786,-0.154524849061646,
-10.9715906888308));
#70009=CARTESIAN_POINT('Ctrl Pts',(-0.480612243469802,-0.570325251330041,
-10.9504085575049));
#70010=CARTESIAN_POINT('Ctrl Pts',(0.116446449284972,-0.792384665988189,
-10.9239308933476));
#70011=CARTESIAN_POINT('Ctrl Pts',(0.729585741366676,-0.32891369683002,
-10.8921576963588));
#70012=CARTESIAN_POINT('Ctrl Pts',(0.680740265357369,0.304748047120233,
-10.8656800322015));
#70013=CARTESIAN_POINT('Ctrl Pts',(0.336664480573665,0.618778606564363,
-10.8444979008756));
#70014=CARTESIAN_POINT('Ctrl Pts',(-0.00030424207012357,0.705944531650651,
-10.8286113023812));
#70015=CARTESIAN_POINT('Ctrl Pts',(-0.336563415811402,0.618833550086267,
-10.8127247038868));
#70016=CARTESIAN_POINT('Ctrl Pts',(-0.681554107221738,0.303929224629296,
-10.791542572561));
#70017=CARTESIAN_POINT('Ctrl Pts',(-0.718724672271428,-0.20149761308359,
-10.7703604412351));
#70018=CARTESIAN_POINT('Ctrl Pts',(-0.423251854828125,-0.562218743134393,
-10.7491783099093));
#70019=CARTESIAN_POINT('Ctrl Pts',(0.0028831951113741,-0.745822169195642,
-10.7279961785834));
#70020=CARTESIAN_POINT('Ctrl Pts',(0.601706547663041,-0.528566424343903,
-10.7015185144261));
#70021=CARTESIAN_POINT('Ctrl Pts',(0.769006630385937,0.221604098315976,
-10.6697453174373));
#70022=CARTESIAN_POINT('Ctrl Pts',(0.321574591885842,0.672955022981378,
-10.64326765328));
#70023=CARTESIAN_POINT('Ctrl Pts',(-0.143965254934612,0.689567938489952,
-10.6220855219541));
#70024=CARTESIAN_POINT('Ctrl Pts',(-0.457226793531636,0.537867487033261,
-10.6061989234597));
#70025=CARTESIAN_POINT('Ctrl Pts',(-0.657128942689954,0.253794106027293,
-10.5903123249653));
#70026=CARTESIAN_POINT('Ctrl Pts',(-0.716223601331694,-0.20955363883752,
-10.5691301936395));
#70027=CARTESIAN_POINT('Ctrl Pts',(-0.417365376642559,-0.61884778822427,
-10.5479480623136));
#70028=CARTESIAN_POINT('Ctrl Pts',(0.0413549888341567,-0.702511076528755,
-10.5267659309878));
#70029=CARTESIAN_POINT('Ctrl Pts',(0.485007333141031,-0.566592364647785,
-10.5055837996619));
#70030=CARTESIAN_POINT('Ctrl Pts',(0.800783960244305,-0.0133522829404121,
-10.4791061355046));
#70031=CARTESIAN_POINT('Ctrl Pts',(0.442673841413548,0.666722914032616,
-10.4473329385158));
#70032=CARTESIAN_POINT('Ctrl Pts',(-0.190537863945514,0.721092229541751,
-10.4208552743584));
#70033=CARTESIAN_POINT('Ctrl Pts',(-0.556122470942101,0.432386093364394,
-10.3996731430326));
#70034=CARTESIAN_POINT('Ctrl Pts',(-0.696683883965076,0.113970786406134,
-10.3837865445382));
#70035=CARTESIAN_POINT('Ctrl Pts',(-0.6651518747368,-0.231954476372266,
-10.3678999460438));
#70036=CARTESIAN_POINT('Ctrl Pts',(-0.410243995550251,-0.623368942737406,
-10.346717814718));
#70037=CARTESIAN_POINT('Ctrl Pts',(0.082500557995093,-0.741862588718796,
-10.3255356833921));
#70038=CARTESIAN_POINT('Ctrl Pts',(0.48629264022718,-0.508676238690136,
-10.3043535520662));
#70039=CARTESIAN_POINT('Ctrl Pts',(0.736453075250717,-0.117880824698104,
-10.2831714207404));
#70040=CARTESIAN_POINT('Ctrl Pts',(0.618993813089344,0.508212449475007,
-10.2566937565831));
#70041=CARTESIAN_POINT('Ctrl Pts',(-0.0942027572610254,0.79473606593157,
-10.2249205595943));
#70042=CARTESIAN_POINT('Ctrl Pts',(-0.612027012017135,0.42626472721044,
-10.1984428954369));
#70043=CARTESIAN_POINT('Ctrl Pts',(-0.703777625297934,-0.0304465195329539,
-10.1772607641111));
#70044=CARTESIAN_POINT('Ctrl Pts',(-0.604785322978651,-0.364132513572057,
-10.1613741656167));
#70045=CARTESIAN_POINT('Ctrl Pts',(-0.356816358110809,-0.607381249430332,
-10.1454875671223));
#70046=CARTESIAN_POINT('Ctrl Pts',(0.0908551895918876,-0.740698527863264,
-10.1243054357964));
#70047=CARTESIAN_POINT('Ctrl Pts',(0.543127711937286,-0.512033916001494,
-10.1031233044706));
#70048=CARTESIAN_POINT('Ctrl Pts',(0.69994058004243,-0.0729056387183608,
-10.0819411731447));
#70049=CARTESIAN_POINT('Ctrl Pts',(0.637628208112178,0.386897000631171,
-10.0607590418189));
#70050=CARTESIAN_POINT('Ctrl Pts',(0.142798839180318,0.788062006426542,
-10.0342813776615));
#70051=CARTESIAN_POINT('Ctrl Pts',(-0.586274794331389,0.544758147712961,
-10.0025081806728));
#70052=CARTESIAN_POINT('Ctrl Pts',(-0.742424871886001,-0.071302108716839,
-9.97603051651542));
#70053=CARTESIAN_POINT('Ctrl Pts',(-0.516703214563073,-0.478798208519891,
-9.95484838518958));
#70054=CARTESIAN_POINT('Ctrl Pts',(-0.225239754106489,-0.669047701962083,
-9.93896178669518));
#70055=CARTESIAN_POINT('Ctrl Pts',(0.12122757218792,-0.693926344302069,
-9.92307518820078));
#70056=CARTESIAN_POINT('Ctrl Pts',(0.54874197779906,-0.505738288500843,
-9.90189305687493));
#70057=CARTESIAN_POINT('Ctrl Pts',(0.745433350289229,-0.0386725081502612,
-9.88071092554906));
#70058=CARTESIAN_POINT('Ctrl Pts',(0.580683923966688,0.397540222108045,
-9.85952879422322));
#70059=CARTESIAN_POINT('Ctrl Pts',(0.235535653683076,0.707659506204665,
-9.83834666289734));
#70060=CARTESIAN_POINT('Ctrl Pts',(-0.401313885472845,0.693094798545597,
-9.81186899874004));
#70061=CARTESIAN_POINT('Ctrl Pts',(-0.799503770929198,0.0356832487024724,
-9.78009580175124));
#70062=CARTESIAN_POINT('Ctrl Pts',(-0.519711826341081,-0.534956352110741,
-9.75361813759391));
#70063=CARTESIAN_POINT('Ctrl Pts',(-0.0838752645359608,-0.69942467530156,
-9.73243600626807));
#70064=CARTESIAN_POINT('Ctrl Pts',(0.261433978866206,-0.655751514695071,
-9.71654940777366));
#70065=CARTESIAN_POINT('Ctrl Pts',(0.541613442530161,-0.450427324266235,
-9.70066280927928));
#70066=CARTESIAN_POINT('Ctrl Pts',(0.745637002453177,-0.0302396300775194,
-9.6794806779534));
#70067=CARTESIAN_POINT('Ctrl Pts',(0.593197195641168,0.453082254887026,
-9.65829854662756));
#70068=CARTESIAN_POINT('Ctrl Pts',(0.185243328053068,0.678908651556959,
-9.6371164153017));
#70069=CARTESIAN_POINT('Ctrl Pts',(-0.278581983793115,0.691846152828526,
-9.61593428397583));
#70070=CARTESIAN_POINT('Ctrl Pts',(-0.754554355140179,0.268478974192128,
-9.58945661981852));
#70071=CARTESIAN_POINT('Ctrl Pts',(-0.632474069342684,-0.490363258796042,
-9.55768342282974));
#70072=CARTESIAN_POINT('Ctrl Pts',(-0.0498142904822183,-0.744175528733757,
-9.5312057586724));
#70073=CARTESIAN_POINT('Ctrl Pts',(0.388845301867087,-0.587391919962783,
-9.51002362734656));
#70074=CARTESIAN_POINT('Ctrl Pts',(0.623764909652236,-0.33056786265037,
-9.49413702885215));
#70075=CARTESIAN_POINT('Ctrl Pts',(0.704398011625223,0.00730320432709524,
-9.47825043035776));
#70076=CARTESIAN_POINT('Ctrl Pts',(0.587893373397589,0.459641551831196,
-9.45706829903191));
#70077=CARTESIAN_POINT('Ctrl Pts',(0.158825559311775,0.729342775599619,
-9.43588616770604));
#70078=CARTESIAN_POINT('Ctrl Pts',(-0.298302397103462,0.637375656602442,
-9.4147040363802));
#70079=CARTESIAN_POINT('Ctrl Pts',(-0.660200912976761,0.346978061817164,
-9.39352190505432));
#70080=CARTESIAN_POINT('Ctrl Pts',(-0.748914914372129,-0.283830381522591,
-9.36704424089701));
#70081=CARTESIAN_POINT('Ctrl Pts',(-0.164628083532023,-0.783183993759156,
-9.33527104390821));
#70082=CARTESIAN_POINT('Ctrl Pts',(0.443775836884319,-0.599451155391359,
-9.30879337975089));
#70083=CARTESIAN_POINT('Ctrl Pts',(0.676623900661522,-0.195984778682572,
-9.28761124842504));
#70084=CARTESIAN_POINT('Ctrl Pts',(0.689421792526712,0.151839936511941,
-9.27172464993064));
#70085=CARTESIAN_POINT('Ctrl Pts',(0.532157948497518,0.461560194802287,
-9.25583805143624));
#70086=CARTESIAN_POINT('Ctrl Pts',(0.150536857936622,0.730908769311981,
-9.2346559201104));
#70087=CARTESIAN_POINT('Ctrl Pts',(-0.351086430223958,0.658714476175113,
-9.21347378878452));
#70088=CARTESIAN_POINT('Ctrl Pts',(-0.639970023186198,0.292695092494087,
-9.19229165745868));
#70089=CARTESIAN_POINT('Ctrl Pts',(-0.72781616183648,-0.162919168446685,
-9.17110952613282));
#70090=CARTESIAN_POINT('Ctrl Pts',(-0.387077784779294,-0.701144794585703,
-9.14463186197549));
#70091=CARTESIAN_POINT('Ctrl Pts',(0.381518042580854,-0.703508036310348,
-9.11285866498672));
#70092=CARTESIAN_POINT('Ctrl Pts',(0.726298025262084,-0.169616802242028,
-9.08638100082937));
#70093=CARTESIAN_POINT('Ctrl Pts',(0.642587744543107,0.288636323051471,
-9.06519886950353));
#70094=CARTESIAN_POINT('Ctrl Pts',(0.427177008054458,0.562029872978596,
-9.04931227100912));
#70095=CARTESIAN_POINT('Ctrl Pts',(0.106813790756512,0.696290679012175,
-9.03342567251474));
#70096=CARTESIAN_POINT('Ctrl Pts',(-0.358417752115536,0.654542351282965,
-9.01224354118889));
#70097=CARTESIAN_POINT('Ctrl Pts',(-0.69401526503328,0.274789473071372,
-8.99106140986302));
#70098=CARTESIAN_POINT('Ctrl Pts',(-0.677256151716331,-0.191196633624784,
-8.96987927853717));
#70099=CARTESIAN_POINT('Ctrl Pts',(-0.449268676104613,-0.595329049811071,
-8.9486971472113));
#70100=CARTESIAN_POINT('Ctrl Pts',(0.158860648830693,-0.784981865202862,
-8.92221948305397));
#70101=CARTESIAN_POINT('Ctrl Pts',(0.746207180183646,-0.289230735244962,
-8.89044628606521));
#70102=CARTESIAN_POINT('Ctrl Pts',(0.663379532687123,0.340890417457322,
-8.86396862190785));
#70103=CARTESIAN_POINT('Ctrl Pts',(0.302925054514254,0.635976688070566,
-8.84278649058203));
#70104=CARTESIAN_POINT('Ctrl Pts',(-0.0382410075393195,0.704908078881972,
-8.8268998920876));
#70105=CARTESIAN_POINT('Ctrl Pts',(-0.36933296774987,0.599852527299907,
-8.81101329359323));
#70106=CARTESIAN_POINT('Ctrl Pts',(-0.696902296093017,0.266863568804114,
-8.78983116226737));
#70107=CARTESIAN_POINT('Ctrl Pts',(-0.706857692602032,-0.239830450567451,
-8.7686490309415));
#70108=CARTESIAN_POINT('Ctrl Pts',(-0.392426815119199,-0.584151729024632,
-8.74746689961565));
#70109=CARTESIAN_POINT('Ctrl Pts',(0.0429592438378583,-0.744589500494483,
-8.72628476828979));
#70110=CARTESIAN_POINT('Ctrl Pts',(0.629242040014653,-0.495467142727417,
-8.69980710413247));
#70111=CARTESIAN_POINT('Ctrl Pts',(0.755986477075477,0.262610015892347,
-8.66803390714367));
#70112=CARTESIAN_POINT('Ctrl Pts',(0.284945549871296,0.689263893375359,
-8.64155624298637));
#70113=CARTESIAN_POINT('Ctrl Pts',(-0.18081435535875,0.680834859064861,
-8.62037411166049));
#70114=CARTESIAN_POINT('Ctrl Pts',(-0.485470897563107,0.512519055206698,
-8.60448751316611));
#70115=CARTESIAN_POINT('Ctrl Pts',(-0.669818183142776,0.218113495928887,
-8.58860091467172));
#70116=CARTESIAN_POINT('Ctrl Pts',(-0.703927307830937,-0.247740428562784,
-8.56741878334585));
#70117=CARTESIAN_POINT('Ctrl Pts',(-0.383505618497739,-0.64038260687711,
-8.54623665202));
#70118=CARTESIAN_POINT('Ctrl Pts',(0.0790479225720012,-0.699273532806809,
-8.52505452069413));
#70119=CARTESIAN_POINT('Ctrl Pts',(0.514754958365451,-0.539709508639534,
-8.50387238936828));
#70120=CARTESIAN_POINT('Ctrl Pts',(0.800344359486549,0.0297008532257883,
-8.47739472521096));
#70121=CARTESIAN_POINT('Ctrl Pts',(0.406204720035274,0.689548620032724,
-8.44562152822216));
#70122=CARTESIAN_POINT('Ctrl Pts',(-0.229013770145407,0.709810801683236,
-8.41914386406485));
#70123=CARTESIAN_POINT('Ctrl Pts',(-0.578555136750526,0.401875465985733,
-8.39796173273899));
#70124=CARTESIAN_POINT('Ctrl Pts',(-0.701801911913352,0.0763665552808169,
-8.3820751342446));
#70125=CARTESIAN_POINT('Ctrl Pts',(-0.651725567877458,-0.267364320263228,
-8.3661885357502));
#70126=CARTESIAN_POINT('Ctrl Pts',(-0.376151562716211,-0.644514527780979,
-8.34500640442435));
#70127=CARTESIAN_POINT('Ctrl Pts',(0.122248771729135,-0.736357033252738,
-8.32382427309847));
#70128=CARTESIAN_POINT('Ctrl Pts',(0.512926016390591,-0.481808000615124,
-8.30264214177264));
#70129=CARTESIAN_POINT('Ctrl Pts',(0.741723760032622,-0.0781337614659248,
-8.28146001044675));
#70130=CARTESIAN_POINT('Ctrl Pts',(0.590788201416899,0.540742577860168,
-8.25498234628945));
#70131=CARTESIAN_POINT('Ctrl Pts',(-0.136775462740103,0.788525235335051,
-8.22320914930065));
#70132=CARTESIAN_POINT('Ctrl Pts',(-0.634049934714981,0.39275865539838,
-8.19673148514334));
#70133=CARTESIAN_POINT('Ctrl Pts',(-0.701124468604536,-0.0682232800858731,
-8.17554935381747));
#70134=CARTESIAN_POINT('Ctrl Pts',(-0.584343046747153,-0.396107280984521,
-8.15966275532308));
#70135=CARTESIAN_POINT('Ctrl Pts',(-0.323660302086688,-0.625678754975878,
-8.14377615682868));
#70136=CARTESIAN_POINT('Ctrl Pts',(0.130528774517201,-0.734745679590988,
-8.12259402550284));
#70137=CARTESIAN_POINT('Ctrl Pts',(0.569859400741034,-0.482106529718409,
-8.10141189417698));
#70138=CARTESIAN_POINT('Ctrl Pts',(0.702847075744717,-0.0351857338159052,
-8.08022976285111));
#70139=CARTESIAN_POINT('Ctrl Pts',(0.615915117961009,0.420603837767584,
-8.05904763152526));
#70140=CARTESIAN_POINT('Ctrl Pts',(0.100242323565696,0.794597200479857,
-8.03256996736792));
#70141=CARTESIAN_POINT('Ctrl Pts',(-0.614702723239511,0.512464765627743,
-8.00079677037916));
#70142=CARTESIAN_POINT('Ctrl Pts',(-0.737520304544937,-0.111096721312356,
-7.9743191062218));
#70143=CARTESIAN_POINT('Ctrl Pts',(-0.490226125422572,-0.505873781070776,
-7.95313697489597));
#70144=CARTESIAN_POINT('Ctrl Pts',(-0.188959895740458,-0.680185218989984,
-7.93725037640156));
#70145=CARTESIAN_POINT('Ctrl Pts',(0.158343748144318,-0.68640888178885,
-7.92136377790718));
#70146=CARTESIAN_POINT('Ctrl Pts',(0.57512722912829,-0.475518290888796,
-7.9001816465813));
#70147=CARTESIAN_POINT('Ctrl Pts',(0.746434431978506,0.00144269434815235,
-7.87899951525548));
#70148=CARTESIAN_POINT('Ctrl Pts',(0.558481156467344,0.428171514253297,
-7.85781738392959));
#70149=CARTESIAN_POINT('Ctrl Pts',(0.197165933085699,0.719294526399437,
-7.83663525260375));
#70150=CARTESIAN_POINT('Ctrl Pts',(-0.437980644554784,0.670526799941397,
-7.81015758844643));
#70151=CARTESIAN_POINT('Ctrl Pts',(-0.80026607813319,-0.00733335920928448,
-7.77838439145762));
#70152=CARTESIAN_POINT('Ctrl Pts',(-0.490212471272208,-0.562112456819458,
-7.75190672730032));
#70153=CARTESIAN_POINT('Ctrl Pts',(-0.0461672328563757,-0.702921420239883,
-7.73072459597445));
#70154=CARTESIAN_POINT('Ctrl Pts',(0.296296052364626,-0.640754573673755,
-7.71483799748007));
#70155=CARTESIAN_POINT('Ctrl Pts',(0.565036603409811,-0.420670336941072,
-7.69895139898565));
#70156=CARTESIAN_POINT('Ctrl Pts',(0.746184610028158,0.00987433095006524,
-7.67776926765981));
#70157=CARTESIAN_POINT('Ctrl Pts',(0.56799153737738,0.484305746484325,-7.65658713633396));
#70158=CARTESIAN_POINT('Ctrl Pts',(0.148491341379806,0.687882525786409,
-7.63540500500808));
#70159=CARTESIAN_POINT('Ctrl Pts',(-0.315358990972195,0.675875526773047,
-7.61422287368224));
#70160=CARTESIAN_POINT('Ctrl Pts',(-0.767891973600488,0.227541537579893,
-7.5877452095249));
#70161=CARTESIAN_POINT('Ctrl Pts',(-0.605208187534785,-0.523643603712323,
-7.55597201253612));
#70162=CARTESIAN_POINT('Ctrl Pts',(-0.00975058277995205,-0.745777183371727,
-7.5294943483788));
#70163=CARTESIAN_POINT('Ctrl Pts',(0.419849643624006,-0.565646721170082,
-7.50831221705293));
#70164=CARTESIAN_POINT('Ctrl Pts',(0.640628155804832,-0.296569284182963,
-7.49242561855854));
#70165=CARTESIAN_POINT('Ctrl Pts',(0.702987671893402,0.0451467467366845,
-7.47653902006416));
#70166=CARTESIAN_POINT('Ctrl Pts',(0.562342884997569,0.490570539624217,
-7.45535688873828));
#70167=CARTESIAN_POINT('Ctrl Pts',(0.119401435125199,0.736824090200709,
-7.43417475741245));
#70168=CARTESIAN_POINT('Ctrl Pts',(-0.332123683053873,0.620423973506661,
-7.41299262608657));
#70169=CARTESIAN_POINT('Ctrl Pts',(-0.677893386628627,0.310997712600778,
-7.39181049476072));
#70170=CARTESIAN_POINT('Ctrl Pts',(-0.732579775894945,-0.323666659379656,
-7.3653328306034));
#70171=CARTESIAN_POINT('Ctrl Pts',(-0.122302166900868,-0.790899332367473,
-7.3335596336146));
#70172=CARTESIAN_POINT('Ctrl Pts',(0.475348861974375,-0.574736583594672,
-7.30708196945728));
#70173=CARTESIAN_POINT('Ctrl Pts',(0.686178318089926,-0.159340052105395,
-7.28589983813143));
#70174=CARTESIAN_POINT('Ctrl Pts',(0.680265741730897,0.18866980404402,-7.27001323963702));
#70175=CARTESIAN_POINT('Ctrl Pts',(0.50658489163482,0.489491208442347,-7.25412664114265));
#70176=CARTESIAN_POINT('Ctrl Pts',(0.111040555138311,0.737942389193872,
-7.23294450981677));
#70177=CARTESIAN_POINT('Ctrl Pts',(-0.385978182755204,0.638895363144113,
-7.21176237849093));
#70178=CARTESIAN_POINT('Ctrl Pts',(-0.654774583609806,0.257880383910193,
-7.19058024716506));
#70179=CARTESIAN_POINT('Ctrl Pts',(-0.718009236529222,-0.201796325874554,
-7.16939811583921));
#70180=CARTESIAN_POINT('Ctrl Pts',(-0.348839181256874,-0.720933048253655,
-7.14292045168188));
#70181=CARTESIAN_POINT('Ctrl Pts',(0.418773010672415,-0.681988811858619,
-7.1111472546931));
#70182=CARTESIAN_POINT('Ctrl Pts',(0.7343636570957,-0.130340708297302,-7.08466959053577));
#70183=CARTESIAN_POINT('Ctrl Pts',(0.626147981225155,0.322751672388126,
-7.06348745920991));
#70184=CARTESIAN_POINT('Ctrl Pts',(0.396356446240715,0.58417406811166,-7.04760086071553));
#70185=CARTESIAN_POINT('Ctrl Pts',(0.069241032314998,0.70102466077804,-7.03171426222112));
#70186=CARTESIAN_POINT('Ctrl Pts',(-0.393074702260597,0.634335284449263,
-7.01053213089527));
#70187=CARTESIAN_POINT('Ctrl Pts',(-0.707779487537858,0.237096266589547,
-6.98934999956941));
#70188=CARTESIAN_POINT('Ctrl Pts',(-0.666002665755798,-0.227315852841898,
-6.96816786824355));
#70189=CARTESIAN_POINT('Ctrl Pts',(-0.416626705641162,-0.618612325309093,
-6.9469857369177));
#70190=CARTESIAN_POINT('Ctrl Pts',(0.200815735222948,-0.77531043778035,
-6.92050807276037));
#70191=CARTESIAN_POINT('Ctrl Pts',(0.760672052637908,-0.248711886132582,
-6.88873487577159));
#70192=CARTESIAN_POINT('Ctrl Pts',(0.644101608620266,0.376047601873901,
-6.86225721161426));
#70193=CARTESIAN_POINT('Ctrl Pts',(0.268310163838186,0.651336773415186,
-6.8410750802884));
#70194=CARTESIAN_POINT('Ctrl Pts',(-0.07606725508181,0.701834415681397,
-6.825188481794));
#70195=CARTESIAN_POINT('Ctrl Pts',(-0.401035133744832,0.579137908513486,
-6.80930188329962));
#70196=CARTESIAN_POINT('Ctrl Pts',(-0.710236411541561,0.229026667389746,
-6.78811975197375));
#70197=CARTESIAN_POINT('Ctrl Pts',(-0.692947868044057,-0.277470169173608,
-6.76693762064789));
#70198=CARTESIAN_POINT('Ctrl Pts',(-0.360467647394768,-0.604396494803816,
-6.74575548932204));
#70199=CARTESIAN_POINT('Ctrl Pts',(0.0829111387628172,-0.741204940581804,
-6.72457335799618));
#70200=CARTESIAN_POINT('Ctrl Pts',(0.654958999580732,-0.460935942740932,
-6.69809569383886));
#70201=CARTESIAN_POINT('Ctrl Pts',(0.740781494882939,0.3028569808165,-6.66632249685007));
#70202=CARTESIAN_POINT('Ctrl Pts',(0.247493004655936,0.703580765593753,
-6.63984483269275));
#70203=CARTESIAN_POINT('Ctrl Pts',(-0.217140895580519,0.670134141730119,
-6.61866270136689));
#70204=CARTESIAN_POINT('Ctrl Pts',(-0.512311972790511,0.485689424288953,
-6.6027761028725));
#70205=CARTESIAN_POINT('Ctrl Pts',(-0.680571624160622,0.181802529862302,
-6.5868895043781));
#70206=CARTESIAN_POINT('Ctrl Pts',(-0.689596638591978,-0.285211239524086,
-6.56570737305225));
#70207=CARTESIAN_POINT('Ctrl Pts',(-0.34853751448554,-0.660066695636425,
-6.54452524172639));
#70208=CARTESIAN_POINT('Ctrl Pts',(0.116512404375386,-0.694015063241657,
-6.52334311040052));
#70209=CARTESIAN_POINT('Ctrl Pts',(0.543014923912942,-0.511266870913038,
-6.50216097907468));
#70210=CARTESIAN_POINT('Ctrl Pts',(0.797591731359379,0.0726681501291486,
-6.47568331491733));
#70211=CARTESIAN_POINT('Ctrl Pts',(0.368561656490527,0.710381509762504,
-6.44391011792857));
#70212=CARTESIAN_POINT('Ctrl Pts',(-0.266827825705201,0.696477986286548,
-6.41743245377122));
#70213=CARTESIAN_POINT('Ctrl Pts',(-0.599315746240538,0.370203414794835,
-6.39625032244539));
#70214=CARTESIAN_POINT('Ctrl Pts',(-0.704891729413253,0.0385415976514491,
-6.38036372395098));
#70215=CARTESIAN_POINT('Ctrl Pts',(-0.636415707053117,-0.30200142601737,
-6.36447712545659));
#70216=CARTESIAN_POINT('Ctrl Pts',(-0.340972135963656,-0.663797545482861,
-6.34329499413074));
#70217=CARTESIAN_POINT('Ctrl Pts',(0.161643869936548,-0.728723180265365,
-6.32211286280486));
#70218=CARTESIAN_POINT('Ctrl Pts',(0.538076797651925,-0.453547551601197,
-6.30093073147902));
#70219=CARTESIAN_POINT('Ctrl Pts',(0.744851349578635,-0.038160346185337,
-6.27974860015315));
#70220=CARTESIAN_POINT('Ctrl Pts',(0.560874095982173,0.57170878506611,-6.25327093599583));
#70221=CARTESIAN_POINT('Ctrl Pts',(-0.178950953192254,0.780037574273926,
-6.22149773900705));
#70222=CARTESIAN_POINT('Ctrl Pts',(-0.654243696240302,0.358114047435898,
-6.19502007484972));
#70223=CARTESIAN_POINT('Ctrl Pts',(-0.696440513048951,-0.105798096922755,
-6.17383794352387));
#70224=CARTESIAN_POINT('Ctrl Pts',(-0.562221864267348,-0.426947701728367,
-6.15795134502947));
#70225=CARTESIAN_POINT('Ctrl Pts',(-0.289550464019102,-0.642148606418798,
-6.14206474653509));
#70226=CARTESIAN_POINT('Ctrl Pts',(0.169783162631269,-0.726713697646756,
-6.1208826152092));
#70227=CARTESIAN_POINT('Ctrl Pts',(0.595024636138863,-0.450700878954778,
-6.09970048388339));
#70228=CARTESIAN_POINT('Ctrl Pts',(0.70362826836473,0.00253654546368757,
-6.07851835255749));
#70229=CARTESIAN_POINT('Ctrl Pts',(0.592641591588357,0.453327123043412,
-6.05733622123166));
#70230=CARTESIAN_POINT('Ctrl Pts',(0.0569329064749938,0.798344967018745,
-6.03085855707431));
#70231=CARTESIAN_POINT('Ctrl Pts',(-0.640560403072364,0.479540489150726,
-5.99908536008555));
#70232=CARTESIAN_POINT('Ctrl Pts',(-0.74990911679165,-0.278210377237643,
-5.96731216309674));
#70233=CARTESIAN_POINT('Ctrl Pts',(-0.172598743972036,-0.781008560151051,
-5.93553896610797));
#70234=CARTESIAN_POINT('Ctrl Pts',(0.562958377491915,-0.568642748947718,
-5.90376576911917));
#70235=CARTESIAN_POINT('Ctrl Pts',(0.78296431633078,0.166020846752831,-5.87199257213039));
#70236=CARTESIAN_POINT('Ctrl Pts',(0.367652295433943,0.649277541756489,
-5.84551490797305));
#70237=CARTESIAN_POINT('Ctrl Pts',(-0.094108426135513,0.697311105773554,
-5.82433277664721));
#70238=CARTESIAN_POINT('Ctrl Pts',(-0.528139077188013,0.527498545068882,
-5.80315064532134));
#70239=CARTESIAN_POINT('Ctrl Pts',(-0.743143845220938,0.0683838136603718,
-5.78196851399549));
#70240=CARTESIAN_POINT('Ctrl Pts',(-0.596304988912091,-0.374986218597206,
-5.76078638266963));
#70241=CARTESIAN_POINT('Ctrl Pts',(-0.345699947738929,-0.615523607024695,
-5.74489978417524));
#70242=CARTESIAN_POINT('Ctrl Pts',(-0.009161937171944,-0.704371126917918,
-5.72901318568084));
#70243=CARTESIAN_POINT('Ctrl Pts',(0.44456117416937,-0.598870476365504,
-5.70783105435499));
#70244=CARTESIAN_POINT('Ctrl Pts',(0.797221488507143,-0.0701424207596342,
-5.68135339019766));
#70245=CARTESIAN_POINT('Ctrl Pts',(0.489274781214441,0.634066932534056,
-5.64958019320888));
#70246=CARTESIAN_POINT('Ctrl Pts',(-0.140080473677338,0.732555257905117,
-5.62310252905155));
#70247=CARTESIAN_POINT('Ctrl Pts',(-0.523138810580797,0.470699274058183,
-5.60192039772569));
#70248=CARTESIAN_POINT('Ctrl Pts',(-0.744016619254324,0.0600456860856954,
-5.58073826639983));
#70249=CARTESIAN_POINT('Ctrl Pts',(-0.610687717749323,-0.428893565214981,
-5.55955613507398));
#70250=CARTESIAN_POINT('Ctrl Pts',(-0.211749126753277,-0.671857217583966,
-5.53837400374811));
#70251=CARTESIAN_POINT('Ctrl Pts',(0.134970931816977,-0.692921822797631,
-5.52248740525373));
#70252=CARTESIAN_POINT('Ctrl Pts',(0.448993413533046,-0.542802769541158,
-5.50660080675932));
#70253=CARTESIAN_POINT('Ctrl Pts',(0.726520552090549,-0.168661084255895,
-5.48541867543347));
#70254=CARTESIAN_POINT('Ctrl Pts',(0.65304184941208,0.462618554495975,-5.45894101127615));
#70255=CARTESIAN_POINT('Ctrl Pts',(-0.0375440690826849,0.800014795396159,
-5.42716781428736));
#70256=CARTESIAN_POINT('Ctrl Pts',(-0.580989448745449,0.467664710376834,
-5.40069015013004));
#70257=CARTESIAN_POINT('Ctrl Pts',(-0.703439922458687,0.0201078062197571,
-5.37950801880418));
#70258=CARTESIAN_POINT('Ctrl Pts',(-0.605953346375472,-0.435874963388025,
-5.35832588747833));
#70259=CARTESIAN_POINT('Ctrl Pts',(-0.187815285885199,-0.722228768117197,
-5.33714375615245));
#70260=CARTESIAN_POINT('Ctrl Pts',(0.273535159807509,-0.649159773727578,
-5.31596162482661));
#70261=CARTESIAN_POINT('Ctrl Pts',(0.551438224564908,-0.44076485660649,
-5.3000750263322));
#70262=CARTESIAN_POINT('Ctrl Pts',(0.693603344904396,-0.123062327230168,
-5.28418842783782));
#70263=CARTESIAN_POINT('Ctrl Pts',(0.662930453897055,0.341762921281637,
-5.26300629651195));
#70264=CARTESIAN_POINT('Ctrl Pts',(0.198265258367223,0.775351830664549,
-5.23652863235464));
#70265=CARTESIAN_POINT('Ctrl Pts',(-0.546507260958737,0.58545968961291,
-5.20475543536584));
#70266=CARTESIAN_POINT('Ctrl Pts',(-0.745568705556984,-0.0196551817061931,
-5.17827777120853));
#70267=CARTESIAN_POINT('Ctrl Pts',(-0.549172285849032,-0.440047552208631,
-5.15709563988267));
#70268=CARTESIAN_POINT('Ctrl Pts',(-0.179687362077751,-0.724485261766983,
-5.1359135085568));
#70269=CARTESIAN_POINT('Ctrl Pts',(0.324385456870523,-0.67205881440986,
-5.11473137723096));
#70270=CARTESIAN_POINT('Ctrl Pts',(0.628721139150488,-0.317709969564103,
-5.09354924590509));
#70271=CARTESIAN_POINT('Ctrl Pts',(0.705631348411274,0.0210279449736901,
-5.0776626474107));
#70272=CARTESIAN_POINT('Ctrl Pts',(0.608322795378933,0.355208830188862,
-5.0617760489163));
#70273=CARTESIAN_POINT('Ctrl Pts',(0.284038448676206,0.689638195560499,
-5.04059391759044));
#70274=CARTESIAN_POINT('Ctrl Pts',(-0.350809927077043,0.719313540142401,
-5.01411625343312));
#70275=CARTESIAN_POINT('Ctrl Pts',(-0.795541563970066,0.0924491992412632,
-4.98234305644434));
#70276=CARTESIAN_POINT('Ctrl Pts',(-0.555541790830451,-0.497626706998958,
-4.95586539228701));
#70277=CARTESIAN_POINT('Ctrl Pts',(-0.133708223738798,-0.690908212899286,
-4.93468326096116));
#70278=CARTESIAN_POINT('Ctrl Pts',(0.332041232394348,-0.668517062310377,
-4.91350112963529));
#70279=CARTESIAN_POINT('Ctrl Pts',(0.682302518044435,-0.302245344918345,
-4.89231899830944));
#70280=CARTESIAN_POINT('Ctrl Pts',(0.684875796890799,0.164848531713828,
-4.87113686698358));
#70281=CARTESIAN_POINT('Ctrl Pts',(0.524213242357612,0.472819469636789,
-4.85525026848919));
#70282=CARTESIAN_POINT('Ctrl Pts',(0.23371275114266,0.664536143768718,-4.83936366999479));
#70283=CARTESIAN_POINT('Ctrl Pts',(-0.229947459772284,0.709508877214857,
-4.81818153866894));
#70284=CARTESIAN_POINT('Ctrl Pts',(-0.733033467760661,0.321156518088531,
-4.79170387451161));
#70285=CARTESIAN_POINT('Ctrl Pts',(-0.666201687207296,-0.444531828339013,
-4.75993067752283));
#70286=CARTESIAN_POINT('Ctrl Pts',(-0.101288996576348,-0.738917830377844,
-4.7334530133655));
#70287=CARTESIAN_POINT('Ctrl Pts',(0.345349925440383,-0.613160237413833,
-4.71227088203965));
#70288=CARTESIAN_POINT('Ctrl Pts',(0.685844918037705,-0.294589869160345,
-4.69108875071378));
#70289=CARTESIAN_POINT('Ctrl Pts',(0.715703969576795,0.211321562048467,
-4.66990661938793));
#70290=CARTESIAN_POINT('Ctrl Pts',(0.415290946306725,0.569002043485502,
-4.64872448806207));
#70291=CARTESIAN_POINT('Ctrl Pts',(0.0934696898535255,0.699729370120608,
-4.63283788956767));
#70292=CARTESIAN_POINT('Ctrl Pts',(-0.252055370210626,0.657797861633536,
-4.61695129107328));
#70293=CARTESIAN_POINT('Ctrl Pts',(-0.634566132837756,0.391924105099125,
-4.59576915974741));
#70294=CARTESIAN_POINT('Ctrl Pts',(-0.766612827327275,-0.229748442748258,
-4.56929149559011));
#70295=CARTESIAN_POINT('Ctrl Pts',(-0.220004051678502,-0.770085353509153,
-4.5375182986013));
#70296=CARTESIAN_POINT('Ctrl Pts',(0.401138704855467,-0.628766061699122,
-4.51104063444399));
#70297=CARTESIAN_POINT('Ctrl Pts',(0.660153306932357,-0.243781990912655,
-4.48985850311813));
#70298=CARTESIAN_POINT('Ctrl Pts',(0.713448163538854,0.21944967658462,-4.46867637179228));
#70299=CARTESIAN_POINT('Ctrl Pts',(0.408703467624615,0.624380052697233,
-4.44749424046641));
#70300=CARTESIAN_POINT('Ctrl Pts',(-0.0518139061167167,0.702527732340824,
-4.42631210914056));
#70301=CARTESIAN_POINT('Ctrl Pts',(-0.381729763931295,0.593835130031606,
-4.41042551064616));
#70302=CARTESIAN_POINT('Ctrl Pts',(-0.617941327913625,0.338198834530834,
-4.39453891215177));
#70303=CARTESIAN_POINT('Ctrl Pts',(-0.737373497855252,-0.11206696999172,
-4.37335678082591));
#70304=CARTESIAN_POINT('Ctrl Pts',(-0.435577045604655,-0.671380824354025,
-4.34687911666859));
#70305=CARTESIAN_POINT('Ctrl Pts',(0.33083155171032,-0.729372140157004,
-4.3151059196798));
#70306=CARTESIAN_POINT('Ctrl Pts',(0.712777470420673,-0.219561605337653,
-4.28862825552248));
#70307=CARTESIAN_POINT('Ctrl Pts',(0.660975650409514,0.241543448084987,
-4.26744612419662));
#70308=CARTESIAN_POINT('Ctrl Pts',(0.401722358340205,0.629114925446567,
-4.24626399287076));
#70309=CARTESIAN_POINT('Ctrl Pts',(-0.0926839103114625,0.74047192210371,
-4.2250818615449));
#70310=CARTESIAN_POINT('Ctrl Pts',(-0.494275113109166,0.50191832815303,
-4.20389973021904));
#70311=CARTESIAN_POINT('Ctrl Pts',(-0.675371530643,0.205501994948046,-4.18801313172465));
#70312=CARTESIAN_POINT('Ctrl Pts',(-0.689923040143449,-0.142253770076197,
-4.17212653323026));
#70313=CARTESIAN_POINT('Ctrl Pts',(-0.489472483728134,-0.562756935786156,
-4.1509444019044));
#70314=CARTESIAN_POINT('Ctrl Pts',(0.1026271793844,-0.793692154439977,-4.12446673774708));
#70315=CARTESIAN_POINT('Ctrl Pts',(0.72431759262137,-0.341756140344921,
-4.09269354075829));
#70316=CARTESIAN_POINT('Ctrl Pts',(0.685406179251917,0.294070383277605,
-4.06621587660097));
#70317=CARTESIAN_POINT('Ctrl Pts',(0.347425834209877,0.611986386671006,
-4.0450337452751));
#70318=CARTESIAN_POINT('Ctrl Pts',(-0.10106997904254,0.739561560619801,
-4.02385161394925));
#70319=CARTESIAN_POINT('Ctrl Pts',(-0.549989118149691,0.504381744883291,
-4.00266948262338));
#70320=CARTESIAN_POINT('Ctrl Pts',(-0.701649997804666,0.0625873482081273,
-3.98148735129754));
#70321=CARTESIAN_POINT('Ctrl Pts',(-0.647794192625342,-0.28057166345084,
-3.96560075280313));
#70322=CARTESIAN_POINT('Ctrl Pts',(-0.433764682453468,-0.555047868816476,
-3.94971415430875));
#70323=CARTESIAN_POINT('Ctrl Pts',(-0.00876936604903183,-0.745789366591879,
-3.92853202298289));
#70324=CARTESIAN_POINT('Ctrl Pts',(0.592020032873446,-0.538508917887617,
-3.90205435882556));
#70325=CARTESIAN_POINT('Ctrl Pts',(0.773304882718845,0.208405356954825,
-3.87028116183678));
#70326=CARTESIAN_POINT('Ctrl Pts',(0.332043120165925,0.667837096325308,
-3.84380349767945));
#70327=CARTESIAN_POINT('Ctrl Pts',(-0.13136609001657,0.691357359215059,
-3.82262136635359));
#70328=CARTESIAN_POINT('Ctrl Pts',(-0.555791578009408,0.498259133808778,
-3.80143923502774));
#70329=CARTESIAN_POINT('Ctrl Pts',(-0.745709399577484,0.0283983456625421,
-3.78025710370188));
#70330=CARTESIAN_POINT('Ctrl Pts',(-0.575307256124054,-0.40651132410552,
-3.75907497237602));
#70331=CARTESIAN_POINT('Ctrl Pts',(-0.312114038360918,-0.633200285366913,
-3.74318837388162));
#70332=CARTESIAN_POINT('Ctrl Pts',(0.0287001253000533,-0.703851006413595,
-3.72730177538723));
#70333=CARTESIAN_POINT('Ctrl Pts',(0.476104623192633,-0.574110676504985,
-3.70611964406137));
#70334=CARTESIAN_POINT('Ctrl Pts',(0.79983728491478,-0.0272009490298287,
-3.67964197990405));
#70335=CARTESIAN_POINT('Ctrl Pts',(0.454494167067824,0.659445438641893,
-3.64786878291526));
#70336=CARTESIAN_POINT('Ctrl Pts',(-0.179245745608589,0.723968219992404,
-3.62139111875794));
#70337=CARTESIAN_POINT('Ctrl Pts',(-0.547677888989984,0.441906073344255,
-3.60020898743208));
#70338=CARTESIAN_POINT('Ctrl Pts',(-0.746168494081024,0.0199755112803014,
-3.57902685610622));
#70339=CARTESIAN_POINT('Ctrl Pts',(-0.586756593893505,-0.461091828356436,
-3.55784472478036));
#70340=CARTESIAN_POINT('Ctrl Pts',(-0.175337816586413,-0.682265744156719,
-3.53666259345451));
#70341=CARTESIAN_POINT('Ctrl Pts',(0.172013285242014,-0.684667221379072,
-3.52077599496011));
#70342=CARTESIAN_POINT('Ctrl Pts',(0.477514626316864,-0.517889677513596,
-3.50488939646572));
#70343=CARTESIAN_POINT('Ctrl Pts',(0.734534508884567,-0.129374403805866,
-3.48370726513986));
#70344=CARTESIAN_POINT('Ctrl Pts',(0.627237233394482,0.497044290794701,
-3.45722960098254));
#70345=CARTESIAN_POINT('Ctrl Pts',(-0.0804823222740962,0.796841157474714,
-3.42545640399375));
#70346=CARTESIAN_POINT('Ctrl Pts',(-0.605282042510176,0.43576676088528,
-3.39897873983643));
#70347=CARTESIAN_POINT('Ctrl Pts',(-0.703504024592373,-0.0177238576331333,
-3.37779660851057));
#70348=CARTESIAN_POINT('Ctrl Pts',(-0.581653969262653,-0.467808831309393,
-3.35661447718471));
#70349=CARTESIAN_POINT('Ctrl Pts',(-0.148731575015875,-0.731278259794368,
-3.33543234585885));
#70350=CARTESIAN_POINT('Ctrl Pts',(0.308025509003036,-0.633522044903279,
-3.314250214533));
#70351=CARTESIAN_POINT('Ctrl Pts',(0.5743279309632,-0.410493851410992,-3.2983636160386));
#70352=CARTESIAN_POINT('Ctrl Pts',(0.699214400400128,-0.0856105057499347,
-3.2824770175442));
#70353=CARTESIAN_POINT('Ctrl Pts',(0.643606290730907,0.376894711602609,
-3.26129488621835));
#70354=CARTESIAN_POINT('Ctrl Pts',(0.156311633013567,0.784886136552685,
-3.23481722206102));
#70355=CARTESIAN_POINT('Ctrl Pts',(-0.577179940899014,0.555244585987189,
-3.20304402507224));
#70356=CARTESIAN_POINT('Ctrl Pts',(-0.743435082593453,-0.0596933735603376,
-3.17656636091491));
#70357=CARTESIAN_POINT('Ctrl Pts',(-0.524730724624935,-0.468923996380709,
-3.15538422958906));
#70358=CARTESIAN_POINT('Ctrl Pts',(-0.140494133246507,-0.733094701340396,
-3.1342020982632));
#70359=CARTESIAN_POINT('Ctrl Pts',(0.360032912737676,-0.653655319262541,
-3.11301996693734));
#70360=CARTESIAN_POINT('Ctrl Pts',(0.644886244911881,-0.283463625000574,
-3.09183783561148));
#70361=CARTESIAN_POINT('Ctrl Pts',(0.703481663861427,0.0589179339543426,
-3.07595123711709));
#70362=CARTESIAN_POINT('Ctrl Pts',(0.588354962968238,0.38738659498273,-3.06006463862269));
#70363=CARTESIAN_POINT('Ctrl Pts',(0.246567099391958,0.703905779632369,
-3.03888250729684));
#70364=CARTESIAN_POINT('Ctrl Pts',(-0.388958651052195,0.699421719522368,
-3.01240484313951));
#70365=CARTESIAN_POINT('Ctrl Pts',(-0.799360178391769,0.0495634910569404,
-2.98063164615074));
#70366=CARTESIAN_POINT('Ctrl Pts',(-0.527996742495623,-0.526762243134179,
-2.95415398199339));
#70367=CARTESIAN_POINT('Ctrl Pts',(-0.0963858541361063,-0.697095269579071,
-2.93297185066755));
#70368=CARTESIAN_POINT('Ctrl Pts',(0.367487293040394,-0.649707266439206,
-2.91178971934168));
#70369=CARTESIAN_POINT('Ctrl Pts',(0.697559134358486,-0.265141903002185,
-2.89060758801583));
#70370=CARTESIAN_POINT('Ctrl Pts',(0.675027237917631,0.201415301415524,
-2.86942545668997));
#70371=CARTESIAN_POINT('Ctrl Pts',(0.498046596364184,0.500307267767271,
-2.85353885819557));
#70372=CARTESIAN_POINT('Ctrl Pts',(0.197663098653,0.676135515893496,-2.83765225970118));
#70373=CARTESIAN_POINT('Ctrl Pts',(-0.267743933191193,0.696126330016126,
-2.81647012837532));
#70374=CARTESIAN_POINT('Ctrl Pts',(-0.749233056554967,0.281299486194467,
-2.78999246421801));
#70375=CARTESIAN_POINT('Ctrl Pts',(-0.641350032948401,-0.47969091056778,
-2.75821926722921));
#70376=CARTESIAN_POINT('Ctrl Pts',(-0.0614334537891717,-0.743293314670101,
-2.7317416030719));
#70377=CARTESIAN_POINT('Ctrl Pts',(0.377801898928307,-0.593715228803531,
-2.71055947174603));
#70378=CARTESIAN_POINT('Ctrl Pts',(0.70068501300572,-0.257307122247392,
-2.68937734042018));
#70379=CARTESIAN_POINT('Ctrl Pts',(0.703313419396356,0.249477872268438,
-2.66819520909431));
#70380=CARTESIAN_POINT('Ctrl Pts',(0.384112878137958,0.590497411021916,
-2.64701307776846));
#70381=CARTESIAN_POINT('Ctrl Pts',(0.0557314198619299,0.703741275733401,
-2.63112647927406));
#70382=CARTESIAN_POINT('Ctrl Pts',(-0.287040965920177,0.643301966657401,
-2.61523988077967));
#70383=CARTESIAN_POINT('Ctrl Pts',(-0.654711033413828,0.357256411878932,
-2.59405774945381));
#70384=CARTESIAN_POINT('Ctrl Pts',(-0.753158458967396,-0.270613949481221,
-2.56758008529649));
#70385=CARTESIAN_POINT('Ctrl Pts',(-0.178302031962507,-0.780795504496738,
-2.53580688830771));
#70386=CARTESIAN_POINT('Ctrl Pts',(0.434348713906479,-0.606300433453199,
-2.50932922415038));
#70387=CARTESIAN_POINT('Ctrl Pts',(0.672300129659377,-0.207953320259739,
-2.48814709282452));
#70388=CARTESIAN_POINT('Ctrl Pts',(0.70062407108951,0.257473015323963,-2.46696496149866));
#70389=CARTESIAN_POINT('Ctrl Pts',(0.374558924196536,0.645441389251823,
-2.44578283017281));
#70390=CARTESIAN_POINT('Ctrl Pts',(-0.0894926216029255,0.698728106099681,
-2.42460069884695));
#70391=CARTESIAN_POINT('Ctrl Pts',(-0.413090643562724,0.572463007129391,
-2.40871410035255));
#70392=CARTESIAN_POINT('Ctrl Pts',(-0.635223074932496,0.304502186354999,
-2.39282750185816));
#70393=CARTESIAN_POINT('Ctrl Pts',(-0.730285540866999,-0.151531217585722,
-2.3716453705323));
#70394=CARTESIAN_POINT('Ctrl Pts',(-0.398867864803067,-0.693818420334465,
-2.34516770637498));
#70395=CARTESIAN_POINT('Ctrl Pts',(0.369549690352763,-0.710539415377113,
-2.31339450938619));
#70396=CARTESIAN_POINT('Ctrl Pts',(0.723546655452461,-0.180939929980367,
-2.28691684522887));
#70397=CARTESIAN_POINT('Ctrl Pts',(0.647040070382234,0.276715006941831,
-2.26573471390301));
#70398=CARTESIAN_POINT('Ctrl Pts',(0.36733345238644,0.649794257721565,-2.24455258257715));
#70399=CARTESIAN_POINT('Ctrl Pts',(-0.132342674989519,0.734421126487522,
-2.22337045125129));
#70400=CARTESIAN_POINT('Ctrl Pts',(-0.520533786771069,0.474630880163505,
-2.20218831992543));
#70401=CARTESIAN_POINT('Ctrl Pts',(-0.685439209546698,0.168910817731426,
-2.18630172143104));
#70402=CARTESIAN_POINT('Ctrl Pts',(-0.681281422170332,-0.179124426662695,
-2.17041512293665));
#70403=CARTESIAN_POINT('Ctrl Pts',(-0.458522831705819,-0.588247816746384,
-2.14923299161079));
#70404=CARTESIAN_POINT('Ctrl Pts',(0.145131611989728,-0.787030106901402,
-2.12275532745347));
#70405=CARTESIAN_POINT('Ctrl Pts',(0.741636792304015,-0.302337729609267,
-2.09098213046468));
#70406=CARTESIAN_POINT('Ctrl Pts',(0.668612518062437,0.330478927570208,
-2.06450446630736));
#70407=CARTESIAN_POINT('Ctrl Pts',(0.314035869248326,0.629772594332678,
-2.0433223349815));
#70408=CARTESIAN_POINT('Ctrl Pts',(-0.14066770319757,0.733061416176826,
-2.02214020365564));
#70409=CARTESIAN_POINT('Ctrl Pts',(-0.57629966717217,0.474096686628197,
-2.00095807232978));
#70410=CARTESIAN_POINT('Ctrl Pts',(-0.703999522147564,0.0247904899309355,
-1.97977594100392));
#70411=CARTESIAN_POINT('Ctrl Pts',(-0.631780297798543,-0.314978459016283,
-1.96388934250953));
#70412=CARTESIAN_POINT('Ctrl Pts',(-0.403309811719612,-0.577556172326435,
-1.94800274401514));
#70413=CARTESIAN_POINT('Ctrl Pts',(0.0313217580437868,-0.745182949734803,
-1.92682061268927));
#70414=CARTESIAN_POINT('Ctrl Pts',(0.620103828443481,-0.505915819003228,
-1.90034294853195));
#70415=CARTESIAN_POINT('Ctrl Pts',(0.760987813965571,0.249661333490343,
-1.86856975154317));
#70416=CARTESIAN_POINT('Ctrl Pts',(0.295673986471208,0.684715937160779,
-1.84209208738584));
#70417=CARTESIAN_POINT('Ctrl Pts',(-0.168329559292972,0.683298768632944,
-1.82090995605999));
#70418=CARTESIAN_POINT('Ctrl Pts',(-0.581764715454044,0.467671100735052,
-1.79972782473413));
#70419=CARTESIAN_POINT('Ctrl Pts',(-0.746157952575386,-0.0117168452704052,
-1.77854569340826));
#70420=CARTESIAN_POINT('Ctrl Pts',(-0.552630154216026,-0.436840712647278,
-1.75736356208241));
#70421=CARTESIAN_POINT('Ctrl Pts',(-0.277635072315359,-0.649058195350113,
-1.74147696358801));
#70422=CARTESIAN_POINT('Ctrl Pts',(0.0664833528996994,-0.701291594280784,
-1.72559036509362));
#70423=CARTESIAN_POINT('Ctrl Pts',(0.506269144371473,-0.54769538482608,
-1.70440823376776));
#70424=CARTESIAN_POINT('Ctrl Pts',(0.800143274452744,0.0158213247235393,
-1.67793056961044));
#70425=CARTESIAN_POINT('Ctrl Pts',(0.418399054009061,0.682916880775836,
-1.64615737262165));
#70426=CARTESIAN_POINT('Ctrl Pts',(-0.217892523820332,0.713289470650559,
-1.61967970846433));
#70427=CARTESIAN_POINT('Ctrl Pts',(-0.570634357674029,0.411835498213804,
-1.59849757713847));
#70428=CARTESIAN_POINT('Ctrl Pts',(-0.746163743590037,-0.0201521800745495,
-1.57731544581261));
#70429=CARTESIAN_POINT('Ctrl Pts',(-0.561129810822313,-0.49195763035154,
-1.55613331448675));
#70430=CARTESIAN_POINT('Ctrl Pts',(-0.138419734612189,-0.690702448703422,
-1.5349511831609));
#70431=CARTESIAN_POINT('Ctrl Pts',(0.208558492969346,-0.674433932524933,
-1.5190645846665));
#70432=CARTESIAN_POINT('Ctrl Pts',(0.504655813759805,-0.491479853157888,
-1.50317798617211));
#70433=CARTESIAN_POINT('Ctrl Pts',(0.740425626835783,-0.0897138352053628,
-1.48199585484625));
#70434=CARTESIAN_POINT('Ctrl Pts',(0.599619882655918,0.530033555816679,
-1.45551819068893));
#70435=CARTESIAN_POINT('Ctrl Pts',(-0.123187980897615,0.79136461622102,
-1.42374499370014));
#70436=CARTESIAN_POINT('Ctrl Pts',(-0.627825347684238,0.402609430692957,
-1.39726732954282));
#70437=CARTESIAN_POINT('Ctrl Pts',(-0.701534974529444,-0.055504299464422,
-1.37608519821696));
#70438=CARTESIAN_POINT('Ctrl Pts',(-0.555673590256809,-0.498390713899415,
-1.3549030668911));
#70439=CARTESIAN_POINT('Ctrl Pts',(-0.109218024599217,-0.738214330501128,
-1.33372093556524));
#70440=CARTESIAN_POINT('Ctrl Pts',(0.341625653170807,-0.616053413812982,
-1.31253880423938));
#70441=CARTESIAN_POINT('Ctrl Pts',(0.595557808340173,-0.37903650385649,
-1.29665220574499));
#70442=CARTESIAN_POINT('Ctrl Pts',(0.702804700428006,-0.0479112667122281,
-1.2807656072506));
#70443=CARTESIAN_POINT('Ctrl Pts',(0.622422081552932,0.410937262240509,
-1.25958347592474));
#70444=CARTESIAN_POINT('Ctrl Pts',(0.113906261266067,0.792152092474895,
-1.23310581176742));
#70445=CARTESIAN_POINT('Ctrl Pts',(-0.606184549458043,0.523424804955423,
-1.20133261477863));
#70446=CARTESIAN_POINT('Ctrl Pts',(-0.739152904729264,-0.099559049352841,
-1.17485495062131));
#70447=CARTESIAN_POINT('Ctrl Pts',(-0.498772672191106,-0.496445232852937,
-1.15367281929545));
#70448=CARTESIAN_POINT('Ctrl Pts',(-0.100894871170555,-0.739585470098981,
-1.13249068796959));
#70449=CARTESIAN_POINT('Ctrl Pts',(0.394639860164164,-0.633362736055885,
-1.11130855664373));
#70450=CARTESIAN_POINT('Ctrl Pts',(0.659187605562879,-0.248398060071516,
-1.09012642531787));
#70451=CARTESIAN_POINT('Ctrl Pts',(0.699298891271897,0.0966376479255593,
-1.07423982682348));
#70452=CARTESIAN_POINT('Ctrl Pts',(0.566686762943658,0.418444798182639,
-1.05835322832909));
#70453=CARTESIAN_POINT('Ctrl Pts',(0.208383162066687,0.716139049954344,
-1.03717109700323));
#70454=CARTESIAN_POINT('Ctrl Pts',(-0.425983270133073,0.677508544252163,
-1.0106934328459));
#70455=CARTESIAN_POINT('Ctrl Pts',(-0.800868612319126,0.00653454254947985,
-0.978920235857118));
#70456=CARTESIAN_POINT('Ctrl Pts',(-0.498925764037445,-0.554375416894904,
-0.952442571699792));
#70457=CARTESIAN_POINT('Ctrl Pts',(-0.0587849258484244,-0.701267695135047,
-0.931260440373935));
#70458=CARTESIAN_POINT('Ctrl Pts',(0.401871301811429,-0.629019792526908,
-0.910078309048076));
#70459=CARTESIAN_POINT('Ctrl Pts',(0.710799778962247,-0.227272191175134,
-0.888896177722219));
#70460=CARTESIAN_POINT('Ctrl Pts',(0.663227825248934,0.237399973442935,
-0.867714046396359));
#70461=CARTESIAN_POINT('Ctrl Pts',(0.470440577277662,0.526349159381354,
-0.851827447901968));
#70462=CARTESIAN_POINT('Ctrl Pts',(0.16104219249472,0.685780831357495,-0.83594084940757));
#70463=CARTESIAN_POINT('Ctrl Pts',(-0.304766616737118,0.680731951966365,
-0.814758718081714));
#70464=CARTESIAN_POINT('Ctrl Pts',(-0.763267334089122,0.240629488373161,
-0.788281053924392));
#70465=CARTESIAN_POINT('Ctrl Pts',(-0.614644853367136,-0.513463668309351,
-0.756507856935603));
#70466=CARTESIAN_POINT('Ctrl Pts',(-0.0214003660392715,-0.745520653788183,
-0.730030192778282));
#70467=CARTESIAN_POINT('Ctrl Pts',(0.409162010937815,-0.572554361200174,
-0.708848061452424));
#70468=CARTESIAN_POINT('Ctrl Pts',(0.713500102386157,-0.219280748262106,
-0.687665930126567));
#70469=CARTESIAN_POINT('Ctrl Pts',(0.688890267353093,0.286913182271502,
-0.666483798800706));
#70470=CARTESIAN_POINT('Ctrl Pts',(0.351824709607146,0.610286219109459,
-0.64530166747485));
#70471=CARTESIAN_POINT('Ctrl Pts',(0.0178320838607445,0.70571934318682,
-0.629415068980454));
#70472=CARTESIAN_POINT('Ctrl Pts',(-0.321197002354292,0.626946904886804,
-0.613528470486061));
#70473=CARTESIAN_POINT('Ctrl Pts',(-0.672963795444224,0.321556235071336,
-0.592346339160204));
#70474=CARTESIAN_POINT('Ctrl Pts',(-0.737527433618484,-0.310697373257205,
-0.56586867500288));
#70475=CARTESIAN_POINT('Ctrl Pts',(-0.136084714826095,-0.789249125190363,
-0.534095478014092));
#70476=CARTESIAN_POINT('Ctrl Pts',(0.466303442539805,-0.582082578534946,
-0.50761781385677));
#70477=CARTESIAN_POINT('Ctrl Pts',(0.682503975557423,-0.171523651470232,
-0.486435682530911));
#70478=CARTESIAN_POINT('Ctrl Pts',(0.685775160935683,0.294752233755149,
-0.465253551205053));
#70479=CARTESIAN_POINT('Ctrl Pts',(0.339331867652397,0.664637404300089,
-0.444071419879196));
#70480=CARTESIAN_POINT('Ctrl Pts',(-0.126912670487204,0.692909095187001,
-0.422889288553336));
#70481=CARTESIAN_POINT('Ctrl Pts',(-0.443257737571659,0.549436516930662,
-0.407002690058943));
#70482=CARTESIAN_POINT('Ctrl Pts',(-0.650668891360673,0.269925384308696,
-0.391116091564549));
#70483=CARTESIAN_POINT('Ctrl Pts',(-0.721087274494807,-0.190557250697438,
-0.36993396023869));
#70484=CARTESIAN_POINT('Ctrl Pts',(-0.361005438736672,-0.714251442192837,
-0.343456296081368));
#70485=CARTESIAN_POINT('Ctrl Pts',(0.407198939161548,-0.689652180392618,
-0.311683099092581));
#70486=CARTESIAN_POINT('Ctrl Pts',(0.732226235701414,-0.141797050653159,
-0.285205434935257));
#70487=CARTESIAN_POINT('Ctrl Pts',(0.631232561002846,0.311089138051407,
-0.264023303609399));
#70488=CARTESIAN_POINT('Ctrl Pts',(0.331887985278457,0.668589766575936,
-0.242841172283542));
#70489=CARTESIAN_POINT('Ctrl Pts',(-0.17162922483904,0.726259811006413,
-0.221659040957683));
#70490=CARTESIAN_POINT('Ctrl Pts',(-0.545275419699615,0.445956922224332,
-0.200476909631823));
#70491=CARTESIAN_POINT('Ctrl Pts',(-0.69355232685328,0.131862298003188,
-0.184590311137431));
#70492=CARTESIAN_POINT('Ctrl Pts',(-0.670622753288826,-0.215533614975662,
-0.168703712643036));
#70493=CARTESIAN_POINT('Ctrl Pts',(-0.426352009365769,-0.611917192034414,
-0.147521581317179));
#70494=CARTESIAN_POINT('Ctrl Pts',(0.187431739085884,-0.778344785456901,
-0.121043917159855));
#70495=CARTESIAN_POINT('Ctrl Pts',(0.756436645482091,-0.261606416380455,
-0.0892707201710683));
#70496=CARTESIAN_POINT('Ctrl Pts',(0.650518462326474,0.365194457230119,
-0.0627930560137451));
#70497=CARTESIAN_POINT('Ctrl Pts',(0.278887226280858,0.64673161704124,-0.0416109246878868));
#70498=CARTESIAN_POINT('Ctrl Pts',(-0.0633939700665578,0.702956002425801,
-0.0257243261934916));
#70499=CARTESIAN_POINT('Ctrl Pts',(-0.392875925177587,0.585943088661304,
-0.00983772769910082));
#70500=CARTESIAN_POINT('Ctrl Pts',(-0.54753912821223,0.413276816066991,
0.000753337963830376));
#70501=CARTESIAN_POINT('Ctrl Pts',(-0.599695759644924,0.3135089884898,0.00604887079529526));
#70502=CARTESIAN_POINT('Origin',(0.,0.,-0.0599999999999996));
#70503=CARTESIAN_POINT('',(0.8511,-1.04229689075431E-16,0.));
#70504=CARTESIAN_POINT('Origin',(0.,0.,0.));
#70505=CARTESIAN_POINT('Origin',(0.8511,-1.04229689075431E-16,-0.0599999999999996));
#70506=CARTESIAN_POINT('Origin',(0.,0.,-0.0599999999999996));
#70507=CARTESIAN_POINT('Origin',(0.,0.,0.));
#70508=CARTESIAN_POINT('',(1.2,-0.692820323027552,0.));
#70509=CARTESIAN_POINT('',(1.2,0.692820323027551,0.));
#70510=CARTESIAN_POINT('',(1.2,-0.692820323027552,0.));
#70511=CARTESIAN_POINT('',(-2.54538057293978E-16,-1.3856406460551,0.));
#70512=CARTESIAN_POINT('',(-2.54538057293978E-16,-1.3856406460551,0.));
#70513=CARTESIAN_POINT('',(-1.2,-0.692820323027551,0.));
#70514=CARTESIAN_POINT('',(-1.2,-0.692820323027551,0.));
#70515=CARTESIAN_POINT('',(-1.2,0.692820323027551,0.));
#70516=CARTESIAN_POINT('',(-1.2,0.692820323027551,0.));
#70517=CARTESIAN_POINT('',(8.48460190979926E-17,1.3856406460551,0.));
#70518=CARTESIAN_POINT('',(8.48460190979926E-17,1.3856406460551,0.));
#70519=CARTESIAN_POINT('',(1.2,0.692820323027551,0.));
#70520=CARTESIAN_POINT('Origin',(0.,0.,-5.925));
#70521=CARTESIAN_POINT('Origin',(0.,0.,0.914655896708346));
#70522=CARTESIAN_POINT('',(1.2,-0.692820323027552,0.858179306876173));
#70523=CARTESIAN_POINT('',(-2.54538057293978E-16,-1.3856406460551,0.858179306876173));
#70524=CARTESIAN_POINT('Ctrl Pts',(1.2,-0.692820323027552,0.858179306876173));
#70525=CARTESIAN_POINT('Ctrl Pts',(0.599999999999999,-1.03923048454133,
1.05817930687617));
#70526=CARTESIAN_POINT('Ctrl Pts',(-2.54538057293978E-16,-1.3856406460551,
0.858179306876173));
#70527=CARTESIAN_POINT('',(1.2,0.692820323027551,0.858179306876173));
#70528=CARTESIAN_POINT('Ctrl Pts',(1.2,0.692820323027551,0.858179306876173));
#70529=CARTESIAN_POINT('Ctrl Pts',(1.2,-6.66133814775094E-16,1.05817930687617));
#70530=CARTESIAN_POINT('Ctrl Pts',(1.2,-0.692820323027552,0.858179306876173));
#70531=CARTESIAN_POINT('',(8.48460190979925E-17,1.3856406460551,0.858179306876173));
#70532=CARTESIAN_POINT('Ctrl Pts',(8.48460190979925E-17,1.3856406460551,
0.858179306876173));
#70533=CARTESIAN_POINT('Ctrl Pts',(0.6,1.03923048454133,1.05817930687617));
#70534=CARTESIAN_POINT('Ctrl Pts',(1.2,0.692820323027551,0.858179306876173));
#70535=CARTESIAN_POINT('',(-1.2,0.692820323027551,0.858179306876173));
#70536=CARTESIAN_POINT('Ctrl Pts',(-1.2,0.692820323027551,0.858179306876173));
#70537=CARTESIAN_POINT('Ctrl Pts',(-0.600000000000001,1.03923048454133,
1.05817930687617));
#70538=CARTESIAN_POINT('Ctrl Pts',(8.48460190979925E-17,1.3856406460551,
0.858179306876173));
#70539=CARTESIAN_POINT('',(-1.2,-1.11389921653139E-16,0.965358983848622));
#70540=CARTESIAN_POINT('Ctrl Pts',(-1.2,-7.58222274085957E-17,0.965358983848622));
#70541=CARTESIAN_POINT('Ctrl Pts',(-1.2,0.321539030917347,0.965358983848622));
#70542=CARTESIAN_POINT('Ctrl Pts',(-1.2,0.692820323027551,0.858179306876173));
#70543=CARTESIAN_POINT('',(-1.14,-1.39609735102798E-16,1.));
#70544=CARTESIAN_POINT('',(-1.28782032302755,-1.5771250364726E-16,0.914655896708346));
#70545=CARTESIAN_POINT('Origin',(0.,0.,1.));
#70546=CARTESIAN_POINT('',(-1.2,-0.692820323027551,0.858179306876173));
#70547=CARTESIAN_POINT('Ctrl Pts',(-1.2,-0.692820323027551,0.858179306876173));
#70548=CARTESIAN_POINT('Ctrl Pts',(-1.2,-0.321539030917347,0.965358983848622));
#70549=CARTESIAN_POINT('Ctrl Pts',(-1.2,-7.58222274085957E-17,0.965358983848622));
#70550=CARTESIAN_POINT('Ctrl Pts',(-2.54538057293978E-16,-1.3856406460551,
0.858179306876173));
#70551=CARTESIAN_POINT('Ctrl Pts',(-0.599999999999999,-1.03923048454133,
1.05817930687617));
#70552=CARTESIAN_POINT('Ctrl Pts',(-1.2,-0.692820323027551,0.858179306876173));
#70553=CARTESIAN_POINT('Origin',(8.48460190979926E-17,1.3856406460551,0.));
#70554=CARTESIAN_POINT('',(8.48460190979926E-17,1.3856406460551,0.));
#70555=CARTESIAN_POINT('',(-1.2,0.692820323027551,0.));
#70556=CARTESIAN_POINT('Origin',(1.2,0.692820323027551,0.));
#70557=CARTESIAN_POINT('',(1.2,0.692820323027551,0.));
#70558=CARTESIAN_POINT('Origin',(1.2,-0.692820323027552,0.));
#70559=CARTESIAN_POINT('',(1.2,-0.692820323027552,0.));
#70560=CARTESIAN_POINT('Origin',(-2.54538057293978E-16,-1.3856406460551,
0.));
#70561=CARTESIAN_POINT('',(-2.54538057293978E-16,-1.3856406460551,0.));
#70562=CARTESIAN_POINT('Origin',(-1.2,-0.692820323027551,0.));
#70563=CARTESIAN_POINT('',(-1.2,-0.692820323027551,0.));
#70564=CARTESIAN_POINT('Origin',(-1.2,0.692820323027551,0.));
#70565=CARTESIAN_POINT('Origin',(0.,0.,1.));
#70566=CARTESIAN_POINT('Origin',(0.7,0.,-12.));
#70567=CARTESIAN_POINT('',(-0.7,-8.57252759403147E-17,-12.));
#70568=CARTESIAN_POINT('Origin',(0.,0.,-12.));
#70569=CARTESIAN_POINT('Origin',(0.,0.,-11.95));
#70570=CARTESIAN_POINT('',(-0.75,-9.18485099360515E-17,-11.95));
#71466=UNCERTAINTY_MEASURE_WITH_UNIT(LENGTH_MEASURE(0.001),#71493,
'DISTANCE_ACCURACY_VALUE',
'Maximum model space distance between geometric entities at asserted c
onnectivities');
#71471=UNCERTAINTY_MEASURE_WITH_UNIT(LENGTH_MEASURE(0.001),#71493,
'DISTANCE_ACCURACY_VALUE',
'Maximum model space distance between geometric entities at asserted c
onnectivities');
#71487=(
GEOMETRIC_REPRESENTATION_CONTEXT(3)
GLOBAL_UNCERTAINTY_ASSIGNED_CONTEXT((#71466))
GLOBAL_UNIT_ASSIGNED_CONTEXT((#71493,#71495,#71496))
REPRESENTATION_CONTEXT('','3D')
);
#71492=(
GEOMETRIC_REPRESENTATION_CONTEXT(3)
GLOBAL_UNCERTAINTY_ASSIGNED_CONTEXT((#71471))
GLOBAL_UNIT_ASSIGNED_CONTEXT((#71493,#71495,#71496))
REPRESENTATION_CONTEXT('','3D')
);
#71493=(
LENGTH_UNIT()
NAMED_UNIT(*)
SI_UNIT(.CENTI.,.METRE.)
);
#71495=(
NAMED_UNIT(*)
PLANE_ANGLE_UNIT()
SI_UNIT($,.RADIAN.)
);
#71496=(
NAMED_UNIT(*)
SI_UNIT($,.STERADIAN.)
SOLID_ANGLE_UNIT()
);
#71512=SHAPE_DEFINITION_REPRESENTATION(#71532,#71617);
#71532=PRODUCT_DEFINITION_SHAPE('',$,#71638);
#71617=SHAPE_REPRESENTATION('',(#30284),#71487);
#71622=PRODUCT_DEFINITION_CONTEXT('part definition',#71684,'design');
#71638=PRODUCT_DEFINITION('2026-10-19-03-23-11-739',
'17_ISO_4017_M16x120-8.8',#71658,#71622);
#71658=PRODUCT_DEFINITION_FORMATION('',$,#71701);
#71684=APPLICATION_CONTEXT(
'Core Data for Automotive Mechanical Design Process');
#71685=PRODUCT_CONTEXT('part definition',#71684,'mechanical');
#71701=PRODUCT('2026-10-19-03-23-11-739','17_ISO_4017_M16x120-8.8',$,(#71685));
#71888=COLOUR_RGB('Black',0.12,0.14,0.17);
#71889=FILL_AREA_STYLE_COLOUR('',#71888);
#71890=FILL_AREA_STYLE('',(#71889));
#71891=SURFACE_STYLE_FILL_AREA(#71890);
#71892=SURFACE_SIDE_STYLE('',(#71891));
#71893=SURFACE_STYLE_USAGE(.BOTH.,#71892);
#71894=PRESENTATION_STYLE_ASSIGNMENT((#71893));
ENDSEC;
END-ISO-10303-21;
